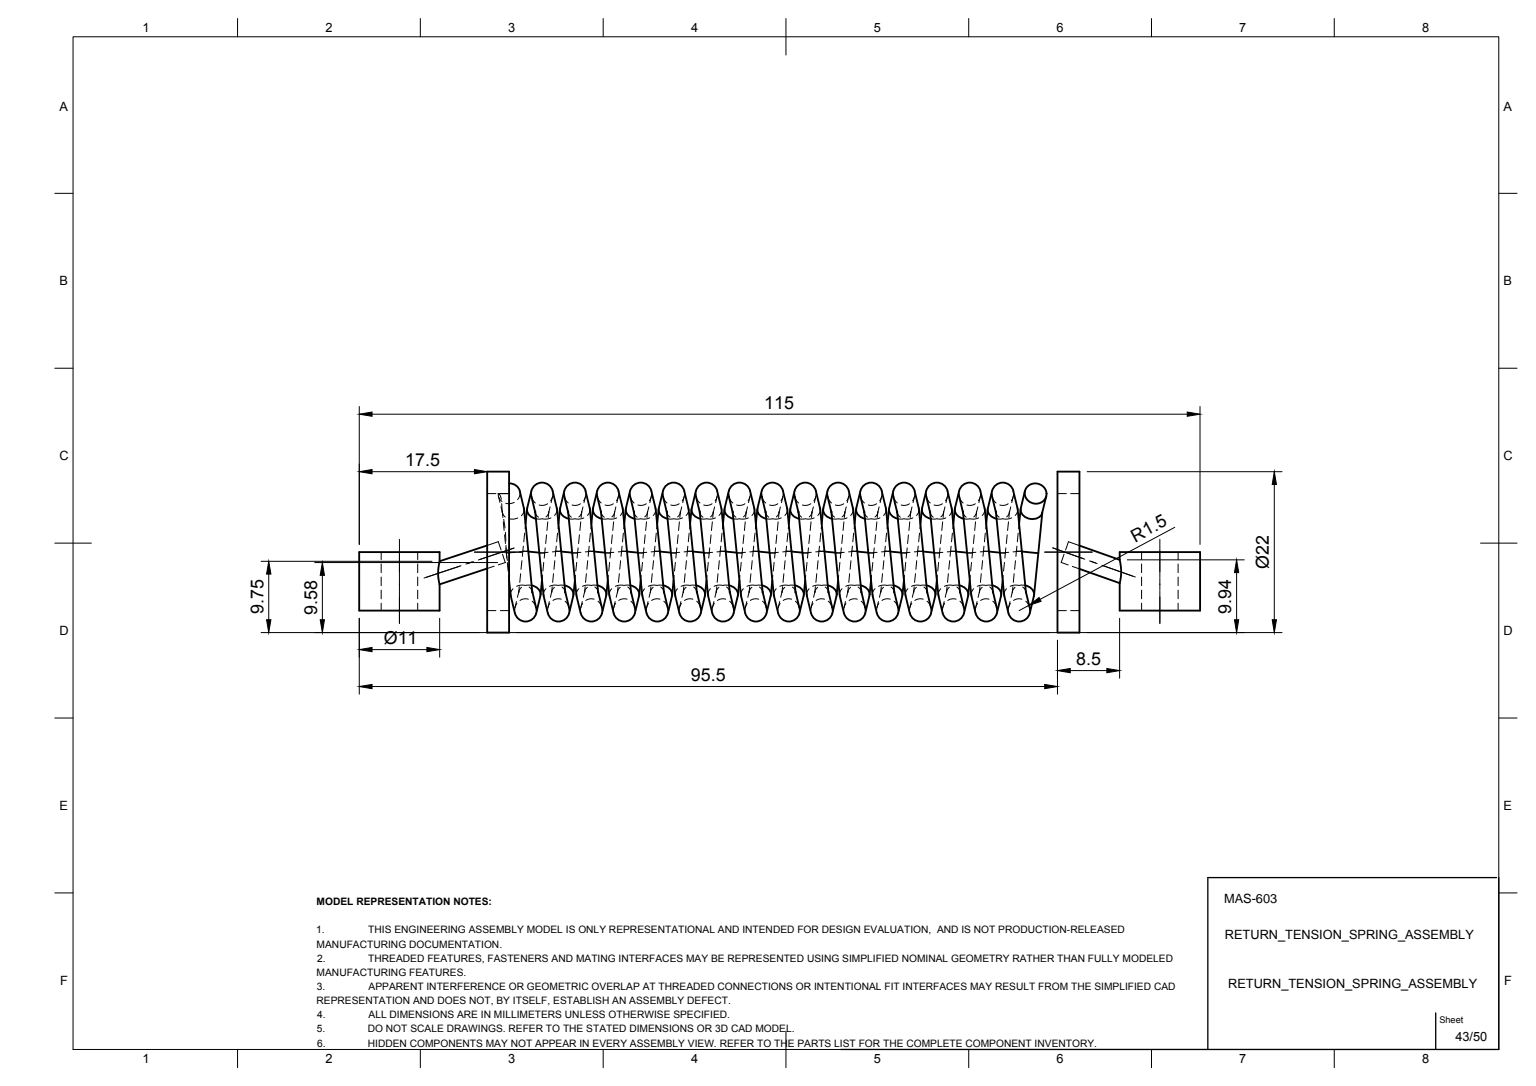
ISO-10303-21;
HEADER;
FILE_DESCRIPTION((''),'2;1');
FILE_NAME('RETURN_TENSION_SPRING_ASSEMBLY.step','2026-10-01T22:06:14-07:00',(''),(''),'','','');
FILE_SCHEMA (('AUTOMOTIVE_DESIGN { 1 0 10303 214 3 1 1 }'));
ENDSEC;
DATA;
#10=MECHANICAL_DESIGN_GEOMETRIC_PRESENTATION_REPRESENTATION('',(#1017,#1018,#1019,#1020),#50440);
#28=B_SPLINE_CURVE_WITH_KNOTS('',3,(#47529,#47530,#47531,#47532,#47533,
#47534,#47535,#47536,#47537,#47538),.UNSPECIFIED.,.F.,.F.,(4,2,2,2,4),(0.,
0.0609860967122279,0.121972193424456,0.180509993590844,0.239047793757233),
 .UNSPECIFIED.) ;
#29=B_SPLINE_CURVE_WITH_KNOTS('',3,(#47539,#47540,#47541,#47542,#47543,
#47544,#47545,#47546,#47547,#47548,#47549,#47550,#47551,#47552,#47553,#47554,
#47555,#47556,#47557,#47558,#47559,#47560,#47561,#47562,#47563,#47564),
 .UNSPECIFIED.,.F.,.F.,(4,2,2,2,2,2,2,2,2,2,2,2,4),(0.239047793757233,0.297585593923622,
0.35612339409001,0.417109490802238,0.478095587514466,0.536342851072485,
0.594590114630504,0.651016946753083,0.707443778875663,0.763870610998243,
0.820297443120823,0.878544706678841,0.93679197023686),.UNSPECIFIED.) ;
#30=B_SPLINE_CURVE_WITH_KNOTS('',3,(#47597,#47598,#47599,#47600,#47601,
#47602,#47603,#47604,#47605,#47606),.UNSPECIFIED.,.F.,.F.,(4,2,2,2,4),(1.59601342827562,
1.72868455666642,1.90688135822923,2.08609099459942,2.19153831493185),
 .UNSPECIFIED.) ;
#31=B_SPLINE_CURVE_WITH_KNOTS('',3,(#47608,#47609,#47610,#47611,#47612,
#47613,#47614,#47615,#47616,#47617),.UNSPECIFIED.,.F.,.F.,(4,2,2,2,4),(1.59601342827561,
1.72868455666641,1.90688135822922,2.0860909945994,2.19148469566779),
 .UNSPECIFIED.) ;
#32=B_SPLINE_CURVE_WITH_KNOTS('',3,(#47619,#47620,#47621,#47622,#47623,
#47624),.UNSPECIFIED.,.F.,.F.,(4,2,4),(1.93627902173741,2.08609099459941,
2.19148469566782),.UNSPECIFIED.) ;
#33=B_SPLINE_CURVE_WITH_KNOTS('',3,(#49299,#49300,#49301,#49302,#49303,
#49304,#49305,#49306,#49307,#49308,#49309,#49310,#49311,#49312,#49313,#49314,
#49315,#49316),.UNSPECIFIED.,.F.,.F.,(4,2,2,2,2,2,2,2,4),(0.228893413219578,
0.285350813018225,0.341808212816873,0.399797519628014,0.457786826439155,
0.518403668051846,0.579020509664538,0.637418929805441,0.695817349946344),
 .UNSPECIFIED.) ;
#34=B_SPLINE_CURVE_WITH_KNOTS('',3,(#49321,#49322,#49323,#49324,#49325,
#49326,#49327,#49328,#49329,#49330),.UNSPECIFIED.,.F.,.F.,(4,2,2,2,4),(0.,
0.0579893068111412,0.115978613622282,0.17243601342093,0.228893413219578),
 .UNSPECIFIED.) ;
#35=B_SPLINE_CURVE_WITH_KNOTS('',3,(#49331,#49332,#49333,#49334,#49335,
#49336,#49337,#49338,#49339,#49340),.UNSPECIFIED.,.F.,.F.,(4,2,2,2,4),(0.695817349946344,
0.754215770087248,0.812614190228152,0.873231031840842,0.933847873453534),
 .UNSPECIFIED.) ;
#417=ELLIPSE('',#31090,8.74484398085574,0.8) ;
#418=ELLIPSE('',#31097,1.63965824641058,0.15) ;
#419=ELLIPSE('',#31099,1.63965824641055,0.15) ;
#420=ELLIPSE('',#31101,1.63965824641045,0.15) ;
#421=ELLIPSE('',#31675,0.162242389830004,0.15) ;
#422=ELLIPSE('',#31677,0.162242389830007,0.15) ;
#423=ELLIPSE('',#31679,0.162242389830008,0.15) ;
#424=ELLIPSE('',#31680,0.162242389830008,0.15) ;
#425=ELLIPSE('',#31682,0.16224238983001,0.15) ;
#426=ELLIPSE('',#31683,0.16224238983001,0.15) ;
#427=ELLIPSE('',#31685,0.162242389830005,0.15) ;
#428=ELLIPSE('',#31686,0.162242389830005,0.15) ;
#429=ELLIPSE('',#31688,0.162242389830007,0.15) ;
#430=ELLIPSE('',#31689,0.162242389830007,0.15) ;
#431=ELLIPSE('',#31691,0.162242389830009,0.15) ;
#432=ELLIPSE('',#31692,0.162242389830009,0.15) ;
#433=ELLIPSE('',#31694,0.162242389830009,0.15) ;
#434=ELLIPSE('',#31695,0.162242389830009,0.15) ;
#435=ELLIPSE('',#31697,0.162242389830006,0.15) ;
#436=ELLIPSE('',#31698,0.162242389830006,0.15) ;
#437=ELLIPSE('',#31700,0.16224238983001,0.15) ;
#438=ELLIPSE('',#31701,0.16224238983001,0.15) ;
#439=ELLIPSE('',#31703,0.162242389830006,0.15) ;
#440=ELLIPSE('',#31704,0.162242389830006,0.15) ;
#441=ELLIPSE('',#31706,0.162242389830011,0.15) ;
#442=ELLIPSE('',#31707,0.162242389830011,0.15) ;
#443=ELLIPSE('',#31709,0.162242389830005,0.15) ;
#444=ELLIPSE('',#31710,0.162242389830005,0.15) ;
#445=ELLIPSE('',#31712,0.162242389830007,0.15) ;
#446=ELLIPSE('',#31713,0.162242389830007,0.15) ;
#447=ELLIPSE('',#31715,0.162242389830006,0.15) ;
#448=ELLIPSE('',#31716,0.162242389830006,0.15) ;
#449=ELLIPSE('',#31718,0.162242389830011,0.15) ;
#450=ELLIPSE('',#31719,0.162242389830011,0.15) ;
#451=ELLIPSE('',#31721,0.162242389830004,0.15) ;
#452=ELLIPSE('',#31722,0.162242389830004,0.15) ;
#453=ELLIPSE('',#31724,0.162242389830007,0.15) ;
#454=ELLIPSE('',#31725,0.162242389830007,0.15) ;
#455=ELLIPSE('',#31727,0.162242389830008,0.15) ;
#456=ELLIPSE('',#31728,0.162242389830008,0.15) ;
#457=ELLIPSE('',#31730,0.162242389830011,0.15) ;
#458=ELLIPSE('',#31731,0.162242389830011,0.15) ;
#459=ELLIPSE('',#31733,0.162242389830005,0.15) ;
#460=ELLIPSE('',#31734,0.162242389830005,0.15) ;
#461=ELLIPSE('',#31736,0.162242389830007,0.15) ;
#462=ELLIPSE('',#31737,0.162242389830007,0.15) ;
#463=ELLIPSE('',#31739,0.162242389830008,0.15) ;
#464=ELLIPSE('',#31740,0.162242389830008,0.15) ;
#465=ELLIPSE('',#31742,0.162242389830008,0.15) ;
#466=ELLIPSE('',#31743,0.162242389830008,0.15) ;
#467=ELLIPSE('',#31745,0.162242389830006,0.15) ;
#468=ELLIPSE('',#31746,0.162242389830006,0.15) ;
#469=ELLIPSE('',#31748,0.16224238983001,0.15) ;
#470=ELLIPSE('',#31749,0.16224238983001,0.15) ;
#471=ELLIPSE('',#31751,0.162242389830006,0.15) ;
#472=ELLIPSE('',#31752,0.162242389830006,0.15) ;
#473=ELLIPSE('',#31754,0.16224238983001,0.15) ;
#474=ELLIPSE('',#31755,0.16224238983001,0.15) ;
#475=ELLIPSE('',#31757,0.162242389830005,0.15) ;
#476=ELLIPSE('',#31758,0.162242389830005,0.15) ;
#477=ELLIPSE('',#31760,0.16224238983001,0.15) ;
#478=ELLIPSE('',#31761,0.16224238983001,0.15) ;
#479=ELLIPSE('',#31763,0.162242389830006,0.15) ;
#480=ELLIPSE('',#31764,0.162242389830006,0.15) ;
#481=ELLIPSE('',#31766,0.162242389830011,0.15) ;
#482=ELLIPSE('',#31767,0.162242389830011,0.15) ;
#483=ELLIPSE('',#31769,0.162242389830004,0.15) ;
#484=ELLIPSE('',#31770,0.162242389830004,0.15) ;
#485=ELLIPSE('',#31772,0.162242389830007,0.15) ;
#486=ELLIPSE('',#31773,0.162242389830007,0.15) ;
#487=ELLIPSE('',#31775,0.162242389830008,0.15) ;
#488=ELLIPSE('',#31776,0.162242389830008,0.15) ;
#489=ELLIPSE('',#31778,0.16224238983001,0.15) ;
#490=ELLIPSE('',#31779,0.16224238983001,0.15) ;
#491=ELLIPSE('',#31781,0.162242389830005,0.15) ;
#492=ELLIPSE('',#31782,0.162242389830005,0.15) ;
#493=ELLIPSE('',#31784,0.162242389830007,0.15) ;
#494=ELLIPSE('',#31785,0.162242389830007,0.15) ;
#495=ELLIPSE('',#31787,0.162242389830009,0.15) ;
#496=ELLIPSE('',#31788,0.162242389830009,0.15) ;
#497=ELLIPSE('',#31790,0.162242389830008,0.15) ;
#498=ELLIPSE('',#31791,0.162242389830008,0.15) ;
#499=ELLIPSE('',#31793,0.162242389830006,0.15) ;
#500=ELLIPSE('',#31794,0.162242389830006,0.15) ;
#501=ELLIPSE('',#31796,0.16224238983001,0.15) ;
#502=ELLIPSE('',#31797,0.16224238983001,0.15) ;
#503=ELLIPSE('',#31799,0.162242389830006,0.15) ;
#504=ELLIPSE('',#31800,0.162242389830006,0.15) ;
#505=ELLIPSE('',#31802,0.16224238983001,0.15) ;
#506=ELLIPSE('',#31803,0.16224238983001,0.15) ;
#507=ELLIPSE('',#31805,0.162242389830005,0.15) ;
#508=ELLIPSE('',#31806,0.162242389830005,0.15) ;
#509=ELLIPSE('',#31808,0.16224238983001,0.15) ;
#510=ELLIPSE('',#31809,0.16224238983001,0.15) ;
#511=ELLIPSE('',#31811,0.162242389830006,0.15) ;
#512=ELLIPSE('',#31812,0.162242389830006,0.15) ;
#513=ELLIPSE('',#31814,0.162242389830011,0.15) ;
#514=ELLIPSE('',#31815,0.162242389830011,0.15) ;
#515=ELLIPSE('',#31817,0.162242389830006,0.15) ;
#516=ELLIPSE('',#31818,0.162242389830006,0.15) ;
#517=ELLIPSE('',#31820,0.16224238983001,0.15) ;
#518=ELLIPSE('',#31821,0.16224238983001,0.15) ;
#519=ELLIPSE('',#31823,0.162242389830006,0.15) ;
#520=ELLIPSE('',#31824,0.162242389830006,0.15) ;
#521=ELLIPSE('',#31826,0.162242389830011,0.15) ;
#522=ELLIPSE('',#31827,0.162242389830011,0.15) ;
#523=ELLIPSE('',#31829,0.162242389830005,0.15) ;
#524=ELLIPSE('',#31830,0.162242389830005,0.15) ;
#525=ELLIPSE('',#31832,0.162242389830007,0.15) ;
#526=ELLIPSE('',#31833,0.162242389830007,0.15) ;
#527=ELLIPSE('',#31835,0.162242389830006,0.15) ;
#528=ELLIPSE('',#31836,0.162242389830006,0.15) ;
#529=ELLIPSE('',#31838,0.162242389830011,0.15) ;
#530=ELLIPSE('',#31839,0.162242389830011,0.15) ;
#531=ELLIPSE('',#31841,0.162242389830006,0.15) ;
#532=ELLIPSE('',#31842,0.162242389830006,0.15) ;
#533=ELLIPSE('',#31844,0.16224238983001,0.15) ;
#534=ELLIPSE('',#31845,0.16224238983001,0.15) ;
#535=ELLIPSE('',#31847,0.162242389830006,0.15) ;
#536=ELLIPSE('',#31848,0.162242389830006,0.15) ;
#537=ELLIPSE('',#31850,0.162242389830011,0.15) ;
#538=ELLIPSE('',#31851,0.162242389830011,0.15) ;
#539=ELLIPSE('',#31853,0.162242389830005,0.15) ;
#540=ELLIPSE('',#31854,0.162242389830005,0.15) ;
#541=ELLIPSE('',#31856,0.162242389830007,0.15) ;
#542=ELLIPSE('',#31857,0.162242389830007,0.15) ;
#543=ELLIPSE('',#31859,0.162242389830006,0.15) ;
#544=ELLIPSE('',#31860,0.162242389830006,0.15) ;
#545=ELLIPSE('',#31862,0.162242389830011,0.15) ;
#546=ELLIPSE('',#31863,0.162242389830011,0.15) ;
#547=ELLIPSE('',#31865,0.162242389830006,0.15) ;
#548=ELLIPSE('',#31866,0.162242389830006,0.15) ;
#549=ELLIPSE('',#31868,0.16224238983001,0.15) ;
#550=ELLIPSE('',#31869,0.16224238983001,0.15) ;
#551=ELLIPSE('',#31871,0.162242389830006,0.15) ;
#552=ELLIPSE('',#31872,0.162242389830006,0.15) ;
#553=ELLIPSE('',#31874,0.162242389830011,0.15) ;
#554=ELLIPSE('',#31875,0.162242389830011,0.15) ;
#555=ELLIPSE('',#31877,0.162242389830005,0.15) ;
#556=ELLIPSE('',#31878,0.162242389830005,0.15) ;
#557=ELLIPSE('',#31880,0.162242389830007,0.15) ;
#558=ELLIPSE('',#31881,0.162242389830007,0.15) ;
#559=ELLIPSE('',#31883,0.162242389830006,0.15) ;
#560=ELLIPSE('',#31884,0.162242389830006,0.15) ;
#561=ELLIPSE('',#31886,0.162242389830011,0.15) ;
#562=ELLIPSE('',#31887,0.162242389830011,0.15) ;
#563=ELLIPSE('',#31889,0.162242389830004,0.15) ;
#564=ELLIPSE('',#31890,0.162242389830004,0.15) ;
#565=ELLIPSE('',#31892,0.162242389830007,0.15) ;
#566=ELLIPSE('',#31893,0.162242389830007,0.15) ;
#567=ELLIPSE('',#31895,0.162242389830006,0.15) ;
#568=ELLIPSE('',#31896,0.162242389830006,0.15) ;
#569=ELLIPSE('',#31898,0.16224238983001,0.15) ;
#570=ELLIPSE('',#31899,0.16224238983001,0.15) ;
#571=ELLIPSE('',#31901,0.162242389830005,0.15) ;
#572=ELLIPSE('',#31902,0.162242389830005,0.15) ;
#573=ELLIPSE('',#31904,0.162242389830007,0.15) ;
#574=ELLIPSE('',#31905,0.162242389830007,0.15) ;
#575=ELLIPSE('',#31907,0.162242389830006,0.15) ;
#576=ELLIPSE('',#31908,0.162242389830006,0.15) ;
#577=ELLIPSE('',#31910,0.162242389830011,0.15) ;
#578=ELLIPSE('',#31911,0.162242389830011,0.15) ;
#579=ELLIPSE('',#31913,0.162242389830004,0.15) ;
#580=ELLIPSE('',#31914,0.162242389830004,0.15) ;
#581=ELLIPSE('',#31916,0.162242389830007,0.15) ;
#582=ELLIPSE('',#31917,0.162242389830007,0.15) ;
#583=ELLIPSE('',#31919,0.162242389830006,0.15) ;
#584=ELLIPSE('',#31920,0.162242389830006,0.15) ;
#585=ELLIPSE('',#31922,0.16224238983001,0.15) ;
#586=ELLIPSE('',#31923,0.16224238983001,0.15) ;
#587=ELLIPSE('',#31925,0.162242389830005,0.15) ;
#588=ELLIPSE('',#31926,0.162242389830005,0.15) ;
#589=ELLIPSE('',#31928,0.162242389830007,0.15) ;
#590=ELLIPSE('',#31929,0.162242389830007,0.15) ;
#591=ELLIPSE('',#31931,0.162242389830006,0.15) ;
#592=ELLIPSE('',#31932,0.162242389830006,0.15) ;
#593=ELLIPSE('',#31934,0.162242389830011,0.15) ;
#594=ELLIPSE('',#31935,0.162242389830011,0.15) ;
#595=ELLIPSE('',#31937,0.162242389830004,0.15) ;
#596=ELLIPSE('',#31938,0.162242389830004,0.15) ;
#597=ELLIPSE('',#31940,0.162242389830007,0.15) ;
#598=ELLIPSE('',#31941,0.162242389830007,0.15) ;
#599=ELLIPSE('',#31943,0.162242389830006,0.15) ;
#600=ELLIPSE('',#31944,0.162242389830006,0.15) ;
#601=ELLIPSE('',#31946,0.162242389830011,0.15) ;
#602=ELLIPSE('',#31947,0.162242389830011,0.15) ;
#603=ELLIPSE('',#31949,0.162242389830005,0.15) ;
#604=ELLIPSE('',#31950,0.162242389830005,0.15) ;
#605=ELLIPSE('',#31952,0.162242389830007,0.15) ;
#606=ELLIPSE('',#31953,0.162242389830007,0.15) ;
#607=ELLIPSE('',#31955,0.162242389830008,0.15) ;
#608=ELLIPSE('',#31956,0.162242389830008,0.15) ;
#609=ELLIPSE('',#31958,0.162242389830011,0.15) ;
#610=ELLIPSE('',#31959,0.162242389830011,0.15) ;
#611=ELLIPSE('',#31961,0.162242389830004,0.15) ;
#612=ELLIPSE('',#31962,0.162242389830004,0.15) ;
#613=ELLIPSE('',#31964,0.162242389830007,0.15) ;
#614=ELLIPSE('',#31965,0.162242389830007,0.15) ;
#615=ELLIPSE('',#31967,0.162242389830006,0.15) ;
#616=ELLIPSE('',#31968,0.162242389830006,0.15) ;
#617=ELLIPSE('',#31970,0.16224238983001,0.15) ;
#618=ELLIPSE('',#31971,0.16224238983001,0.15) ;
#619=ELLIPSE('',#31973,0.162242389830005,0.15) ;
#620=ELLIPSE('',#31974,0.162242389830005,0.15) ;
#621=ELLIPSE('',#31976,0.162242389830007,0.15) ;
#622=ELLIPSE('',#31977,0.162242389830007,0.15) ;
#623=ELLIPSE('',#31979,0.162242389830008,0.15) ;
#624=ELLIPSE('',#31980,0.162242389830008,0.15) ;
#625=ELLIPSE('',#31982,0.162242389830011,0.15) ;
#626=ELLIPSE('',#31983,0.162242389830011,0.15) ;
#627=ELLIPSE('',#31985,0.162242389830004,0.15) ;
#628=ELLIPSE('',#31986,0.162242389830004,0.15) ;
#629=ELLIPSE('',#31988,0.162242389830007,0.15) ;
#630=ELLIPSE('',#31989,0.162242389830007,0.15) ;
#631=ELLIPSE('',#31991,0.162242389830006,0.15) ;
#632=ELLIPSE('',#31992,0.162242389830006,0.15) ;
#633=ELLIPSE('',#31994,0.162242389830011,0.15) ;
#634=ELLIPSE('',#31995,0.162242389830011,0.15) ;
#635=ELLIPSE('',#31997,0.162242389830005,0.15) ;
#636=ELLIPSE('',#31998,0.162242389830005,0.15) ;
#637=ELLIPSE('',#32000,0.162242389830007,0.15) ;
#638=ELLIPSE('',#32001,0.162242389830007,0.15) ;
#639=ELLIPSE('',#32003,0.162242389830008,0.15) ;
#640=ELLIPSE('',#32004,0.162242389830008,0.15) ;
#641=ELLIPSE('',#32006,0.162242389830011,0.15) ;
#642=ELLIPSE('',#32007,0.162242389830011,0.15) ;
#643=ELLIPSE('',#32009,0.162242389830004,0.15) ;
#644=ELLIPSE('',#32010,0.162242389830004,0.15) ;
#645=ELLIPSE('',#32012,0.162242389830007,0.15) ;
#646=ELLIPSE('',#32013,0.162242389830007,0.15) ;
#647=ELLIPSE('',#32015,0.162242389830006,0.15) ;
#648=ELLIPSE('',#32016,0.162242389830006,0.15) ;
#649=ELLIPSE('',#32018,0.16224238983001,0.15) ;
#650=ELLIPSE('',#32019,0.16224238983001,0.15) ;
#651=ELLIPSE('',#32021,0.162242389830005,0.15) ;
#652=ELLIPSE('',#32022,0.162242389830005,0.15) ;
#653=ELLIPSE('',#32024,0.162242389830007,0.15) ;
#654=ELLIPSE('',#32025,0.162242389830007,0.15) ;
#655=ELLIPSE('',#32027,0.162242389830008,0.15) ;
#656=ELLIPSE('',#32028,0.162242389830008,0.15) ;
#657=ELLIPSE('',#32030,0.162242389830012,0.15) ;
#658=ELLIPSE('',#32031,0.162242389830012,0.15) ;
#659=ELLIPSE('',#32033,0.162242389830004,0.15) ;
#660=ELLIPSE('',#32034,0.162242389830004,0.15) ;
#661=ELLIPSE('',#32036,0.162242389830007,0.15) ;
#662=ELLIPSE('',#32037,0.162242389830007,0.15) ;
#663=ELLIPSE('',#32039,0.162242389830006,0.15) ;
#664=ELLIPSE('',#32040,0.162242389830006,0.15) ;
#665=ELLIPSE('',#32042,0.162242389830011,0.15) ;
#666=ELLIPSE('',#32043,0.162242389830011,0.15) ;
#667=ELLIPSE('',#32045,0.162242389830005,0.15) ;
#668=ELLIPSE('',#32046,0.162242389830005,0.15) ;
#669=ELLIPSE('',#32048,0.162242389830007,0.15) ;
#670=ELLIPSE('',#32049,0.162242389830007,0.15) ;
#671=ELLIPSE('',#32051,0.162242389830008,0.15) ;
#672=ELLIPSE('',#32052,0.162242389830008,0.15) ;
#748=SPHERICAL_SURFACE('',#31105,0.15) ;
#749=SPHERICAL_SURFACE('',#31108,0.15) ;
#750=SPHERICAL_SURFACE('',#31112,0.15) ;
#751=SPHERICAL_SURFACE('',#31116,0.15) ;
#752=SPHERICAL_SURFACE('',#31122,0.15) ;
#753=SPHERICAL_SURFACE('',#31126,0.15) ;
#754=SPHERICAL_SURFACE('',#31130,0.15) ;
#755=SPHERICAL_SURFACE('',#31134,0.15) ;
#756=SPHERICAL_SURFACE('',#31140,0.15) ;
#757=SPHERICAL_SURFACE('',#31144,0.15) ;
#758=SPHERICAL_SURFACE('',#31148,0.15) ;
#759=SPHERICAL_SURFACE('',#31152,0.15) ;
#760=SPHERICAL_SURFACE('',#31158,0.15) ;
#761=SPHERICAL_SURFACE('',#31162,0.15) ;
#762=SPHERICAL_SURFACE('',#31166,0.15) ;
#763=SPHERICAL_SURFACE('',#31170,0.15) ;
#764=SPHERICAL_SURFACE('',#31176,0.15) ;
#765=SPHERICAL_SURFACE('',#31180,0.15) ;
#766=SPHERICAL_SURFACE('',#31184,0.15) ;
#767=SPHERICAL_SURFACE('',#31188,0.15) ;
#768=SPHERICAL_SURFACE('',#31194,0.15) ;
#769=SPHERICAL_SURFACE('',#31198,0.15) ;
#770=SPHERICAL_SURFACE('',#31202,0.15) ;
#771=SPHERICAL_SURFACE('',#31206,0.15) ;
#772=SPHERICAL_SURFACE('',#31212,0.15) ;
#773=SPHERICAL_SURFACE('',#31216,0.15) ;
#774=SPHERICAL_SURFACE('',#31220,0.15) ;
#775=SPHERICAL_SURFACE('',#31224,0.15) ;
#776=SPHERICAL_SURFACE('',#31230,0.15) ;
#777=SPHERICAL_SURFACE('',#31234,0.15) ;
#778=SPHERICAL_SURFACE('',#31238,0.15) ;
#779=SPHERICAL_SURFACE('',#31242,0.15) ;
#780=SPHERICAL_SURFACE('',#31248,0.15) ;
#781=SPHERICAL_SURFACE('',#31252,0.15) ;
#782=SPHERICAL_SURFACE('',#31256,0.15) ;
#783=SPHERICAL_SURFACE('',#31260,0.15) ;
#784=SPHERICAL_SURFACE('',#31266,0.15) ;
#785=SPHERICAL_SURFACE('',#31270,0.15) ;
#786=SPHERICAL_SURFACE('',#31274,0.15) ;
#787=SPHERICAL_SURFACE('',#31278,0.15) ;
#788=SPHERICAL_SURFACE('',#31284,0.15) ;
#789=SPHERICAL_SURFACE('',#31288,0.15) ;
#790=SPHERICAL_SURFACE('',#31292,0.15) ;
#791=SPHERICAL_SURFACE('',#31296,0.15) ;
#792=SPHERICAL_SURFACE('',#31302,0.15) ;
#793=SPHERICAL_SURFACE('',#31306,0.15) ;
#794=SPHERICAL_SURFACE('',#31310,0.15) ;
#795=SPHERICAL_SURFACE('',#31314,0.15) ;
#796=SPHERICAL_SURFACE('',#31320,0.15) ;
#797=SPHERICAL_SURFACE('',#31324,0.15) ;
#798=SPHERICAL_SURFACE('',#31328,0.15) ;
#799=SPHERICAL_SURFACE('',#31332,0.15) ;
#800=SPHERICAL_SURFACE('',#31338,0.15) ;
#801=SPHERICAL_SURFACE('',#31342,0.15) ;
#802=SPHERICAL_SURFACE('',#31346,0.15) ;
#803=SPHERICAL_SURFACE('',#31350,0.15) ;
#804=SPHERICAL_SURFACE('',#31356,0.15) ;
#805=SPHERICAL_SURFACE('',#31360,0.15) ;
#806=SPHERICAL_SURFACE('',#31364,0.15) ;
#807=SPHERICAL_SURFACE('',#31368,0.15) ;
#808=SPHERICAL_SURFACE('',#31374,0.15) ;
#809=SPHERICAL_SURFACE('',#31378,0.15) ;
#810=SPHERICAL_SURFACE('',#31382,0.15) ;
#811=SPHERICAL_SURFACE('',#31386,0.15) ;
#812=SPHERICAL_SURFACE('',#31392,0.15) ;
#813=SPHERICAL_SURFACE('',#31396,0.15) ;
#814=SPHERICAL_SURFACE('',#31400,0.15) ;
#815=SPHERICAL_SURFACE('',#31404,0.15) ;
#816=SPHERICAL_SURFACE('',#31410,0.15) ;
#817=SPHERICAL_SURFACE('',#31414,0.15) ;
#818=SPHERICAL_SURFACE('',#31418,0.15) ;
#819=SPHERICAL_SURFACE('',#31422,0.15) ;
#820=SPHERICAL_SURFACE('',#31428,0.15) ;
#821=SPHERICAL_SURFACE('',#31432,0.15) ;
#822=SPHERICAL_SURFACE('',#31436,0.15) ;
#823=SPHERICAL_SURFACE('',#31440,0.15) ;
#824=SPHERICAL_SURFACE('',#31446,0.15) ;
#825=SPHERICAL_SURFACE('',#31450,0.15) ;
#826=SPHERICAL_SURFACE('',#31454,0.15) ;
#827=SPHERICAL_SURFACE('',#31458,0.15) ;
#828=SPHERICAL_SURFACE('',#31464,0.15) ;
#829=SPHERICAL_SURFACE('',#31468,0.15) ;
#830=SPHERICAL_SURFACE('',#31472,0.15) ;
#831=SPHERICAL_SURFACE('',#31476,0.15) ;
#832=SPHERICAL_SURFACE('',#31482,0.15) ;
#833=SPHERICAL_SURFACE('',#31486,0.15) ;
#834=SPHERICAL_SURFACE('',#31490,0.15) ;
#835=SPHERICAL_SURFACE('',#31494,0.15) ;
#836=SPHERICAL_SURFACE('',#31500,0.15) ;
#837=SPHERICAL_SURFACE('',#31504,0.15) ;
#838=SPHERICAL_SURFACE('',#31508,0.15) ;
#839=SPHERICAL_SURFACE('',#31512,0.15) ;
#840=SPHERICAL_SURFACE('',#31518,0.15) ;
#841=SPHERICAL_SURFACE('',#31522,0.15) ;
#842=SPHERICAL_SURFACE('',#31526,0.15) ;
#843=SPHERICAL_SURFACE('',#31530,0.15) ;
#844=SPHERICAL_SURFACE('',#31536,0.15) ;
#845=SPHERICAL_SURFACE('',#31540,0.15) ;
#846=SPHERICAL_SURFACE('',#31544,0.15) ;
#847=SPHERICAL_SURFACE('',#31548,0.15) ;
#848=SPHERICAL_SURFACE('',#31554,0.15) ;
#849=SPHERICAL_SURFACE('',#31558,0.15) ;
#850=SPHERICAL_SURFACE('',#31562,0.15) ;
#851=SPHERICAL_SURFACE('',#31566,0.15) ;
#852=SPHERICAL_SURFACE('',#31572,0.15) ;
#853=SPHERICAL_SURFACE('',#31576,0.15) ;
#854=SPHERICAL_SURFACE('',#31580,0.15) ;
#855=SPHERICAL_SURFACE('',#31584,0.15) ;
#856=SPHERICAL_SURFACE('',#31590,0.15) ;
#857=SPHERICAL_SURFACE('',#31594,0.15) ;
#858=SPHERICAL_SURFACE('',#31598,0.15) ;
#859=SPHERICAL_SURFACE('',#31602,0.15) ;
#860=SPHERICAL_SURFACE('',#31608,0.15) ;
#861=SPHERICAL_SURFACE('',#31612,0.15) ;
#862=SPHERICAL_SURFACE('',#31616,0.15) ;
#863=SPHERICAL_SURFACE('',#31620,0.15) ;
#864=SPHERICAL_SURFACE('',#31626,0.15) ;
#865=SPHERICAL_SURFACE('',#31630,0.15) ;
#866=SPHERICAL_SURFACE('',#31634,0.15) ;
#867=SPHERICAL_SURFACE('',#31638,0.15) ;
#868=SPHERICAL_SURFACE('',#31644,0.15) ;
#869=SPHERICAL_SURFACE('',#31648,0.15) ;
#870=SPHERICAL_SURFACE('',#31652,0.15) ;
#871=SPHERICAL_SURFACE('',#31656,0.15) ;
#872=SPHERICAL_SURFACE('',#31662,0.15) ;
#873=SPHERICAL_SURFACE('',#31666,0.15) ;
#874=SPHERICAL_SURFACE('',#31670,0.15) ;
#923=SHAPE_REPRESENTATION_RELATIONSHIP('SRR','None',#50656,#968) ;
#968=ADVANCED_BREP_SHAPE_REPRESENTATION('',(#1071,#1072,#1073,#1074),#50425) ;
#1017=STYLED_ITEM('',(#50883),#1071) ;
#1018=STYLED_ITEM('',(#50883),#1072) ;
#1019=STYLED_ITEM('',(#50883),#1073) ;
#1020=STYLED_ITEM('',(#50883),#1074) ;
#1071=MANIFOLD_SOLID_BREP('RETURN_TENSION_SPRING_ASSEMBLY',#28693) ;
#1072=MANIFOLD_SOLID_BREP('RETURN_TENSION_SPRING_ASSEMBLY',#28694) ;
#1073=MANIFOLD_SOLID_BREP('RETURN_TENSION_SPRING_ASSEMBLY',#28695) ;
#1074=MANIFOLD_SOLID_BREP('RETURN_TENSION_SPRING_ASSEMBLY',#28696) ;
#1379=FACE_BOUND('',#5297,.T.) ;
#1380=FACE_BOUND('',#5300,.T.) ;
#1381=FACE_BOUND('',#5302,.T.) ;
#1382=FACE_BOUND('',#5308,.T.) ;
#1383=FACE_BOUND('',#5310,.T.) ;
#1384=FACE_BOUND('',#5314,.T.) ;
#1385=FACE_BOUND('',#5316,.T.) ;
#1386=FACE_BOUND('',#5577,.T.) ;
#1387=FACE_BOUND('',#5579,.T.) ;
#2244=PLANE('',#31076) ;
#2245=PLANE('',#31077) ;
#2246=PLANE('',#31080) ;
#2247=PLANE('',#31087) ;
#2248=PLANE('',#31088) ;
#2249=PLANE('',#31096) ;
#2250=PLANE('',#31102) ;
#2251=PLANE('',#31103) ;
#2252=PLANE('',#32055) ;
#2253=PLANE('',#32062) ;
#2254=PLANE('',#32063) ;
#2255=PLANE('',#32066) ;
#3475=FACE_OUTER_BOUND('',#5296,.T.) ;
#3476=FACE_OUTER_BOUND('',#5298,.T.) ;
#3477=FACE_OUTER_BOUND('',#5299,.T.) ;
#3478=FACE_OUTER_BOUND('',#5301,.T.) ;
#3479=FACE_OUTER_BOUND('',#5303,.T.) ;
#3480=FACE_OUTER_BOUND('',#5304,.T.) ;
#3481=FACE_OUTER_BOUND('',#5305,.T.) ;
#3482=FACE_OUTER_BOUND('',#5306,.T.) ;
#3483=FACE_OUTER_BOUND('',#5307,.T.) ;
#3484=FACE_OUTER_BOUND('',#5309,.T.) ;
#3485=FACE_OUTER_BOUND('',#5311,.T.) ;
#3486=FACE_OUTER_BOUND('',#5312,.T.) ;
#3487=FACE_OUTER_BOUND('',#5313,.T.) ;
#3488=FACE_OUTER_BOUND('',#5315,.T.) ;
#3489=FACE_OUTER_BOUND('',#5317,.T.) ;
#3490=FACE_OUTER_BOUND('',#5318,.T.) ;
#3491=FACE_OUTER_BOUND('',#5319,.T.) ;
#3492=FACE_OUTER_BOUND('',#5320,.T.) ;
#3493=FACE_OUTER_BOUND('',#5321,.T.) ;
#3494=FACE_OUTER_BOUND('',#5322,.T.) ;
#3495=FACE_OUTER_BOUND('',#5323,.T.) ;
#3496=FACE_OUTER_BOUND('',#5324,.T.) ;
#3497=FACE_OUTER_BOUND('',#5325,.T.) ;
#3498=FACE_OUTER_BOUND('',#5326,.T.) ;
#3499=FACE_OUTER_BOUND('',#5327,.T.) ;
#3500=FACE_OUTER_BOUND('',#5328,.T.) ;
#3501=FACE_OUTER_BOUND('',#5329,.T.) ;
#3502=FACE_OUTER_BOUND('',#5330,.T.) ;
#3503=FACE_OUTER_BOUND('',#5331,.T.) ;
#3504=FACE_OUTER_BOUND('',#5332,.T.) ;
#3505=FACE_OUTER_BOUND('',#5333,.T.) ;
#3506=FACE_OUTER_BOUND('',#5334,.T.) ;
#3507=FACE_OUTER_BOUND('',#5335,.T.) ;
#3508=FACE_OUTER_BOUND('',#5336,.T.) ;
#3509=FACE_OUTER_BOUND('',#5337,.T.) ;
#3510=FACE_OUTER_BOUND('',#5338,.T.) ;
#3511=FACE_OUTER_BOUND('',#5339,.T.) ;
#3512=FACE_OUTER_BOUND('',#5340,.T.) ;
#3513=FACE_OUTER_BOUND('',#5341,.T.) ;
#3514=FACE_OUTER_BOUND('',#5342,.T.) ;
#3515=FACE_OUTER_BOUND('',#5343,.T.) ;
#3516=FACE_OUTER_BOUND('',#5344,.T.) ;
#3517=FACE_OUTER_BOUND('',#5345,.T.) ;
#3518=FACE_OUTER_BOUND('',#5346,.T.) ;
#3519=FACE_OUTER_BOUND('',#5347,.T.) ;
#3520=FACE_OUTER_BOUND('',#5348,.T.) ;
#3521=FACE_OUTER_BOUND('',#5349,.T.) ;
#3522=FACE_OUTER_BOUND('',#5350,.T.) ;
#3523=FACE_OUTER_BOUND('',#5351,.T.) ;
#3524=FACE_OUTER_BOUND('',#5352,.T.) ;
#3525=FACE_OUTER_BOUND('',#5353,.T.) ;
#3526=FACE_OUTER_BOUND('',#5354,.T.) ;
#3527=FACE_OUTER_BOUND('',#5355,.T.) ;
#3528=FACE_OUTER_BOUND('',#5356,.T.) ;
#3529=FACE_OUTER_BOUND('',#5357,.T.) ;
#3530=FACE_OUTER_BOUND('',#5358,.T.) ;
#3531=FACE_OUTER_BOUND('',#5359,.T.) ;
#3532=FACE_OUTER_BOUND('',#5360,.T.) ;
#3533=FACE_OUTER_BOUND('',#5361,.T.) ;
#3534=FACE_OUTER_BOUND('',#5362,.T.) ;
#3535=FACE_OUTER_BOUND('',#5363,.T.) ;
#3536=FACE_OUTER_BOUND('',#5364,.T.) ;
#3537=FACE_OUTER_BOUND('',#5365,.T.) ;
#3538=FACE_OUTER_BOUND('',#5366,.T.) ;
#3539=FACE_OUTER_BOUND('',#5367,.T.) ;
#3540=FACE_OUTER_BOUND('',#5368,.T.) ;
#3541=FACE_OUTER_BOUND('',#5369,.T.) ;
#3542=FACE_OUTER_BOUND('',#5370,.T.) ;
#3543=FACE_OUTER_BOUND('',#5371,.T.) ;
#3544=FACE_OUTER_BOUND('',#5372,.T.) ;
#3545=FACE_OUTER_BOUND('',#5373,.T.) ;
#3546=FACE_OUTER_BOUND('',#5374,.T.) ;
#3547=FACE_OUTER_BOUND('',#5375,.T.) ;
#3548=FACE_OUTER_BOUND('',#5376,.T.) ;
#3549=FACE_OUTER_BOUND('',#5377,.T.) ;
#3550=FACE_OUTER_BOUND('',#5378,.T.) ;
#3551=FACE_OUTER_BOUND('',#5379,.T.) ;
#3552=FACE_OUTER_BOUND('',#5380,.T.) ;
#3553=FACE_OUTER_BOUND('',#5381,.T.) ;
#3554=FACE_OUTER_BOUND('',#5382,.T.) ;
#3555=FACE_OUTER_BOUND('',#5383,.T.) ;
#3556=FACE_OUTER_BOUND('',#5384,.T.) ;
#3557=FACE_OUTER_BOUND('',#5385,.T.) ;
#3558=FACE_OUTER_BOUND('',#5386,.T.) ;
#3559=FACE_OUTER_BOUND('',#5387,.T.) ;
#3560=FACE_OUTER_BOUND('',#5388,.T.) ;
#3561=FACE_OUTER_BOUND('',#5389,.T.) ;
#3562=FACE_OUTER_BOUND('',#5390,.T.) ;
#3563=FACE_OUTER_BOUND('',#5391,.T.) ;
#3564=FACE_OUTER_BOUND('',#5392,.T.) ;
#3565=FACE_OUTER_BOUND('',#5393,.T.) ;
#3566=FACE_OUTER_BOUND('',#5394,.T.) ;
#3567=FACE_OUTER_BOUND('',#5395,.T.) ;
#3568=FACE_OUTER_BOUND('',#5396,.T.) ;
#3569=FACE_OUTER_BOUND('',#5397,.T.) ;
#3570=FACE_OUTER_BOUND('',#5398,.T.) ;
#3571=FACE_OUTER_BOUND('',#5399,.T.) ;
#3572=FACE_OUTER_BOUND('',#5400,.T.) ;
#3573=FACE_OUTER_BOUND('',#5401,.T.) ;
#3574=FACE_OUTER_BOUND('',#5402,.T.) ;
#3575=FACE_OUTER_BOUND('',#5403,.T.) ;
#3576=FACE_OUTER_BOUND('',#5404,.T.) ;
#3577=FACE_OUTER_BOUND('',#5405,.T.) ;
#3578=FACE_OUTER_BOUND('',#5406,.T.) ;
#3579=FACE_OUTER_BOUND('',#5407,.T.) ;
#3580=FACE_OUTER_BOUND('',#5408,.T.) ;
#3581=FACE_OUTER_BOUND('',#5409,.T.) ;
#3582=FACE_OUTER_BOUND('',#5410,.T.) ;
#3583=FACE_OUTER_BOUND('',#5411,.T.) ;
#3584=FACE_OUTER_BOUND('',#5412,.T.) ;
#3585=FACE_OUTER_BOUND('',#5413,.T.) ;
#3586=FACE_OUTER_BOUND('',#5414,.T.) ;
#3587=FACE_OUTER_BOUND('',#5415,.T.) ;
#3588=FACE_OUTER_BOUND('',#5416,.T.) ;
#3589=FACE_OUTER_BOUND('',#5417,.T.) ;
#3590=FACE_OUTER_BOUND('',#5418,.T.) ;
#3591=FACE_OUTER_BOUND('',#5419,.T.) ;
#3592=FACE_OUTER_BOUND('',#5420,.T.) ;
#3593=FACE_OUTER_BOUND('',#5421,.T.) ;
#3594=FACE_OUTER_BOUND('',#5422,.T.) ;
#3595=FACE_OUTER_BOUND('',#5423,.T.) ;
#3596=FACE_OUTER_BOUND('',#5424,.T.) ;
#3597=FACE_OUTER_BOUND('',#5425,.T.) ;
#3598=FACE_OUTER_BOUND('',#5426,.T.) ;
#3599=FACE_OUTER_BOUND('',#5427,.T.) ;
#3600=FACE_OUTER_BOUND('',#5428,.T.) ;
#3601=FACE_OUTER_BOUND('',#5429,.T.) ;
#3602=FACE_OUTER_BOUND('',#5430,.T.) ;
#3603=FACE_OUTER_BOUND('',#5431,.T.) ;
#3604=FACE_OUTER_BOUND('',#5432,.T.) ;
#3605=FACE_OUTER_BOUND('',#5433,.T.) ;
#3606=FACE_OUTER_BOUND('',#5434,.T.) ;
#3607=FACE_OUTER_BOUND('',#5435,.T.) ;
#3608=FACE_OUTER_BOUND('',#5436,.T.) ;
#3609=FACE_OUTER_BOUND('',#5437,.T.) ;
#3610=FACE_OUTER_BOUND('',#5438,.T.) ;
#3611=FACE_OUTER_BOUND('',#5439,.T.) ;
#3612=FACE_OUTER_BOUND('',#5440,.T.) ;
#3613=FACE_OUTER_BOUND('',#5441,.T.) ;
#3614=FACE_OUTER_BOUND('',#5442,.T.) ;
#3615=FACE_OUTER_BOUND('',#5443,.T.) ;
#3616=FACE_OUTER_BOUND('',#5444,.T.) ;
#3617=FACE_OUTER_BOUND('',#5445,.T.) ;
#3618=FACE_OUTER_BOUND('',#5446,.T.) ;
#3619=FACE_OUTER_BOUND('',#5447,.T.) ;
#3620=FACE_OUTER_BOUND('',#5448,.T.) ;
#3621=FACE_OUTER_BOUND('',#5449,.T.) ;
#3622=FACE_OUTER_BOUND('',#5450,.T.) ;
#3623=FACE_OUTER_BOUND('',#5451,.T.) ;
#3624=FACE_OUTER_BOUND('',#5452,.T.) ;
#3625=FACE_OUTER_BOUND('',#5453,.T.) ;
#3626=FACE_OUTER_BOUND('',#5454,.T.) ;
#3627=FACE_OUTER_BOUND('',#5455,.T.) ;
#3628=FACE_OUTER_BOUND('',#5456,.T.) ;
#3629=FACE_OUTER_BOUND('',#5457,.T.) ;
#3630=FACE_OUTER_BOUND('',#5458,.T.) ;
#3631=FACE_OUTER_BOUND('',#5459,.T.) ;
#3632=FACE_OUTER_BOUND('',#5460,.T.) ;
#3633=FACE_OUTER_BOUND('',#5461,.T.) ;
#3634=FACE_OUTER_BOUND('',#5462,.T.) ;
#3635=FACE_OUTER_BOUND('',#5463,.T.) ;
#3636=FACE_OUTER_BOUND('',#5464,.T.) ;
#3637=FACE_OUTER_BOUND('',#5465,.T.) ;
#3638=FACE_OUTER_BOUND('',#5466,.T.) ;
#3639=FACE_OUTER_BOUND('',#5467,.T.) ;
#3640=FACE_OUTER_BOUND('',#5468,.T.) ;
#3641=FACE_OUTER_BOUND('',#5469,.T.) ;
#3642=FACE_OUTER_BOUND('',#5470,.T.) ;
#3643=FACE_OUTER_BOUND('',#5471,.T.) ;
#3644=FACE_OUTER_BOUND('',#5472,.T.) ;
#3645=FACE_OUTER_BOUND('',#5473,.T.) ;
#3646=FACE_OUTER_BOUND('',#5474,.T.) ;
#3647=FACE_OUTER_BOUND('',#5475,.T.) ;
#3648=FACE_OUTER_BOUND('',#5476,.T.) ;
#3649=FACE_OUTER_BOUND('',#5477,.T.) ;
#3650=FACE_OUTER_BOUND('',#5478,.T.) ;
#3651=FACE_OUTER_BOUND('',#5479,.T.) ;
#3652=FACE_OUTER_BOUND('',#5480,.T.) ;
#3653=FACE_OUTER_BOUND('',#5481,.T.) ;
#3654=FACE_OUTER_BOUND('',#5482,.T.) ;
#3655=FACE_OUTER_BOUND('',#5483,.T.) ;
#3656=FACE_OUTER_BOUND('',#5484,.T.) ;
#3657=FACE_OUTER_BOUND('',#5485,.T.) ;
#3658=FACE_OUTER_BOUND('',#5486,.T.) ;
#3659=FACE_OUTER_BOUND('',#5487,.T.) ;
#3660=FACE_OUTER_BOUND('',#5488,.T.) ;
#3661=FACE_OUTER_BOUND('',#5489,.T.) ;
#3662=FACE_OUTER_BOUND('',#5490,.T.) ;
#3663=FACE_OUTER_BOUND('',#5491,.T.) ;
#3664=FACE_OUTER_BOUND('',#5492,.T.) ;
#3665=FACE_OUTER_BOUND('',#5493,.T.) ;
#3666=FACE_OUTER_BOUND('',#5494,.T.) ;
#3667=FACE_OUTER_BOUND('',#5495,.T.) ;
#3668=FACE_OUTER_BOUND('',#5496,.T.) ;
#3669=FACE_OUTER_BOUND('',#5497,.T.) ;
#3670=FACE_OUTER_BOUND('',#5498,.T.) ;
#3671=FACE_OUTER_BOUND('',#5499,.T.) ;
#3672=FACE_OUTER_BOUND('',#5500,.T.) ;
#3673=FACE_OUTER_BOUND('',#5501,.T.) ;
#3674=FACE_OUTER_BOUND('',#5502,.T.) ;
#3675=FACE_OUTER_BOUND('',#5503,.T.) ;
#3676=FACE_OUTER_BOUND('',#5504,.T.) ;
#3677=FACE_OUTER_BOUND('',#5505,.T.) ;
#3678=FACE_OUTER_BOUND('',#5506,.T.) ;
#3679=FACE_OUTER_BOUND('',#5507,.T.) ;
#3680=FACE_OUTER_BOUND('',#5508,.T.) ;
#3681=FACE_OUTER_BOUND('',#5509,.T.) ;
#3682=FACE_OUTER_BOUND('',#5510,.T.) ;
#3683=FACE_OUTER_BOUND('',#5511,.T.) ;
#3684=FACE_OUTER_BOUND('',#5512,.T.) ;
#3685=FACE_OUTER_BOUND('',#5513,.T.) ;
#3686=FACE_OUTER_BOUND('',#5514,.T.) ;
#3687=FACE_OUTER_BOUND('',#5515,.T.) ;
#3688=FACE_OUTER_BOUND('',#5516,.T.) ;
#3689=FACE_OUTER_BOUND('',#5517,.T.) ;
#3690=FACE_OUTER_BOUND('',#5518,.T.) ;
#3691=FACE_OUTER_BOUND('',#5519,.T.) ;
#3692=FACE_OUTER_BOUND('',#5520,.T.) ;
#3693=FACE_OUTER_BOUND('',#5521,.T.) ;
#3694=FACE_OUTER_BOUND('',#5522,.T.) ;
#3695=FACE_OUTER_BOUND('',#5523,.T.) ;
#3696=FACE_OUTER_BOUND('',#5524,.T.) ;
#3697=FACE_OUTER_BOUND('',#5525,.T.) ;
#3698=FACE_OUTER_BOUND('',#5526,.T.) ;
#3699=FACE_OUTER_BOUND('',#5527,.T.) ;
#3700=FACE_OUTER_BOUND('',#5528,.T.) ;
#3701=FACE_OUTER_BOUND('',#5529,.T.) ;
#3702=FACE_OUTER_BOUND('',#5530,.T.) ;
#3703=FACE_OUTER_BOUND('',#5531,.T.) ;
#3704=FACE_OUTER_BOUND('',#5532,.T.) ;
#3705=FACE_OUTER_BOUND('',#5533,.T.) ;
#3706=FACE_OUTER_BOUND('',#5534,.T.) ;
#3707=FACE_OUTER_BOUND('',#5535,.T.) ;
#3708=FACE_OUTER_BOUND('',#5536,.T.) ;
#3709=FACE_OUTER_BOUND('',#5537,.T.) ;
#3710=FACE_OUTER_BOUND('',#5538,.T.) ;
#3711=FACE_OUTER_BOUND('',#5539,.T.) ;
#3712=FACE_OUTER_BOUND('',#5540,.T.) ;
#3713=FACE_OUTER_BOUND('',#5541,.T.) ;
#3714=FACE_OUTER_BOUND('',#5542,.T.) ;
#3715=FACE_OUTER_BOUND('',#5543,.T.) ;
#3716=FACE_OUTER_BOUND('',#5544,.T.) ;
#3717=FACE_OUTER_BOUND('',#5545,.T.) ;
#3718=FACE_OUTER_BOUND('',#5546,.T.) ;
#3719=FACE_OUTER_BOUND('',#5547,.T.) ;
#3720=FACE_OUTER_BOUND('',#5548,.T.) ;
#3721=FACE_OUTER_BOUND('',#5549,.T.) ;
#3722=FACE_OUTER_BOUND('',#5550,.T.) ;
#3723=FACE_OUTER_BOUND('',#5551,.T.) ;
#3724=FACE_OUTER_BOUND('',#5552,.T.) ;
#3725=FACE_OUTER_BOUND('',#5553,.T.) ;
#3726=FACE_OUTER_BOUND('',#5554,.T.) ;
#3727=FACE_OUTER_BOUND('',#5555,.T.) ;
#3728=FACE_OUTER_BOUND('',#5556,.T.) ;
#3729=FACE_OUTER_BOUND('',#5557,.T.) ;
#3730=FACE_OUTER_BOUND('',#5558,.T.) ;
#3731=FACE_OUTER_BOUND('',#5559,.T.) ;
#3732=FACE_OUTER_BOUND('',#5560,.T.) ;
#3733=FACE_OUTER_BOUND('',#5561,.T.) ;
#3734=FACE_OUTER_BOUND('',#5562,.T.) ;
#3735=FACE_OUTER_BOUND('',#5563,.T.) ;
#3736=FACE_OUTER_BOUND('',#5564,.T.) ;
#3737=FACE_OUTER_BOUND('',#5565,.T.) ;
#3738=FACE_OUTER_BOUND('',#5566,.T.) ;
#3739=FACE_OUTER_BOUND('',#5567,.T.) ;
#3740=FACE_OUTER_BOUND('',#5568,.T.) ;
#3741=FACE_OUTER_BOUND('',#5569,.T.) ;
#3742=FACE_OUTER_BOUND('',#5570,.T.) ;
#3743=FACE_OUTER_BOUND('',#5571,.T.) ;
#3744=FACE_OUTER_BOUND('',#5572,.T.) ;
#3745=FACE_OUTER_BOUND('',#5573,.T.) ;
#3746=FACE_OUTER_BOUND('',#5574,.T.) ;
#3747=FACE_OUTER_BOUND('',#5575,.T.) ;
#3748=FACE_OUTER_BOUND('',#5576,.T.) ;
#3749=FACE_OUTER_BOUND('',#5578,.T.) ;
#3750=FACE_OUTER_BOUND('',#5580,.T.) ;
#3751=FACE_OUTER_BOUND('',#5581,.T.) ;
#5296=EDGE_LOOP('',(#24295,#24296,#24297,#24298)) ;
#5297=EDGE_LOOP('',(#24299,#24300)) ;
#5298=EDGE_LOOP('',(#24301,#24302,#24303,#24304)) ;
#5299=EDGE_LOOP('',(#24305)) ;
#5300=EDGE_LOOP('',(#24306)) ;
#5301=EDGE_LOOP('',(#24307)) ;
#5302=EDGE_LOOP('',(#24308)) ;
#5303=EDGE_LOOP('',(#24309,#24310,#24311,#24312,#24313)) ;
#5304=EDGE_LOOP('',(#24314)) ;
#5305=EDGE_LOOP('',(#24315,#24316,#24317,#24318)) ;
#5306=EDGE_LOOP('',(#24319,#24320,#24321,#24322)) ;
#5307=EDGE_LOOP('',(#24323)) ;
#5308=EDGE_LOOP('',(#24324)) ;
#5309=EDGE_LOOP('',(#24325)) ;
#5310=EDGE_LOOP('',(#24326)) ;
#5311=EDGE_LOOP('',(#24327,#24328,#24329,#24330,#24331,#24332,#24333,#24334)) ;
#5312=EDGE_LOOP('',(#24335,#24336,#24337,#24338)) ;
#5313=EDGE_LOOP('',(#24339)) ;
#5314=EDGE_LOOP('',(#24340,#24341,#24342,#24343,#24344,#24345,#24346)) ;
#5315=EDGE_LOOP('',(#24347)) ;
#5316=EDGE_LOOP('',(#24348)) ;
#5317=EDGE_LOOP('',(#24349,#24350,#24351)) ;
#5318=EDGE_LOOP('',(#24352,#24353,#24354)) ;
#5319=EDGE_LOOP('',(#24355,#24356,#24357,#24358)) ;
#5320=EDGE_LOOP('',(#24359,#24360,#24361)) ;
#5321=EDGE_LOOP('',(#24362,#24363,#24364,#24365,#24366,#24367)) ;
#5322=EDGE_LOOP('',(#24368,#24369,#24370)) ;
#5323=EDGE_LOOP('',(#24371,#24372,#24373)) ;
#5324=EDGE_LOOP('',(#24374,#24375,#24376)) ;
#5325=EDGE_LOOP('',(#24377,#24378,#24379,#24380,#24381,#24382)) ;
#5326=EDGE_LOOP('',(#24383,#24384,#24385)) ;
#5327=EDGE_LOOP('',(#24386,#24387,#24388)) ;
#5328=EDGE_LOOP('',(#24389,#24390,#24391)) ;
#5329=EDGE_LOOP('',(#24392,#24393,#24394,#24395,#24396,#24397)) ;
#5330=EDGE_LOOP('',(#24398,#24399,#24400)) ;
#5331=EDGE_LOOP('',(#24401,#24402,#24403)) ;
#5332=EDGE_LOOP('',(#24404,#24405,#24406)) ;
#5333=EDGE_LOOP('',(#24407,#24408,#24409,#24410,#24411,#24412)) ;
#5334=EDGE_LOOP('',(#24413,#24414,#24415)) ;
#5335=EDGE_LOOP('',(#24416,#24417,#24418)) ;
#5336=EDGE_LOOP('',(#24419,#24420,#24421)) ;
#5337=EDGE_LOOP('',(#24422,#24423,#24424,#24425,#24426,#24427)) ;
#5338=EDGE_LOOP('',(#24428,#24429,#24430)) ;
#5339=EDGE_LOOP('',(#24431,#24432,#24433)) ;
#5340=EDGE_LOOP('',(#24434,#24435,#24436)) ;
#5341=EDGE_LOOP('',(#24437,#24438,#24439,#24440,#24441,#24442)) ;
#5342=EDGE_LOOP('',(#24443,#24444,#24445)) ;
#5343=EDGE_LOOP('',(#24446,#24447,#24448)) ;
#5344=EDGE_LOOP('',(#24449,#24450,#24451)) ;
#5345=EDGE_LOOP('',(#24452,#24453,#24454,#24455,#24456,#24457)) ;
#5346=EDGE_LOOP('',(#24458,#24459,#24460)) ;
#5347=EDGE_LOOP('',(#24461,#24462,#24463)) ;
#5348=EDGE_LOOP('',(#24464,#24465,#24466)) ;
#5349=EDGE_LOOP('',(#24467,#24468,#24469,#24470,#24471,#24472)) ;
#5350=EDGE_LOOP('',(#24473,#24474,#24475)) ;
#5351=EDGE_LOOP('',(#24476,#24477,#24478)) ;
#5352=EDGE_LOOP('',(#24479,#24480,#24481)) ;
#5353=EDGE_LOOP('',(#24482,#24483,#24484,#24485,#24486,#24487)) ;
#5354=EDGE_LOOP('',(#24488,#24489,#24490)) ;
#5355=EDGE_LOOP('',(#24491,#24492,#24493)) ;
#5356=EDGE_LOOP('',(#24494,#24495,#24496)) ;
#5357=EDGE_LOOP('',(#24497,#24498,#24499,#24500,#24501,#24502)) ;
#5358=EDGE_LOOP('',(#24503,#24504,#24505)) ;
#5359=EDGE_LOOP('',(#24506,#24507,#24508)) ;
#5360=EDGE_LOOP('',(#24509,#24510,#24511)) ;
#5361=EDGE_LOOP('',(#24512,#24513,#24514,#24515,#24516,#24517)) ;
#5362=EDGE_LOOP('',(#24518,#24519,#24520)) ;
#5363=EDGE_LOOP('',(#24521,#24522,#24523)) ;
#5364=EDGE_LOOP('',(#24524,#24525,#24526)) ;
#5365=EDGE_LOOP('',(#24527,#24528,#24529,#24530,#24531,#24532)) ;
#5366=EDGE_LOOP('',(#24533,#24534,#24535)) ;
#5367=EDGE_LOOP('',(#24536,#24537,#24538)) ;
#5368=EDGE_LOOP('',(#24539,#24540,#24541)) ;
#5369=EDGE_LOOP('',(#24542,#24543,#24544,#24545,#24546,#24547)) ;
#5370=EDGE_LOOP('',(#24548,#24549,#24550)) ;
#5371=EDGE_LOOP('',(#24551,#24552,#24553)) ;
#5372=EDGE_LOOP('',(#24554,#24555,#24556)) ;
#5373=EDGE_LOOP('',(#24557,#24558,#24559,#24560,#24561,#24562)) ;
#5374=EDGE_LOOP('',(#24563,#24564,#24565)) ;
#5375=EDGE_LOOP('',(#24566,#24567,#24568)) ;
#5376=EDGE_LOOP('',(#24569,#24570,#24571)) ;
#5377=EDGE_LOOP('',(#24572,#24573,#24574,#24575,#24576,#24577)) ;
#5378=EDGE_LOOP('',(#24578,#24579,#24580)) ;
#5379=EDGE_LOOP('',(#24581,#24582,#24583)) ;
#5380=EDGE_LOOP('',(#24584,#24585,#24586)) ;
#5381=EDGE_LOOP('',(#24587,#24588,#24589,#24590,#24591,#24592)) ;
#5382=EDGE_LOOP('',(#24593,#24594,#24595)) ;
#5383=EDGE_LOOP('',(#24596,#24597,#24598)) ;
#5384=EDGE_LOOP('',(#24599,#24600,#24601)) ;
#5385=EDGE_LOOP('',(#24602,#24603,#24604,#24605,#24606,#24607)) ;
#5386=EDGE_LOOP('',(#24608,#24609,#24610)) ;
#5387=EDGE_LOOP('',(#24611,#24612,#24613)) ;
#5388=EDGE_LOOP('',(#24614,#24615,#24616)) ;
#5389=EDGE_LOOP('',(#24617,#24618,#24619,#24620,#24621,#24622)) ;
#5390=EDGE_LOOP('',(#24623,#24624,#24625)) ;
#5391=EDGE_LOOP('',(#24626,#24627,#24628)) ;
#5392=EDGE_LOOP('',(#24629,#24630,#24631)) ;
#5393=EDGE_LOOP('',(#24632,#24633,#24634,#24635,#24636,#24637)) ;
#5394=EDGE_LOOP('',(#24638,#24639,#24640)) ;
#5395=EDGE_LOOP('',(#24641,#24642,#24643)) ;
#5396=EDGE_LOOP('',(#24644,#24645,#24646)) ;
#5397=EDGE_LOOP('',(#24647,#24648,#24649,#24650,#24651,#24652)) ;
#5398=EDGE_LOOP('',(#24653,#24654,#24655)) ;
#5399=EDGE_LOOP('',(#24656,#24657,#24658)) ;
#5400=EDGE_LOOP('',(#24659,#24660,#24661)) ;
#5401=EDGE_LOOP('',(#24662,#24663,#24664,#24665,#24666,#24667)) ;
#5402=EDGE_LOOP('',(#24668,#24669,#24670)) ;
#5403=EDGE_LOOP('',(#24671,#24672,#24673)) ;
#5404=EDGE_LOOP('',(#24674,#24675,#24676)) ;
#5405=EDGE_LOOP('',(#24677,#24678,#24679,#24680,#24681,#24682)) ;
#5406=EDGE_LOOP('',(#24683,#24684,#24685)) ;
#5407=EDGE_LOOP('',(#24686,#24687,#24688)) ;
#5408=EDGE_LOOP('',(#24689,#24690,#24691)) ;
#5409=EDGE_LOOP('',(#24692,#24693,#24694,#24695,#24696,#24697)) ;
#5410=EDGE_LOOP('',(#24698,#24699,#24700)) ;
#5411=EDGE_LOOP('',(#24701,#24702,#24703)) ;
#5412=EDGE_LOOP('',(#24704,#24705,#24706)) ;
#5413=EDGE_LOOP('',(#24707,#24708,#24709,#24710,#24711,#24712)) ;
#5414=EDGE_LOOP('',(#24713,#24714,#24715)) ;
#5415=EDGE_LOOP('',(#24716,#24717,#24718)) ;
#5416=EDGE_LOOP('',(#24719,#24720,#24721)) ;
#5417=EDGE_LOOP('',(#24722,#24723,#24724,#24725,#24726,#24727)) ;
#5418=EDGE_LOOP('',(#24728,#24729,#24730)) ;
#5419=EDGE_LOOP('',(#24731,#24732,#24733)) ;
#5420=EDGE_LOOP('',(#24734,#24735,#24736)) ;
#5421=EDGE_LOOP('',(#24737,#24738,#24739,#24740,#24741,#24742)) ;
#5422=EDGE_LOOP('',(#24743,#24744,#24745)) ;
#5423=EDGE_LOOP('',(#24746,#24747,#24748)) ;
#5424=EDGE_LOOP('',(#24749,#24750,#24751)) ;
#5425=EDGE_LOOP('',(#24752,#24753,#24754,#24755,#24756,#24757)) ;
#5426=EDGE_LOOP('',(#24758,#24759,#24760)) ;
#5427=EDGE_LOOP('',(#24761,#24762,#24763)) ;
#5428=EDGE_LOOP('',(#24764,#24765,#24766)) ;
#5429=EDGE_LOOP('',(#24767,#24768,#24769,#24770,#24771,#24772)) ;
#5430=EDGE_LOOP('',(#24773,#24774,#24775)) ;
#5431=EDGE_LOOP('',(#24776,#24777,#24778)) ;
#5432=EDGE_LOOP('',(#24779,#24780,#24781)) ;
#5433=EDGE_LOOP('',(#24782,#24783,#24784,#24785,#24786,#24787)) ;
#5434=EDGE_LOOP('',(#24788,#24789,#24790)) ;
#5435=EDGE_LOOP('',(#24791,#24792,#24793)) ;
#5436=EDGE_LOOP('',(#24794,#24795,#24796)) ;
#5437=EDGE_LOOP('',(#24797,#24798,#24799,#24800,#24801,#24802)) ;
#5438=EDGE_LOOP('',(#24803,#24804,#24805)) ;
#5439=EDGE_LOOP('',(#24806,#24807,#24808)) ;
#5440=EDGE_LOOP('',(#24809,#24810,#24811)) ;
#5441=EDGE_LOOP('',(#24812,#24813,#24814,#24815,#24816,#24817)) ;
#5442=EDGE_LOOP('',(#24818,#24819,#24820)) ;
#5443=EDGE_LOOP('',(#24821,#24822,#24823)) ;
#5444=EDGE_LOOP('',(#24824,#24825,#24826)) ;
#5445=EDGE_LOOP('',(#24827,#24828,#24829,#24830,#24831)) ;
#5446=EDGE_LOOP('',(#24832,#24833,#24834,#24835,#24836,#24837)) ;
#5447=EDGE_LOOP('',(#24838,#24839,#24840,#24841,#24842,#24843,#24844,#24845,
#24846,#24847)) ;
#5448=EDGE_LOOP('',(#24848,#24849,#24850,#24851,#24852,#24853,#24854,#24855,
#24856)) ;
#5449=EDGE_LOOP('',(#24857,#24858,#24859,#24860,#24861,#24862,#24863,#24864,
#24865,#24866)) ;
#5450=EDGE_LOOP('',(#24867,#24868,#24869,#24870,#24871,#24872,#24873,#24874,
#24875)) ;
#5451=EDGE_LOOP('',(#24876,#24877,#24878,#24879,#24880,#24881,#24882,#24883,
#24884)) ;
#5452=EDGE_LOOP('',(#24885,#24886,#24887,#24888,#24889,#24890,#24891,#24892,
#24893)) ;
#5453=EDGE_LOOP('',(#24894,#24895,#24896,#24897,#24898,#24899,#24900,#24901,
#24902,#24903)) ;
#5454=EDGE_LOOP('',(#24904,#24905,#24906,#24907,#24908,#24909,#24910,#24911,
#24912)) ;
#5455=EDGE_LOOP('',(#24913,#24914,#24915,#24916,#24917,#24918,#24919,#24920,
#24921)) ;
#5456=EDGE_LOOP('',(#24922,#24923,#24924,#24925,#24926,#24927,#24928,#24929,
#24930)) ;
#5457=EDGE_LOOP('',(#24931,#24932,#24933,#24934,#24935,#24936,#24937,#24938,
#24939,#24940)) ;
#5458=EDGE_LOOP('',(#24941,#24942,#24943,#24944,#24945,#24946,#24947,#24948,
#24949)) ;
#5459=EDGE_LOOP('',(#24950,#24951,#24952,#24953,#24954,#24955,#24956,#24957,
#24958)) ;
#5460=EDGE_LOOP('',(#24959,#24960,#24961,#24962,#24963,#24964,#24965,#24966,
#24967)) ;
#5461=EDGE_LOOP('',(#24968,#24969,#24970,#24971,#24972,#24973,#24974,#24975,
#24976,#24977)) ;
#5462=EDGE_LOOP('',(#24978,#24979,#24980,#24981,#24982,#24983,#24984,#24985,
#24986)) ;
#5463=EDGE_LOOP('',(#24987,#24988,#24989,#24990,#24991,#24992,#24993,#24994,
#24995)) ;
#5464=EDGE_LOOP('',(#24996,#24997,#24998,#24999,#25000,#25001,#25002,#25003,
#25004)) ;
#5465=EDGE_LOOP('',(#25005,#25006,#25007,#25008,#25009,#25010,#25011,#25012,
#25013,#25014)) ;
#5466=EDGE_LOOP('',(#25015,#25016,#25017,#25018,#25019,#25020,#25021,#25022,
#25023)) ;
#5467=EDGE_LOOP('',(#25024,#25025,#25026,#25027,#25028,#25029,#25030,#25031,
#25032)) ;
#5468=EDGE_LOOP('',(#25033,#25034,#25035,#25036,#25037,#25038,#25039,#25040,
#25041)) ;
#5469=EDGE_LOOP('',(#25042,#25043,#25044,#25045,#25046,#25047,#25048,#25049,
#25050,#25051)) ;
#5470=EDGE_LOOP('',(#25052,#25053,#25054,#25055,#25056,#25057,#25058,#25059,
#25060)) ;
#5471=EDGE_LOOP('',(#25061,#25062,#25063,#25064,#25065,#25066,#25067,#25068,
#25069)) ;
#5472=EDGE_LOOP('',(#25070,#25071,#25072,#25073,#25074,#25075,#25076,#25077,
#25078)) ;
#5473=EDGE_LOOP('',(#25079,#25080,#25081,#25082,#25083,#25084,#25085,#25086,
#25087,#25088)) ;
#5474=EDGE_LOOP('',(#25089,#25090,#25091,#25092,#25093,#25094,#25095,#25096,
#25097)) ;
#5475=EDGE_LOOP('',(#25098,#25099,#25100,#25101,#25102,#25103,#25104,#25105,
#25106)) ;
#5476=EDGE_LOOP('',(#25107,#25108,#25109,#25110,#25111,#25112,#25113,#25114,
#25115)) ;
#5477=EDGE_LOOP('',(#25116,#25117,#25118,#25119,#25120,#25121,#25122,#25123,
#25124,#25125)) ;
#5478=EDGE_LOOP('',(#25126,#25127,#25128,#25129,#25130,#25131,#25132,#25133,
#25134)) ;
#5479=EDGE_LOOP('',(#25135,#25136,#25137,#25138,#25139,#25140,#25141,#25142,
#25143)) ;
#5480=EDGE_LOOP('',(#25144,#25145,#25146,#25147,#25148,#25149,#25150,#25151,
#25152)) ;
#5481=EDGE_LOOP('',(#25153,#25154,#25155,#25156,#25157,#25158,#25159,#25160,
#25161,#25162)) ;
#5482=EDGE_LOOP('',(#25163,#25164,#25165,#25166,#25167,#25168,#25169,#25170,
#25171)) ;
#5483=EDGE_LOOP('',(#25172,#25173,#25174,#25175,#25176,#25177,#25178,#25179,
#25180)) ;
#5484=EDGE_LOOP('',(#25181,#25182,#25183,#25184,#25185,#25186,#25187,#25188,
#25189)) ;
#5485=EDGE_LOOP('',(#25190,#25191,#25192,#25193,#25194,#25195,#25196,#25197,
#25198,#25199)) ;
#5486=EDGE_LOOP('',(#25200,#25201,#25202,#25203,#25204,#25205,#25206,#25207,
#25208)) ;
#5487=EDGE_LOOP('',(#25209,#25210,#25211,#25212,#25213,#25214,#25215,#25216,
#25217)) ;
#5488=EDGE_LOOP('',(#25218,#25219,#25220,#25221,#25222,#25223,#25224,#25225,
#25226)) ;
#5489=EDGE_LOOP('',(#25227,#25228,#25229,#25230,#25231,#25232,#25233,#25234,
#25235,#25236)) ;
#5490=EDGE_LOOP('',(#25237,#25238,#25239,#25240,#25241,#25242,#25243,#25244,
#25245)) ;
#5491=EDGE_LOOP('',(#25246,#25247,#25248,#25249,#25250,#25251,#25252,#25253,
#25254)) ;
#5492=EDGE_LOOP('',(#25255,#25256,#25257,#25258,#25259,#25260,#25261,#25262,
#25263)) ;
#5493=EDGE_LOOP('',(#25264,#25265,#25266,#25267,#25268,#25269,#25270,#25271,
#25272,#25273)) ;
#5494=EDGE_LOOP('',(#25274,#25275,#25276,#25277,#25278,#25279,#25280,#25281,
#25282)) ;
#5495=EDGE_LOOP('',(#25283,#25284,#25285,#25286,#25287,#25288,#25289,#25290,
#25291)) ;
#5496=EDGE_LOOP('',(#25292,#25293,#25294,#25295,#25296,#25297,#25298,#25299,
#25300)) ;
#5497=EDGE_LOOP('',(#25301,#25302,#25303,#25304,#25305,#25306,#25307,#25308,
#25309,#25310)) ;
#5498=EDGE_LOOP('',(#25311,#25312,#25313,#25314,#25315,#25316,#25317,#25318,
#25319)) ;
#5499=EDGE_LOOP('',(#25320,#25321,#25322,#25323,#25324,#25325,#25326,#25327,
#25328)) ;
#5500=EDGE_LOOP('',(#25329,#25330,#25331,#25332,#25333,#25334,#25335,#25336,
#25337)) ;
#5501=EDGE_LOOP('',(#25338,#25339,#25340,#25341,#25342,#25343,#25344,#25345,
#25346,#25347)) ;
#5502=EDGE_LOOP('',(#25348,#25349,#25350,#25351,#25352,#25353,#25354,#25355,
#25356)) ;
#5503=EDGE_LOOP('',(#25357,#25358,#25359,#25360,#25361,#25362,#25363,#25364,
#25365)) ;
#5504=EDGE_LOOP('',(#25366,#25367,#25368,#25369,#25370,#25371,#25372,#25373,
#25374)) ;
#5505=EDGE_LOOP('',(#25375,#25376,#25377,#25378,#25379,#25380,#25381,#25382,
#25383,#25384)) ;
#5506=EDGE_LOOP('',(#25385,#25386,#25387,#25388,#25389,#25390,#25391,#25392,
#25393)) ;
#5507=EDGE_LOOP('',(#25394,#25395,#25396,#25397,#25398,#25399,#25400,#25401,
#25402)) ;
#5508=EDGE_LOOP('',(#25403,#25404,#25405,#25406,#25407,#25408,#25409,#25410,
#25411)) ;
#5509=EDGE_LOOP('',(#25412,#25413,#25414,#25415,#25416,#25417,#25418,#25419,
#25420,#25421)) ;
#5510=EDGE_LOOP('',(#25422,#25423,#25424,#25425,#25426,#25427,#25428,#25429,
#25430)) ;
#5511=EDGE_LOOP('',(#25431,#25432,#25433,#25434,#25435,#25436,#25437,#25438,
#25439)) ;
#5512=EDGE_LOOP('',(#25440,#25441,#25442,#25443,#25444,#25445,#25446,#25447,
#25448)) ;
#5513=EDGE_LOOP('',(#25449,#25450,#25451,#25452,#25453,#25454,#25455,#25456,
#25457,#25458)) ;
#5514=EDGE_LOOP('',(#25459,#25460,#25461,#25462,#25463,#25464,#25465,#25466,
#25467)) ;
#5515=EDGE_LOOP('',(#25468,#25469,#25470,#25471,#25472,#25473,#25474,#25475,
#25476)) ;
#5516=EDGE_LOOP('',(#25477,#25478,#25479,#25480,#25481,#25482,#25483,#25484,
#25485)) ;
#5517=EDGE_LOOP('',(#25486,#25487,#25488,#25489,#25490,#25491,#25492,#25493,
#25494,#25495)) ;
#5518=EDGE_LOOP('',(#25496,#25497,#25498,#25499,#25500,#25501,#25502,#25503,
#25504)) ;
#5519=EDGE_LOOP('',(#25505,#25506,#25507,#25508,#25509,#25510,#25511,#25512,
#25513)) ;
#5520=EDGE_LOOP('',(#25514,#25515,#25516,#25517,#25518,#25519,#25520,#25521,
#25522)) ;
#5521=EDGE_LOOP('',(#25523,#25524,#25525,#25526,#25527,#25528,#25529,#25530,
#25531,#25532)) ;
#5522=EDGE_LOOP('',(#25533,#25534,#25535,#25536,#25537,#25538,#25539,#25540,
#25541)) ;
#5523=EDGE_LOOP('',(#25542,#25543,#25544,#25545,#25546,#25547,#25548,#25549,
#25550)) ;
#5524=EDGE_LOOP('',(#25551,#25552,#25553,#25554,#25555,#25556,#25557,#25558,
#25559)) ;
#5525=EDGE_LOOP('',(#25560,#25561,#25562,#25563,#25564,#25565,#25566,#25567,
#25568,#25569)) ;
#5526=EDGE_LOOP('',(#25570,#25571,#25572,#25573,#25574,#25575,#25576,#25577,
#25578)) ;
#5527=EDGE_LOOP('',(#25579,#25580,#25581,#25582,#25583,#25584,#25585,#25586,
#25587)) ;
#5528=EDGE_LOOP('',(#25588,#25589,#25590,#25591,#25592,#25593,#25594,#25595,
#25596)) ;
#5529=EDGE_LOOP('',(#25597,#25598,#25599,#25600,#25601,#25602,#25603,#25604,
#25605,#25606)) ;
#5530=EDGE_LOOP('',(#25607,#25608,#25609,#25610,#25611,#25612,#25613,#25614,
#25615)) ;
#5531=EDGE_LOOP('',(#25616,#25617,#25618,#25619,#25620,#25621,#25622,#25623,
#25624)) ;
#5532=EDGE_LOOP('',(#25625,#25626,#25627,#25628,#25629,#25630,#25631,#25632,
#25633)) ;
#5533=EDGE_LOOP('',(#25634,#25635,#25636,#25637,#25638,#25639,#25640,#25641,
#25642,#25643)) ;
#5534=EDGE_LOOP('',(#25644,#25645,#25646,#25647,#25648,#25649,#25650,#25651,
#25652)) ;
#5535=EDGE_LOOP('',(#25653,#25654,#25655,#25656,#25657,#25658,#25659,#25660,
#25661)) ;
#5536=EDGE_LOOP('',(#25662,#25663,#25664,#25665,#25666,#25667,#25668,#25669,
#25670)) ;
#5537=EDGE_LOOP('',(#25671,#25672,#25673,#25674,#25675,#25676,#25677,#25678,
#25679,#25680)) ;
#5538=EDGE_LOOP('',(#25681,#25682,#25683,#25684,#25685,#25686,#25687,#25688,
#25689)) ;
#5539=EDGE_LOOP('',(#25690,#25691,#25692,#25693,#25694,#25695,#25696,#25697,
#25698)) ;
#5540=EDGE_LOOP('',(#25699,#25700,#25701,#25702,#25703,#25704,#25705,#25706,
#25707)) ;
#5541=EDGE_LOOP('',(#25708,#25709,#25710,#25711,#25712,#25713,#25714,#25715,
#25716,#25717)) ;
#5542=EDGE_LOOP('',(#25718,#25719,#25720,#25721,#25722,#25723,#25724,#25725,
#25726)) ;
#5543=EDGE_LOOP('',(#25727,#25728,#25729,#25730,#25731,#25732,#25733,#25734,
#25735)) ;
#5544=EDGE_LOOP('',(#25736,#25737,#25738,#25739,#25740,#25741,#25742,#25743,
#25744)) ;
#5545=EDGE_LOOP('',(#25745,#25746,#25747,#25748,#25749,#25750,#25751,#25752,
#25753,#25754)) ;
#5546=EDGE_LOOP('',(#25755,#25756,#25757,#25758,#25759,#25760,#25761,#25762,
#25763)) ;
#5547=EDGE_LOOP('',(#25764,#25765,#25766,#25767,#25768,#25769,#25770,#25771,
#25772)) ;
#5548=EDGE_LOOP('',(#25773,#25774,#25775,#25776,#25777,#25778,#25779,#25780,
#25781)) ;
#5549=EDGE_LOOP('',(#25782,#25783,#25784,#25785,#25786,#25787,#25788,#25789,
#25790,#25791)) ;
#5550=EDGE_LOOP('',(#25792,#25793,#25794,#25795,#25796,#25797,#25798,#25799,
#25800)) ;
#5551=EDGE_LOOP('',(#25801,#25802,#25803,#25804,#25805,#25806,#25807,#25808,
#25809)) ;
#5552=EDGE_LOOP('',(#25810,#25811,#25812,#25813,#25814,#25815,#25816,#25817,
#25818)) ;
#5553=EDGE_LOOP('',(#25819,#25820,#25821,#25822,#25823,#25824,#25825,#25826,
#25827,#25828)) ;
#5554=EDGE_LOOP('',(#25829,#25830,#25831,#25832,#25833,#25834,#25835,#25836,
#25837)) ;
#5555=EDGE_LOOP('',(#25838,#25839,#25840,#25841,#25842,#25843,#25844,#25845,
#25846)) ;
#5556=EDGE_LOOP('',(#25847,#25848,#25849,#25850,#25851,#25852,#25853,#25854,
#25855)) ;
#5557=EDGE_LOOP('',(#25856,#25857,#25858,#25859,#25860,#25861,#25862,#25863,
#25864,#25865)) ;
#5558=EDGE_LOOP('',(#25866,#25867,#25868,#25869,#25870,#25871,#25872,#25873,
#25874)) ;
#5559=EDGE_LOOP('',(#25875,#25876,#25877,#25878,#25879,#25880,#25881,#25882,
#25883)) ;
#5560=EDGE_LOOP('',(#25884,#25885,#25886,#25887,#25888,#25889,#25890,#25891,
#25892)) ;
#5561=EDGE_LOOP('',(#25893,#25894,#25895,#25896,#25897,#25898,#25899,#25900,
#25901,#25902)) ;
#5562=EDGE_LOOP('',(#25903,#25904,#25905,#25906,#25907,#25908,#25909,#25910,
#25911)) ;
#5563=EDGE_LOOP('',(#25912,#25913,#25914,#25915,#25916,#25917,#25918,#25919,
#25920)) ;
#5564=EDGE_LOOP('',(#25921,#25922,#25923,#25924,#25925,#25926,#25927,#25928,
#25929)) ;
#5565=EDGE_LOOP('',(#25930,#25931,#25932,#25933,#25934,#25935,#25936,#25937,
#25938,#25939)) ;
#5566=EDGE_LOOP('',(#25940,#25941,#25942,#25943,#25944,#25945,#25946,#25947,
#25948)) ;
#5567=EDGE_LOOP('',(#25949,#25950,#25951,#25952,#25953,#25954,#25955,#25956,
#25957)) ;
#5568=EDGE_LOOP('',(#25958,#25959,#25960,#25961,#25962,#25963,#25964,#25965,
#25966)) ;
#5569=EDGE_LOOP('',(#25967,#25968,#25969,#25970,#25971,#25972,#25973,#25974,
#25975,#25976)) ;
#5570=EDGE_LOOP('',(#25977,#25978,#25979,#25980,#25981,#25982,#25983,#25984,
#25985)) ;
#5571=EDGE_LOOP('',(#25986,#25987,#25988,#25989,#25990,#25991,#25992,#25993,
#25994)) ;
#5572=EDGE_LOOP('',(#25995,#25996,#25997,#25998,#25999,#26000,#26001)) ;
#5573=EDGE_LOOP('',(#26002)) ;
#5574=EDGE_LOOP('',(#26003,#26004,#26005,#26006,#26007,#26008,#26009,#26010,
#26011)) ;
#5575=EDGE_LOOP('',(#26012,#26013,#26014,#26015)) ;
#5576=EDGE_LOOP('',(#26016)) ;
#5577=EDGE_LOOP('',(#26017)) ;
#5578=EDGE_LOOP('',(#26018)) ;
#5579=EDGE_LOOP('',(#26019)) ;
#5580=EDGE_LOOP('',(#26020,#26021,#26022,#26023,#26024,#26025)) ;
#5581=EDGE_LOOP('',(#26026)) ;
#7901=LINE('',#47525,#10373) ;
#7902=LINE('',#47569,#10374) ;
#7903=LINE('',#47576,#10375) ;
#7904=LINE('',#47582,#10376) ;
#7905=LINE('',#47588,#10377) ;
#7906=LINE('',#47627,#10378) ;
#7907=LINE('',#47633,#10379) ;
#7908=LINE('',#47637,#10380) ;
#7909=LINE('',#48665,#10381) ;
#7910=LINE('',#48670,#10382) ;
#7911=LINE('',#48675,#10383) ;
#7912=LINE('',#48680,#10384) ;
#7913=LINE('',#48685,#10385) ;
#7914=LINE('',#48690,#10386) ;
#7915=LINE('',#48695,#10387) ;
#7916=LINE('',#48700,#10388) ;
#7917=LINE('',#48705,#10389) ;
#7918=LINE('',#48710,#10390) ;
#7919=LINE('',#48715,#10391) ;
#7920=LINE('',#48720,#10392) ;
#7921=LINE('',#48725,#10393) ;
#7922=LINE('',#48730,#10394) ;
#7923=LINE('',#48735,#10395) ;
#7924=LINE('',#48740,#10396) ;
#7925=LINE('',#48745,#10397) ;
#7926=LINE('',#48750,#10398) ;
#7927=LINE('',#48755,#10399) ;
#7928=LINE('',#48760,#10400) ;
#7929=LINE('',#48765,#10401) ;
#7930=LINE('',#48770,#10402) ;
#7931=LINE('',#48775,#10403) ;
#7932=LINE('',#48780,#10404) ;
#7933=LINE('',#48785,#10405) ;
#7934=LINE('',#48790,#10406) ;
#7935=LINE('',#48795,#10407) ;
#7936=LINE('',#48800,#10408) ;
#7937=LINE('',#48805,#10409) ;
#7938=LINE('',#48810,#10410) ;
#7939=LINE('',#48815,#10411) ;
#7940=LINE('',#48820,#10412) ;
#7941=LINE('',#48825,#10413) ;
#7942=LINE('',#48830,#10414) ;
#7943=LINE('',#48835,#10415) ;
#7944=LINE('',#48840,#10416) ;
#7945=LINE('',#48845,#10417) ;
#7946=LINE('',#48850,#10418) ;
#7947=LINE('',#48855,#10419) ;
#7948=LINE('',#48860,#10420) ;
#7949=LINE('',#48865,#10421) ;
#7950=LINE('',#48870,#10422) ;
#7951=LINE('',#48875,#10423) ;
#7952=LINE('',#48880,#10424) ;
#7953=LINE('',#48885,#10425) ;
#7954=LINE('',#48890,#10426) ;
#7955=LINE('',#48895,#10427) ;
#7956=LINE('',#48900,#10428) ;
#7957=LINE('',#48905,#10429) ;
#7958=LINE('',#48910,#10430) ;
#7959=LINE('',#48915,#10431) ;
#7960=LINE('',#48920,#10432) ;
#7961=LINE('',#48925,#10433) ;
#7962=LINE('',#48930,#10434) ;
#7963=LINE('',#48935,#10435) ;
#7964=LINE('',#48940,#10436) ;
#7965=LINE('',#48945,#10437) ;
#7966=LINE('',#48950,#10438) ;
#7967=LINE('',#48955,#10439) ;
#7968=LINE('',#48960,#10440) ;
#7969=LINE('',#48965,#10441) ;
#7970=LINE('',#48970,#10442) ;
#7971=LINE('',#48975,#10443) ;
#7972=LINE('',#48980,#10444) ;
#7973=LINE('',#48985,#10445) ;
#7974=LINE('',#48990,#10446) ;
#7975=LINE('',#48995,#10447) ;
#7976=LINE('',#49000,#10448) ;
#7977=LINE('',#49005,#10449) ;
#7978=LINE('',#49010,#10450) ;
#7979=LINE('',#49015,#10451) ;
#7980=LINE('',#49020,#10452) ;
#7981=LINE('',#49025,#10453) ;
#7982=LINE('',#49030,#10454) ;
#7983=LINE('',#49035,#10455) ;
#7984=LINE('',#49040,#10456) ;
#7985=LINE('',#49045,#10457) ;
#7986=LINE('',#49050,#10458) ;
#7987=LINE('',#49055,#10459) ;
#7988=LINE('',#49060,#10460) ;
#7989=LINE('',#49065,#10461) ;
#7990=LINE('',#49070,#10462) ;
#7991=LINE('',#49075,#10463) ;
#7992=LINE('',#49080,#10464) ;
#7993=LINE('',#49085,#10465) ;
#7994=LINE('',#49090,#10466) ;
#7995=LINE('',#49095,#10467) ;
#7996=LINE('',#49100,#10468) ;
#7997=LINE('',#49105,#10469) ;
#7998=LINE('',#49110,#10470) ;
#7999=LINE('',#49115,#10471) ;
#8000=LINE('',#49120,#10472) ;
#8001=LINE('',#49125,#10473) ;
#8002=LINE('',#49130,#10474) ;
#8003=LINE('',#49135,#10475) ;
#8004=LINE('',#49140,#10476) ;
#8005=LINE('',#49145,#10477) ;
#8006=LINE('',#49150,#10478) ;
#8007=LINE('',#49155,#10479) ;
#8008=LINE('',#49160,#10480) ;
#8009=LINE('',#49165,#10481) ;
#8010=LINE('',#49170,#10482) ;
#8011=LINE('',#49175,#10483) ;
#8012=LINE('',#49180,#10484) ;
#8013=LINE('',#49185,#10485) ;
#8014=LINE('',#49190,#10486) ;
#8015=LINE('',#49195,#10487) ;
#8016=LINE('',#49200,#10488) ;
#8017=LINE('',#49205,#10489) ;
#8018=LINE('',#49210,#10490) ;
#8019=LINE('',#49215,#10491) ;
#8020=LINE('',#49220,#10492) ;
#8021=LINE('',#49225,#10493) ;
#8022=LINE('',#49230,#10494) ;
#8023=LINE('',#49235,#10495) ;
#8024=LINE('',#49240,#10496) ;
#8025=LINE('',#49245,#10497) ;
#8026=LINE('',#49250,#10498) ;
#8027=LINE('',#49255,#10499) ;
#8028=LINE('',#49260,#10500) ;
#8029=LINE('',#49265,#10501) ;
#8030=LINE('',#49270,#10502) ;
#8031=LINE('',#49275,#10503) ;
#8032=LINE('',#49280,#10504) ;
#8033=LINE('',#49285,#10505) ;
#8034=LINE('',#49290,#10506) ;
#8035=LINE('',#49297,#10507) ;
#8036=LINE('',#49318,#10508) ;
#8037=LINE('',#49345,#10509) ;
#8038=LINE('',#49351,#10510) ;
#10373=VECTOR('',#38270,0.55) ;
#10374=VECTOR('',#38277,0.25) ;
#10375=VECTOR('',#38288,0.15) ;
#10376=VECTOR('',#38295,0.8) ;
#10377=VECTOR('',#38302,1.1) ;
#10378=VECTOR('',#38315,0.8) ;
#10379=VECTOR('',#38322,1.1) ;
#10380=VECTOR('',#38327,1.) ;
#10381=VECTOR('',#39492,0.15) ;
#10382=VECTOR('',#39499,0.15) ;
#10383=VECTOR('',#39506,0.15) ;
#10384=VECTOR('',#39513,0.15) ;
#10385=VECTOR('',#39520,0.15) ;
#10386=VECTOR('',#39527,0.15) ;
#10387=VECTOR('',#39534,0.15) ;
#10388=VECTOR('',#39541,0.15) ;
#10389=VECTOR('',#39548,0.15) ;
#10390=VECTOR('',#39555,0.15) ;
#10391=VECTOR('',#39562,0.15) ;
#10392=VECTOR('',#39569,0.15) ;
#10393=VECTOR('',#39576,0.15) ;
#10394=VECTOR('',#39583,0.15) ;
#10395=VECTOR('',#39590,0.15) ;
#10396=VECTOR('',#39597,0.15) ;
#10397=VECTOR('',#39604,0.15) ;
#10398=VECTOR('',#39611,0.15) ;
#10399=VECTOR('',#39618,0.15) ;
#10400=VECTOR('',#39625,0.15) ;
#10401=VECTOR('',#39632,0.15) ;
#10402=VECTOR('',#39639,0.15) ;
#10403=VECTOR('',#39646,0.15) ;
#10404=VECTOR('',#39653,0.15) ;
#10405=VECTOR('',#39660,0.15) ;
#10406=VECTOR('',#39667,0.15) ;
#10407=VECTOR('',#39674,0.15) ;
#10408=VECTOR('',#39681,0.15) ;
#10409=VECTOR('',#39688,0.15) ;
#10410=VECTOR('',#39695,0.15) ;
#10411=VECTOR('',#39702,0.15) ;
#10412=VECTOR('',#39709,0.15) ;
#10413=VECTOR('',#39716,0.15) ;
#10414=VECTOR('',#39723,0.15) ;
#10415=VECTOR('',#39730,0.15) ;
#10416=VECTOR('',#39737,0.15) ;
#10417=VECTOR('',#39744,0.15) ;
#10418=VECTOR('',#39751,0.15) ;
#10419=VECTOR('',#39758,0.15) ;
#10420=VECTOR('',#39765,0.15) ;
#10421=VECTOR('',#39772,0.15) ;
#10422=VECTOR('',#39779,0.15) ;
#10423=VECTOR('',#39786,0.15) ;
#10424=VECTOR('',#39793,0.15) ;
#10425=VECTOR('',#39800,0.15) ;
#10426=VECTOR('',#39807,0.15) ;
#10427=VECTOR('',#39814,0.15) ;
#10428=VECTOR('',#39821,0.15) ;
#10429=VECTOR('',#39828,0.15) ;
#10430=VECTOR('',#39835,0.15) ;
#10431=VECTOR('',#39842,0.15) ;
#10432=VECTOR('',#39849,0.15) ;
#10433=VECTOR('',#39856,0.15) ;
#10434=VECTOR('',#39863,0.15) ;
#10435=VECTOR('',#39870,0.15) ;
#10436=VECTOR('',#39877,0.15) ;
#10437=VECTOR('',#39884,0.15) ;
#10438=VECTOR('',#39891,0.15) ;
#10439=VECTOR('',#39898,0.15) ;
#10440=VECTOR('',#39905,0.15) ;
#10441=VECTOR('',#39912,0.15) ;
#10442=VECTOR('',#39919,0.15) ;
#10443=VECTOR('',#39926,0.15) ;
#10444=VECTOR('',#39933,0.15) ;
#10445=VECTOR('',#39940,0.15) ;
#10446=VECTOR('',#39947,0.15) ;
#10447=VECTOR('',#39954,0.15) ;
#10448=VECTOR('',#39961,0.15) ;
#10449=VECTOR('',#39968,0.15) ;
#10450=VECTOR('',#39975,0.15) ;
#10451=VECTOR('',#39982,0.15) ;
#10452=VECTOR('',#39989,0.15) ;
#10453=VECTOR('',#39996,0.15) ;
#10454=VECTOR('',#40003,0.15) ;
#10455=VECTOR('',#40010,0.15) ;
#10456=VECTOR('',#40017,0.15) ;
#10457=VECTOR('',#40024,0.15) ;
#10458=VECTOR('',#40031,0.15) ;
#10459=VECTOR('',#40038,0.15) ;
#10460=VECTOR('',#40045,0.15) ;
#10461=VECTOR('',#40052,0.15) ;
#10462=VECTOR('',#40059,0.15) ;
#10463=VECTOR('',#40066,0.15) ;
#10464=VECTOR('',#40073,0.15) ;
#10465=VECTOR('',#40080,0.15) ;
#10466=VECTOR('',#40087,0.15) ;
#10467=VECTOR('',#40094,0.15) ;
#10468=VECTOR('',#40101,0.15) ;
#10469=VECTOR('',#40108,0.15) ;
#10470=VECTOR('',#40115,0.15) ;
#10471=VECTOR('',#40122,0.15) ;
#10472=VECTOR('',#40129,0.15) ;
#10473=VECTOR('',#40136,0.15) ;
#10474=VECTOR('',#40143,0.15) ;
#10475=VECTOR('',#40150,0.15) ;
#10476=VECTOR('',#40157,0.15) ;
#10477=VECTOR('',#40164,0.15) ;
#10478=VECTOR('',#40171,0.15) ;
#10479=VECTOR('',#40178,0.15) ;
#10480=VECTOR('',#40185,0.15) ;
#10481=VECTOR('',#40192,0.15) ;
#10482=VECTOR('',#40199,0.15) ;
#10483=VECTOR('',#40206,0.15) ;
#10484=VECTOR('',#40213,0.15) ;
#10485=VECTOR('',#40220,0.15) ;
#10486=VECTOR('',#40227,0.15) ;
#10487=VECTOR('',#40234,0.15) ;
#10488=VECTOR('',#40241,0.15) ;
#10489=VECTOR('',#40248,0.15) ;
#10490=VECTOR('',#40255,0.15) ;
#10491=VECTOR('',#40262,0.15) ;
#10492=VECTOR('',#40269,0.15) ;
#10493=VECTOR('',#40276,0.15) ;
#10494=VECTOR('',#40283,0.15) ;
#10495=VECTOR('',#40290,0.15) ;
#10496=VECTOR('',#40297,0.15) ;
#10497=VECTOR('',#40304,0.15) ;
#10498=VECTOR('',#40311,0.15) ;
#10499=VECTOR('',#40318,0.15) ;
#10500=VECTOR('',#40325,0.15) ;
#10501=VECTOR('',#40332,0.15) ;
#10502=VECTOR('',#40339,0.15) ;
#10503=VECTOR('',#40346,0.15) ;
#10504=VECTOR('',#40353,0.15) ;
#10505=VECTOR('',#40360,0.15) ;
#10506=VECTOR('',#40367,0.15) ;
#10507=VECTOR('',#40376,0.55) ;
#10508=VECTOR('',#40377,0.55) ;
#10509=VECTOR('',#40384,0.25) ;
#10510=VECTOR('',#40393,0.15) ;
#11295=CIRCLE('',#31071,0.55) ;
#11296=CIRCLE('',#31072,0.55) ;
#11297=CIRCLE('',#31074,0.25) ;
#11298=CIRCLE('',#31075,0.25) ;
#11299=CIRCLE('',#31079,0.15) ;
#11300=CIRCLE('',#31082,0.8) ;
#11301=CIRCLE('',#31083,0.8) ;
#11302=CIRCLE('',#31085,1.1) ;
#11303=CIRCLE('',#31086,1.1) ;
#11304=CIRCLE('',#31091,0.8) ;
#11305=CIRCLE('',#31092,0.8) ;
#11306=CIRCLE('',#31094,1.1) ;
#11307=CIRCLE('',#31095,1.1) ;
#11308=CIRCLE('',#31098,0.0992156741649173) ;
#11309=CIRCLE('',#31100,0.139053721633041) ;
#11310=CIRCLE('',#31104,0.15) ;
#11311=CIRCLE('',#31106,0.15) ;
#11312=CIRCLE('',#31107,0.15) ;
#11313=CIRCLE('',#31109,0.15) ;
#11314=CIRCLE('',#31110,0.15) ;
#11315=CIRCLE('',#31111,0.15) ;
#11316=CIRCLE('',#31113,0.15) ;
#11317=CIRCLE('',#31114,0.15) ;
#11318=CIRCLE('',#31115,0.15) ;
#11319=CIRCLE('',#31117,0.15) ;
#11320=CIRCLE('',#31118,0.15) ;
#11321=CIRCLE('',#31119,0.149999999999999) ;
#11322=CIRCLE('',#31120,0.15) ;
#11323=CIRCLE('',#31121,0.15) ;
#11324=CIRCLE('',#31123,0.15) ;
#11325=CIRCLE('',#31124,0.15) ;
#11326=CIRCLE('',#31125,0.15) ;
#11327=CIRCLE('',#31127,0.15) ;
#11328=CIRCLE('',#31128,0.15) ;
#11329=CIRCLE('',#31129,0.15) ;
#11330=CIRCLE('',#31131,0.15) ;
#11331=CIRCLE('',#31132,0.15) ;
#11332=CIRCLE('',#31133,0.15) ;
#11333=CIRCLE('',#31135,0.15) ;
#11334=CIRCLE('',#31136,0.15) ;
#11335=CIRCLE('',#31137,0.149999999999999) ;
#11336=CIRCLE('',#31138,0.15) ;
#11337=CIRCLE('',#31139,0.15) ;
#11338=CIRCLE('',#31141,0.15) ;
#11339=CIRCLE('',#31142,0.15) ;
#11340=CIRCLE('',#31143,0.15) ;
#11341=CIRCLE('',#31145,0.15) ;
#11342=CIRCLE('',#31146,0.15) ;
#11343=CIRCLE('',#31147,0.15) ;
#11344=CIRCLE('',#31149,0.15) ;
#11345=CIRCLE('',#31150,0.15) ;
#11346=CIRCLE('',#31151,0.15) ;
#11347=CIRCLE('',#31153,0.15) ;
#11348=CIRCLE('',#31154,0.15) ;
#11349=CIRCLE('',#31155,0.149999999999999) ;
#11350=CIRCLE('',#31156,0.15) ;
#11351=CIRCLE('',#31157,0.15) ;
#11352=CIRCLE('',#31159,0.15) ;
#11353=CIRCLE('',#31160,0.15) ;
#11354=CIRCLE('',#31161,0.15) ;
#11355=CIRCLE('',#31163,0.15) ;
#11356=CIRCLE('',#31164,0.15) ;
#11357=CIRCLE('',#31165,0.15) ;
#11358=CIRCLE('',#31167,0.15) ;
#11359=CIRCLE('',#31168,0.15) ;
#11360=CIRCLE('',#31169,0.15) ;
#11361=CIRCLE('',#31171,0.15) ;
#11362=CIRCLE('',#31172,0.15) ;
#11363=CIRCLE('',#31173,0.149999999999999) ;
#11364=CIRCLE('',#31174,0.15) ;
#11365=CIRCLE('',#31175,0.15) ;
#11366=CIRCLE('',#31177,0.15) ;
#11367=CIRCLE('',#31178,0.15) ;
#11368=CIRCLE('',#31179,0.15) ;
#11369=CIRCLE('',#31181,0.15) ;
#11370=CIRCLE('',#31182,0.15) ;
#11371=CIRCLE('',#31183,0.15) ;
#11372=CIRCLE('',#31185,0.15) ;
#11373=CIRCLE('',#31186,0.15) ;
#11374=CIRCLE('',#31187,0.15) ;
#11375=CIRCLE('',#31189,0.15) ;
#11376=CIRCLE('',#31190,0.15) ;
#11377=CIRCLE('',#31191,0.149999999999999) ;
#11378=CIRCLE('',#31192,0.15) ;
#11379=CIRCLE('',#31193,0.15) ;
#11380=CIRCLE('',#31195,0.15) ;
#11381=CIRCLE('',#31196,0.15) ;
#11382=CIRCLE('',#31197,0.15) ;
#11383=CIRCLE('',#31199,0.15) ;
#11384=CIRCLE('',#31200,0.15) ;
#11385=CIRCLE('',#31201,0.15) ;
#11386=CIRCLE('',#31203,0.15) ;
#11387=CIRCLE('',#31204,0.15) ;
#11388=CIRCLE('',#31205,0.15) ;
#11389=CIRCLE('',#31207,0.15) ;
#11390=CIRCLE('',#31208,0.15) ;
#11391=CIRCLE('',#31209,0.149999999999999) ;
#11392=CIRCLE('',#31210,0.15) ;
#11393=CIRCLE('',#31211,0.15) ;
#11394=CIRCLE('',#31213,0.15) ;
#11395=CIRCLE('',#31214,0.15) ;
#11396=CIRCLE('',#31215,0.15) ;
#11397=CIRCLE('',#31217,0.15) ;
#11398=CIRCLE('',#31218,0.15) ;
#11399=CIRCLE('',#31219,0.15) ;
#11400=CIRCLE('',#31221,0.15) ;
#11401=CIRCLE('',#31222,0.15) ;
#11402=CIRCLE('',#31223,0.15) ;
#11403=CIRCLE('',#31225,0.15) ;
#11404=CIRCLE('',#31226,0.15) ;
#11405=CIRCLE('',#31227,0.149999999999999) ;
#11406=CIRCLE('',#31228,0.15) ;
#11407=CIRCLE('',#31229,0.15) ;
#11408=CIRCLE('',#31231,0.15) ;
#11409=CIRCLE('',#31232,0.15) ;
#11410=CIRCLE('',#31233,0.15) ;
#11411=CIRCLE('',#31235,0.15) ;
#11412=CIRCLE('',#31236,0.15) ;
#11413=CIRCLE('',#31237,0.15) ;
#11414=CIRCLE('',#31239,0.15) ;
#11415=CIRCLE('',#31240,0.15) ;
#11416=CIRCLE('',#31241,0.15) ;
#11417=CIRCLE('',#31243,0.15) ;
#11418=CIRCLE('',#31244,0.15) ;
#11419=CIRCLE('',#31245,0.149999999999999) ;
#11420=CIRCLE('',#31246,0.15) ;
#11421=CIRCLE('',#31247,0.15) ;
#11422=CIRCLE('',#31249,0.15) ;
#11423=CIRCLE('',#31250,0.15) ;
#11424=CIRCLE('',#31251,0.15) ;
#11425=CIRCLE('',#31253,0.15) ;
#11426=CIRCLE('',#31254,0.15) ;
#11427=CIRCLE('',#31255,0.15) ;
#11428=CIRCLE('',#31257,0.15) ;
#11429=CIRCLE('',#31258,0.15) ;
#11430=CIRCLE('',#31259,0.15) ;
#11431=CIRCLE('',#31261,0.15) ;
#11432=CIRCLE('',#31262,0.15) ;
#11433=CIRCLE('',#31263,0.149999999999999) ;
#11434=CIRCLE('',#31264,0.15) ;
#11435=CIRCLE('',#31265,0.15) ;
#11436=CIRCLE('',#31267,0.15) ;
#11437=CIRCLE('',#31268,0.15) ;
#11438=CIRCLE('',#31269,0.15) ;
#11439=CIRCLE('',#31271,0.15) ;
#11440=CIRCLE('',#31272,0.15) ;
#11441=CIRCLE('',#31273,0.15) ;
#11442=CIRCLE('',#31275,0.15) ;
#11443=CIRCLE('',#31276,0.15) ;
#11444=CIRCLE('',#31277,0.15) ;
#11445=CIRCLE('',#31279,0.15) ;
#11446=CIRCLE('',#31280,0.15) ;
#11447=CIRCLE('',#31281,0.149999999999999) ;
#11448=CIRCLE('',#31282,0.15) ;
#11449=CIRCLE('',#31283,0.15) ;
#11450=CIRCLE('',#31285,0.15) ;
#11451=CIRCLE('',#31286,0.15) ;
#11452=CIRCLE('',#31287,0.15) ;
#11453=CIRCLE('',#31289,0.15) ;
#11454=CIRCLE('',#31290,0.15) ;
#11455=CIRCLE('',#31291,0.15) ;
#11456=CIRCLE('',#31293,0.15) ;
#11457=CIRCLE('',#31294,0.15) ;
#11458=CIRCLE('',#31295,0.15) ;
#11459=CIRCLE('',#31297,0.15) ;
#11460=CIRCLE('',#31298,0.15) ;
#11461=CIRCLE('',#31299,0.149999999999999) ;
#11462=CIRCLE('',#31300,0.15) ;
#11463=CIRCLE('',#31301,0.15) ;
#11464=CIRCLE('',#31303,0.15) ;
#11465=CIRCLE('',#31304,0.15) ;
#11466=CIRCLE('',#31305,0.15) ;
#11467=CIRCLE('',#31307,0.15) ;
#11468=CIRCLE('',#31308,0.15) ;
#11469=CIRCLE('',#31309,0.15) ;
#11470=CIRCLE('',#31311,0.15) ;
#11471=CIRCLE('',#31312,0.15) ;
#11472=CIRCLE('',#31313,0.15) ;
#11473=CIRCLE('',#31315,0.15) ;
#11474=CIRCLE('',#31316,0.15) ;
#11475=CIRCLE('',#31317,0.149999999999999) ;
#11476=CIRCLE('',#31318,0.15) ;
#11477=CIRCLE('',#31319,0.15) ;
#11478=CIRCLE('',#31321,0.15) ;
#11479=CIRCLE('',#31322,0.15) ;
#11480=CIRCLE('',#31323,0.15) ;
#11481=CIRCLE('',#31325,0.15) ;
#11482=CIRCLE('',#31326,0.15) ;
#11483=CIRCLE('',#31327,0.15) ;
#11484=CIRCLE('',#31329,0.15) ;
#11485=CIRCLE('',#31330,0.15) ;
#11486=CIRCLE('',#31331,0.15) ;
#11487=CIRCLE('',#31333,0.15) ;
#11488=CIRCLE('',#31334,0.15) ;
#11489=CIRCLE('',#31335,0.149999999999999) ;
#11490=CIRCLE('',#31336,0.15) ;
#11491=CIRCLE('',#31337,0.15) ;
#11492=CIRCLE('',#31339,0.15) ;
#11493=CIRCLE('',#31340,0.15) ;
#11494=CIRCLE('',#31341,0.15) ;
#11495=CIRCLE('',#31343,0.15) ;
#11496=CIRCLE('',#31344,0.15) ;
#11497=CIRCLE('',#31345,0.15) ;
#11498=CIRCLE('',#31347,0.15) ;
#11499=CIRCLE('',#31348,0.15) ;
#11500=CIRCLE('',#31349,0.15) ;
#11501=CIRCLE('',#31351,0.15) ;
#11502=CIRCLE('',#31352,0.15) ;
#11503=CIRCLE('',#31353,0.149999999999999) ;
#11504=CIRCLE('',#31354,0.15) ;
#11505=CIRCLE('',#31355,0.15) ;
#11506=CIRCLE('',#31357,0.15) ;
#11507=CIRCLE('',#31358,0.15) ;
#11508=CIRCLE('',#31359,0.15) ;
#11509=CIRCLE('',#31361,0.15) ;
#11510=CIRCLE('',#31362,0.15) ;
#11511=CIRCLE('',#31363,0.15) ;
#11512=CIRCLE('',#31365,0.15) ;
#11513=CIRCLE('',#31366,0.15) ;
#11514=CIRCLE('',#31367,0.15) ;
#11515=CIRCLE('',#31369,0.15) ;
#11516=CIRCLE('',#31370,0.15) ;
#11517=CIRCLE('',#31371,0.149999999999999) ;
#11518=CIRCLE('',#31372,0.15) ;
#11519=CIRCLE('',#31373,0.15) ;
#11520=CIRCLE('',#31375,0.15) ;
#11521=CIRCLE('',#31376,0.15) ;
#11522=CIRCLE('',#31377,0.15) ;
#11523=CIRCLE('',#31379,0.15) ;
#11524=CIRCLE('',#31380,0.15) ;
#11525=CIRCLE('',#31381,0.15) ;
#11526=CIRCLE('',#31383,0.15) ;
#11527=CIRCLE('',#31384,0.15) ;
#11528=CIRCLE('',#31385,0.15) ;
#11529=CIRCLE('',#31387,0.15) ;
#11530=CIRCLE('',#31388,0.15) ;
#11531=CIRCLE('',#31389,0.149999999999999) ;
#11532=CIRCLE('',#31390,0.15) ;
#11533=CIRCLE('',#31391,0.15) ;
#11534=CIRCLE('',#31393,0.15) ;
#11535=CIRCLE('',#31394,0.15) ;
#11536=CIRCLE('',#31395,0.15) ;
#11537=CIRCLE('',#31397,0.15) ;
#11538=CIRCLE('',#31398,0.15) ;
#11539=CIRCLE('',#31399,0.15) ;
#11540=CIRCLE('',#31401,0.15) ;
#11541=CIRCLE('',#31402,0.15) ;
#11542=CIRCLE('',#31403,0.15) ;
#11543=CIRCLE('',#31405,0.15) ;
#11544=CIRCLE('',#31406,0.15) ;
#11545=CIRCLE('',#31407,0.149999999999999) ;
#11546=CIRCLE('',#31408,0.15) ;
#11547=CIRCLE('',#31409,0.15) ;
#11548=CIRCLE('',#31411,0.15) ;
#11549=CIRCLE('',#31412,0.15) ;
#11550=CIRCLE('',#31413,0.15) ;
#11551=CIRCLE('',#31415,0.15) ;
#11552=CIRCLE('',#31416,0.15) ;
#11553=CIRCLE('',#31417,0.15) ;
#11554=CIRCLE('',#31419,0.15) ;
#11555=CIRCLE('',#31420,0.15) ;
#11556=CIRCLE('',#31421,0.15) ;
#11557=CIRCLE('',#31423,0.15) ;
#11558=CIRCLE('',#31424,0.15) ;
#11559=CIRCLE('',#31425,0.149999999999999) ;
#11560=CIRCLE('',#31426,0.15) ;
#11561=CIRCLE('',#31427,0.15) ;
#11562=CIRCLE('',#31429,0.15) ;
#11563=CIRCLE('',#31430,0.15) ;
#11564=CIRCLE('',#31431,0.15) ;
#11565=CIRCLE('',#31433,0.15) ;
#11566=CIRCLE('',#31434,0.15) ;
#11567=CIRCLE('',#31435,0.15) ;
#11568=CIRCLE('',#31437,0.15) ;
#11569=CIRCLE('',#31438,0.15) ;
#11570=CIRCLE('',#31439,0.15) ;
#11571=CIRCLE('',#31441,0.15) ;
#11572=CIRCLE('',#31442,0.15) ;
#11573=CIRCLE('',#31443,0.149999999999999) ;
#11574=CIRCLE('',#31444,0.15) ;
#11575=CIRCLE('',#31445,0.15) ;
#11576=CIRCLE('',#31447,0.15) ;
#11577=CIRCLE('',#31448,0.15) ;
#11578=CIRCLE('',#31449,0.15) ;
#11579=CIRCLE('',#31451,0.15) ;
#11580=CIRCLE('',#31452,0.15) ;
#11581=CIRCLE('',#31453,0.15) ;
#11582=CIRCLE('',#31455,0.15) ;
#11583=CIRCLE('',#31456,0.15) ;
#11584=CIRCLE('',#31457,0.15) ;
#11585=CIRCLE('',#31459,0.15) ;
#11586=CIRCLE('',#31460,0.15) ;
#11587=CIRCLE('',#31461,0.149999999999999) ;
#11588=CIRCLE('',#31462,0.15) ;
#11589=CIRCLE('',#31463,0.15) ;
#11590=CIRCLE('',#31465,0.15) ;
#11591=CIRCLE('',#31466,0.15) ;
#11592=CIRCLE('',#31467,0.15) ;
#11593=CIRCLE('',#31469,0.15) ;
#11594=CIRCLE('',#31470,0.15) ;
#11595=CIRCLE('',#31471,0.15) ;
#11596=CIRCLE('',#31473,0.15) ;
#11597=CIRCLE('',#31474,0.15) ;
#11598=CIRCLE('',#31475,0.15) ;
#11599=CIRCLE('',#31477,0.15) ;
#11600=CIRCLE('',#31478,0.15) ;
#11601=CIRCLE('',#31479,0.149999999999999) ;
#11602=CIRCLE('',#31480,0.15) ;
#11603=CIRCLE('',#31481,0.15) ;
#11604=CIRCLE('',#31483,0.15) ;
#11605=CIRCLE('',#31484,0.15) ;
#11606=CIRCLE('',#31485,0.15) ;
#11607=CIRCLE('',#31487,0.15) ;
#11608=CIRCLE('',#31488,0.15) ;
#11609=CIRCLE('',#31489,0.15) ;
#11610=CIRCLE('',#31491,0.15) ;
#11611=CIRCLE('',#31492,0.15) ;
#11612=CIRCLE('',#31493,0.15) ;
#11613=CIRCLE('',#31495,0.15) ;
#11614=CIRCLE('',#31496,0.15) ;
#11615=CIRCLE('',#31497,0.149999999999999) ;
#11616=CIRCLE('',#31498,0.15) ;
#11617=CIRCLE('',#31499,0.15) ;
#11618=CIRCLE('',#31501,0.15) ;
#11619=CIRCLE('',#31502,0.15) ;
#11620=CIRCLE('',#31503,0.15) ;
#11621=CIRCLE('',#31505,0.15) ;
#11622=CIRCLE('',#31506,0.15) ;
#11623=CIRCLE('',#31507,0.15) ;
#11624=CIRCLE('',#31509,0.15) ;
#11625=CIRCLE('',#31510,0.15) ;
#11626=CIRCLE('',#31511,0.15) ;
#11627=CIRCLE('',#31513,0.15) ;
#11628=CIRCLE('',#31514,0.15) ;
#11629=CIRCLE('',#31515,0.149999999999999) ;
#11630=CIRCLE('',#31516,0.15) ;
#11631=CIRCLE('',#31517,0.15) ;
#11632=CIRCLE('',#31519,0.15) ;
#11633=CIRCLE('',#31520,0.15) ;
#11634=CIRCLE('',#31521,0.15) ;
#11635=CIRCLE('',#31523,0.15) ;
#11636=CIRCLE('',#31524,0.15) ;
#11637=CIRCLE('',#31525,0.15) ;
#11638=CIRCLE('',#31527,0.15) ;
#11639=CIRCLE('',#31528,0.15) ;
#11640=CIRCLE('',#31529,0.15) ;
#11641=CIRCLE('',#31531,0.15) ;
#11642=CIRCLE('',#31532,0.15) ;
#11643=CIRCLE('',#31533,0.149999999999999) ;
#11644=CIRCLE('',#31534,0.15) ;
#11645=CIRCLE('',#31535,0.15) ;
#11646=CIRCLE('',#31537,0.15) ;
#11647=CIRCLE('',#31538,0.15) ;
#11648=CIRCLE('',#31539,0.15) ;
#11649=CIRCLE('',#31541,0.15) ;
#11650=CIRCLE('',#31542,0.15) ;
#11651=CIRCLE('',#31543,0.15) ;
#11652=CIRCLE('',#31545,0.15) ;
#11653=CIRCLE('',#31546,0.15) ;
#11654=CIRCLE('',#31547,0.15) ;
#11655=CIRCLE('',#31549,0.15) ;
#11656=CIRCLE('',#31550,0.15) ;
#11657=CIRCLE('',#31551,0.149999999999999) ;
#11658=CIRCLE('',#31552,0.15) ;
#11659=CIRCLE('',#31553,0.15) ;
#11660=CIRCLE('',#31555,0.15) ;
#11661=CIRCLE('',#31556,0.15) ;
#11662=CIRCLE('',#31557,0.15) ;
#11663=CIRCLE('',#31559,0.15) ;
#11664=CIRCLE('',#31560,0.15) ;
#11665=CIRCLE('',#31561,0.15) ;
#11666=CIRCLE('',#31563,0.15) ;
#11667=CIRCLE('',#31564,0.15) ;
#11668=CIRCLE('',#31565,0.15) ;
#11669=CIRCLE('',#31567,0.15) ;
#11670=CIRCLE('',#31568,0.15) ;
#11671=CIRCLE('',#31569,0.149999999999999) ;
#11672=CIRCLE('',#31570,0.15) ;
#11673=CIRCLE('',#31571,0.15) ;
#11674=CIRCLE('',#31573,0.15) ;
#11675=CIRCLE('',#31574,0.15) ;
#11676=CIRCLE('',#31575,0.15) ;
#11677=CIRCLE('',#31577,0.15) ;
#11678=CIRCLE('',#31578,0.15) ;
#11679=CIRCLE('',#31579,0.15) ;
#11680=CIRCLE('',#31581,0.15) ;
#11681=CIRCLE('',#31582,0.15) ;
#11682=CIRCLE('',#31583,0.15) ;
#11683=CIRCLE('',#31585,0.15) ;
#11684=CIRCLE('',#31586,0.15) ;
#11685=CIRCLE('',#31587,0.149999999999999) ;
#11686=CIRCLE('',#31588,0.15) ;
#11687=CIRCLE('',#31589,0.15) ;
#11688=CIRCLE('',#31591,0.15) ;
#11689=CIRCLE('',#31592,0.15) ;
#11690=CIRCLE('',#31593,0.15) ;
#11691=CIRCLE('',#31595,0.15) ;
#11692=CIRCLE('',#31596,0.15) ;
#11693=CIRCLE('',#31597,0.15) ;
#11694=CIRCLE('',#31599,0.15) ;
#11695=CIRCLE('',#31600,0.15) ;
#11696=CIRCLE('',#31601,0.15) ;
#11697=CIRCLE('',#31603,0.15) ;
#11698=CIRCLE('',#31604,0.15) ;
#11699=CIRCLE('',#31605,0.149999999999999) ;
#11700=CIRCLE('',#31606,0.15) ;
#11701=CIRCLE('',#31607,0.15) ;
#11702=CIRCLE('',#31609,0.15) ;
#11703=CIRCLE('',#31610,0.15) ;
#11704=CIRCLE('',#31611,0.15) ;
#11705=CIRCLE('',#31613,0.15) ;
#11706=CIRCLE('',#31614,0.15) ;
#11707=CIRCLE('',#31615,0.15) ;
#11708=CIRCLE('',#31617,0.15) ;
#11709=CIRCLE('',#31618,0.15) ;
#11710=CIRCLE('',#31619,0.15) ;
#11711=CIRCLE('',#31621,0.15) ;
#11712=CIRCLE('',#31622,0.15) ;
#11713=CIRCLE('',#31623,0.149999999999999) ;
#11714=CIRCLE('',#31624,0.15) ;
#11715=CIRCLE('',#31625,0.15) ;
#11716=CIRCLE('',#31627,0.15) ;
#11717=CIRCLE('',#31628,0.15) ;
#11718=CIRCLE('',#31629,0.15) ;
#11719=CIRCLE('',#31631,0.15) ;
#11720=CIRCLE('',#31632,0.15) ;
#11721=CIRCLE('',#31633,0.15) ;
#11722=CIRCLE('',#31635,0.15) ;
#11723=CIRCLE('',#31636,0.15) ;
#11724=CIRCLE('',#31637,0.15) ;
#11725=CIRCLE('',#31639,0.15) ;
#11726=CIRCLE('',#31640,0.15) ;
#11727=CIRCLE('',#31641,0.149999999999999) ;
#11728=CIRCLE('',#31642,0.15) ;
#11729=CIRCLE('',#31643,0.15) ;
#11730=CIRCLE('',#31645,0.15) ;
#11731=CIRCLE('',#31646,0.15) ;
#11732=CIRCLE('',#31647,0.15) ;
#11733=CIRCLE('',#31649,0.15) ;
#11734=CIRCLE('',#31650,0.15) ;
#11735=CIRCLE('',#31651,0.15) ;
#11736=CIRCLE('',#31653,0.15) ;
#11737=CIRCLE('',#31654,0.15) ;
#11738=CIRCLE('',#31655,0.15) ;
#11739=CIRCLE('',#31657,0.15) ;
#11740=CIRCLE('',#31658,0.15) ;
#11741=CIRCLE('',#31659,0.149999999999999) ;
#11742=CIRCLE('',#31660,0.15) ;
#11743=CIRCLE('',#31661,0.15) ;
#11744=CIRCLE('',#31663,0.15) ;
#11745=CIRCLE('',#31664,0.15) ;
#11746=CIRCLE('',#31665,0.15) ;
#11747=CIRCLE('',#31667,0.15) ;
#11748=CIRCLE('',#31668,0.15) ;
#11749=CIRCLE('',#31669,0.15) ;
#11750=CIRCLE('',#31671,0.15) ;
#11751=CIRCLE('',#31672,0.15) ;
#11752=CIRCLE('',#31673,0.15) ;
#11753=CIRCLE('',#32054,0.15) ;
#11754=CIRCLE('',#32057,0.55) ;
#11755=CIRCLE('',#32058,0.55) ;
#11756=CIRCLE('',#32060,0.25) ;
#11757=CIRCLE('',#32061,0.25) ;
#11758=CIRCLE('',#32065,0.15) ;
#13753=VERTEX_POINT('',#47522) ;
#13754=VERTEX_POINT('',#47524) ;
#13755=VERTEX_POINT('',#47527) ;
#13756=VERTEX_POINT('',#47528) ;
#13757=VERTEX_POINT('',#47566) ;
#13758=VERTEX_POINT('',#47568) ;
#13759=VERTEX_POINT('',#47574) ;
#13760=VERTEX_POINT('',#47579) ;
#13761=VERTEX_POINT('',#47581) ;
#13762=VERTEX_POINT('',#47585) ;
#13763=VERTEX_POINT('',#47587) ;
#13764=VERTEX_POINT('',#47593) ;
#13765=VERTEX_POINT('',#47594) ;
#13766=VERTEX_POINT('',#47596) ;
#13767=VERTEX_POINT('',#47607) ;
#13768=VERTEX_POINT('',#47618) ;
#13769=VERTEX_POINT('',#47626) ;
#13770=VERTEX_POINT('',#47630) ;
#13771=VERTEX_POINT('',#47632) ;
#13772=VERTEX_POINT('',#47636) ;
#13773=VERTEX_POINT('',#47638) ;
#13774=VERTEX_POINT('',#47640) ;
#13775=VERTEX_POINT('',#47642) ;
#13776=VERTEX_POINT('',#47644) ;
#13777=VERTEX_POINT('',#47651) ;
#13778=VERTEX_POINT('',#47655) ;
#13779=VERTEX_POINT('',#47657) ;
#13780=VERTEX_POINT('',#47661) ;
#13781=VERTEX_POINT('',#47662) ;
#13782=VERTEX_POINT('',#47664) ;
#13783=VERTEX_POINT('',#47668) ;
#13784=VERTEX_POINT('',#47669) ;
#13785=VERTEX_POINT('',#47671) ;
#13786=VERTEX_POINT('',#47673) ;
#13787=VERTEX_POINT('',#47675) ;
#13788=VERTEX_POINT('',#47679) ;
#13789=VERTEX_POINT('',#47680) ;
#13790=VERTEX_POINT('',#47682) ;
#13791=VERTEX_POINT('',#47686) ;
#13792=VERTEX_POINT('',#47687) ;
#13793=VERTEX_POINT('',#47689) ;
#13794=VERTEX_POINT('',#47693) ;
#13795=VERTEX_POINT('',#47694) ;
#13796=VERTEX_POINT('',#47696) ;
#13797=VERTEX_POINT('',#47700) ;
#13798=VERTEX_POINT('',#47701) ;
#13799=VERTEX_POINT('',#47703) ;
#13800=VERTEX_POINT('',#47705) ;
#13801=VERTEX_POINT('',#47707) ;
#13802=VERTEX_POINT('',#47711) ;
#13803=VERTEX_POINT('',#47712) ;
#13804=VERTEX_POINT('',#47714) ;
#13805=VERTEX_POINT('',#47718) ;
#13806=VERTEX_POINT('',#47719) ;
#13807=VERTEX_POINT('',#47721) ;
#13808=VERTEX_POINT('',#47725) ;
#13809=VERTEX_POINT('',#47726) ;
#13810=VERTEX_POINT('',#47728) ;
#13811=VERTEX_POINT('',#47732) ;
#13812=VERTEX_POINT('',#47733) ;
#13813=VERTEX_POINT('',#47735) ;
#13814=VERTEX_POINT('',#47737) ;
#13815=VERTEX_POINT('',#47739) ;
#13816=VERTEX_POINT('',#47743) ;
#13817=VERTEX_POINT('',#47744) ;
#13818=VERTEX_POINT('',#47746) ;
#13819=VERTEX_POINT('',#47750) ;
#13820=VERTEX_POINT('',#47751) ;
#13821=VERTEX_POINT('',#47753) ;
#13822=VERTEX_POINT('',#47757) ;
#13823=VERTEX_POINT('',#47758) ;
#13824=VERTEX_POINT('',#47760) ;
#13825=VERTEX_POINT('',#47764) ;
#13826=VERTEX_POINT('',#47765) ;
#13827=VERTEX_POINT('',#47767) ;
#13828=VERTEX_POINT('',#47769) ;
#13829=VERTEX_POINT('',#47771) ;
#13830=VERTEX_POINT('',#47775) ;
#13831=VERTEX_POINT('',#47776) ;
#13832=VERTEX_POINT('',#47778) ;
#13833=VERTEX_POINT('',#47782) ;
#13834=VERTEX_POINT('',#47783) ;
#13835=VERTEX_POINT('',#47785) ;
#13836=VERTEX_POINT('',#47789) ;
#13837=VERTEX_POINT('',#47790) ;
#13838=VERTEX_POINT('',#47792) ;
#13839=VERTEX_POINT('',#47796) ;
#13840=VERTEX_POINT('',#47797) ;
#13841=VERTEX_POINT('',#47799) ;
#13842=VERTEX_POINT('',#47801) ;
#13843=VERTEX_POINT('',#47803) ;
#13844=VERTEX_POINT('',#47807) ;
#13845=VERTEX_POINT('',#47808) ;
#13846=VERTEX_POINT('',#47810) ;
#13847=VERTEX_POINT('',#47814) ;
#13848=VERTEX_POINT('',#47815) ;
#13849=VERTEX_POINT('',#47817) ;
#13850=VERTEX_POINT('',#47821) ;
#13851=VERTEX_POINT('',#47822) ;
#13852=VERTEX_POINT('',#47824) ;
#13853=VERTEX_POINT('',#47828) ;
#13854=VERTEX_POINT('',#47829) ;
#13855=VERTEX_POINT('',#47831) ;
#13856=VERTEX_POINT('',#47833) ;
#13857=VERTEX_POINT('',#47835) ;
#13858=VERTEX_POINT('',#47839) ;
#13859=VERTEX_POINT('',#47840) ;
#13860=VERTEX_POINT('',#47842) ;
#13861=VERTEX_POINT('',#47846) ;
#13862=VERTEX_POINT('',#47847) ;
#13863=VERTEX_POINT('',#47849) ;
#13864=VERTEX_POINT('',#47853) ;
#13865=VERTEX_POINT('',#47854) ;
#13866=VERTEX_POINT('',#47856) ;
#13867=VERTEX_POINT('',#47860) ;
#13868=VERTEX_POINT('',#47861) ;
#13869=VERTEX_POINT('',#47863) ;
#13870=VERTEX_POINT('',#47865) ;
#13871=VERTEX_POINT('',#47867) ;
#13872=VERTEX_POINT('',#47871) ;
#13873=VERTEX_POINT('',#47872) ;
#13874=VERTEX_POINT('',#47874) ;
#13875=VERTEX_POINT('',#47878) ;
#13876=VERTEX_POINT('',#47879) ;
#13877=VERTEX_POINT('',#47881) ;
#13878=VERTEX_POINT('',#47885) ;
#13879=VERTEX_POINT('',#47886) ;
#13880=VERTEX_POINT('',#47888) ;
#13881=VERTEX_POINT('',#47892) ;
#13882=VERTEX_POINT('',#47893) ;
#13883=VERTEX_POINT('',#47895) ;
#13884=VERTEX_POINT('',#47897) ;
#13885=VERTEX_POINT('',#47899) ;
#13886=VERTEX_POINT('',#47903) ;
#13887=VERTEX_POINT('',#47904) ;
#13888=VERTEX_POINT('',#47906) ;
#13889=VERTEX_POINT('',#47910) ;
#13890=VERTEX_POINT('',#47911) ;
#13891=VERTEX_POINT('',#47913) ;
#13892=VERTEX_POINT('',#47917) ;
#13893=VERTEX_POINT('',#47918) ;
#13894=VERTEX_POINT('',#47920) ;
#13895=VERTEX_POINT('',#47924) ;
#13896=VERTEX_POINT('',#47925) ;
#13897=VERTEX_POINT('',#47927) ;
#13898=VERTEX_POINT('',#47929) ;
#13899=VERTEX_POINT('',#47931) ;
#13900=VERTEX_POINT('',#47935) ;
#13901=VERTEX_POINT('',#47936) ;
#13902=VERTEX_POINT('',#47938) ;
#13903=VERTEX_POINT('',#47942) ;
#13904=VERTEX_POINT('',#47943) ;
#13905=VERTEX_POINT('',#47945) ;
#13906=VERTEX_POINT('',#47949) ;
#13907=VERTEX_POINT('',#47950) ;
#13908=VERTEX_POINT('',#47952) ;
#13909=VERTEX_POINT('',#47956) ;
#13910=VERTEX_POINT('',#47957) ;
#13911=VERTEX_POINT('',#47959) ;
#13912=VERTEX_POINT('',#47961) ;
#13913=VERTEX_POINT('',#47963) ;
#13914=VERTEX_POINT('',#47967) ;
#13915=VERTEX_POINT('',#47968) ;
#13916=VERTEX_POINT('',#47970) ;
#13917=VERTEX_POINT('',#47974) ;
#13918=VERTEX_POINT('',#47975) ;
#13919=VERTEX_POINT('',#47977) ;
#13920=VERTEX_POINT('',#47981) ;
#13921=VERTEX_POINT('',#47982) ;
#13922=VERTEX_POINT('',#47984) ;
#13923=VERTEX_POINT('',#47988) ;
#13924=VERTEX_POINT('',#47989) ;
#13925=VERTEX_POINT('',#47991) ;
#13926=VERTEX_POINT('',#47993) ;
#13927=VERTEX_POINT('',#47995) ;
#13928=VERTEX_POINT('',#47999) ;
#13929=VERTEX_POINT('',#48000) ;
#13930=VERTEX_POINT('',#48002) ;
#13931=VERTEX_POINT('',#48006) ;
#13932=VERTEX_POINT('',#48007) ;
#13933=VERTEX_POINT('',#48009) ;
#13934=VERTEX_POINT('',#48013) ;
#13935=VERTEX_POINT('',#48014) ;
#13936=VERTEX_POINT('',#48016) ;
#13937=VERTEX_POINT('',#48020) ;
#13938=VERTEX_POINT('',#48021) ;
#13939=VERTEX_POINT('',#48023) ;
#13940=VERTEX_POINT('',#48025) ;
#13941=VERTEX_POINT('',#48027) ;
#13942=VERTEX_POINT('',#48031) ;
#13943=VERTEX_POINT('',#48032) ;
#13944=VERTEX_POINT('',#48034) ;
#13945=VERTEX_POINT('',#48038) ;
#13946=VERTEX_POINT('',#48039) ;
#13947=VERTEX_POINT('',#48041) ;
#13948=VERTEX_POINT('',#48045) ;
#13949=VERTEX_POINT('',#48046) ;
#13950=VERTEX_POINT('',#48048) ;
#13951=VERTEX_POINT('',#48052) ;
#13952=VERTEX_POINT('',#48053) ;
#13953=VERTEX_POINT('',#48055) ;
#13954=VERTEX_POINT('',#48057) ;
#13955=VERTEX_POINT('',#48059) ;
#13956=VERTEX_POINT('',#48063) ;
#13957=VERTEX_POINT('',#48064) ;
#13958=VERTEX_POINT('',#48066) ;
#13959=VERTEX_POINT('',#48070) ;
#13960=VERTEX_POINT('',#48071) ;
#13961=VERTEX_POINT('',#48073) ;
#13962=VERTEX_POINT('',#48077) ;
#13963=VERTEX_POINT('',#48078) ;
#13964=VERTEX_POINT('',#48080) ;
#13965=VERTEX_POINT('',#48084) ;
#13966=VERTEX_POINT('',#48085) ;
#13967=VERTEX_POINT('',#48087) ;
#13968=VERTEX_POINT('',#48089) ;
#13969=VERTEX_POINT('',#48091) ;
#13970=VERTEX_POINT('',#48095) ;
#13971=VERTEX_POINT('',#48096) ;
#13972=VERTEX_POINT('',#48098) ;
#13973=VERTEX_POINT('',#48102) ;
#13974=VERTEX_POINT('',#48103) ;
#13975=VERTEX_POINT('',#48105) ;
#13976=VERTEX_POINT('',#48109) ;
#13977=VERTEX_POINT('',#48110) ;
#13978=VERTEX_POINT('',#48112) ;
#13979=VERTEX_POINT('',#48116) ;
#13980=VERTEX_POINT('',#48117) ;
#13981=VERTEX_POINT('',#48119) ;
#13982=VERTEX_POINT('',#48121) ;
#13983=VERTEX_POINT('',#48123) ;
#13984=VERTEX_POINT('',#48127) ;
#13985=VERTEX_POINT('',#48128) ;
#13986=VERTEX_POINT('',#48130) ;
#13987=VERTEX_POINT('',#48134) ;
#13988=VERTEX_POINT('',#48135) ;
#13989=VERTEX_POINT('',#48137) ;
#13990=VERTEX_POINT('',#48141) ;
#13991=VERTEX_POINT('',#48142) ;
#13992=VERTEX_POINT('',#48144) ;
#13993=VERTEX_POINT('',#48148) ;
#13994=VERTEX_POINT('',#48149) ;
#13995=VERTEX_POINT('',#48151) ;
#13996=VERTEX_POINT('',#48153) ;
#13997=VERTEX_POINT('',#48155) ;
#13998=VERTEX_POINT('',#48159) ;
#13999=VERTEX_POINT('',#48160) ;
#14000=VERTEX_POINT('',#48162) ;
#14001=VERTEX_POINT('',#48166) ;
#14002=VERTEX_POINT('',#48167) ;
#14003=VERTEX_POINT('',#48169) ;
#14004=VERTEX_POINT('',#48173) ;
#14005=VERTEX_POINT('',#48174) ;
#14006=VERTEX_POINT('',#48176) ;
#14007=VERTEX_POINT('',#48180) ;
#14008=VERTEX_POINT('',#48181) ;
#14009=VERTEX_POINT('',#48183) ;
#14010=VERTEX_POINT('',#48185) ;
#14011=VERTEX_POINT('',#48187) ;
#14012=VERTEX_POINT('',#48191) ;
#14013=VERTEX_POINT('',#48192) ;
#14014=VERTEX_POINT('',#48194) ;
#14015=VERTEX_POINT('',#48198) ;
#14016=VERTEX_POINT('',#48199) ;
#14017=VERTEX_POINT('',#48201) ;
#14018=VERTEX_POINT('',#48205) ;
#14019=VERTEX_POINT('',#48206) ;
#14020=VERTEX_POINT('',#48208) ;
#14021=VERTEX_POINT('',#48212) ;
#14022=VERTEX_POINT('',#48213) ;
#14023=VERTEX_POINT('',#48215) ;
#14024=VERTEX_POINT('',#48217) ;
#14025=VERTEX_POINT('',#48219) ;
#14026=VERTEX_POINT('',#48223) ;
#14027=VERTEX_POINT('',#48224) ;
#14028=VERTEX_POINT('',#48226) ;
#14029=VERTEX_POINT('',#48230) ;
#14030=VERTEX_POINT('',#48231) ;
#14031=VERTEX_POINT('',#48233) ;
#14032=VERTEX_POINT('',#48237) ;
#14033=VERTEX_POINT('',#48238) ;
#14034=VERTEX_POINT('',#48240) ;
#14035=VERTEX_POINT('',#48244) ;
#14036=VERTEX_POINT('',#48245) ;
#14037=VERTEX_POINT('',#48247) ;
#14038=VERTEX_POINT('',#48249) ;
#14039=VERTEX_POINT('',#48251) ;
#14040=VERTEX_POINT('',#48255) ;
#14041=VERTEX_POINT('',#48256) ;
#14042=VERTEX_POINT('',#48258) ;
#14043=VERTEX_POINT('',#48262) ;
#14044=VERTEX_POINT('',#48263) ;
#14045=VERTEX_POINT('',#48265) ;
#14046=VERTEX_POINT('',#48269) ;
#14047=VERTEX_POINT('',#48270) ;
#14048=VERTEX_POINT('',#48272) ;
#14049=VERTEX_POINT('',#48276) ;
#14050=VERTEX_POINT('',#48277) ;
#14051=VERTEX_POINT('',#48279) ;
#14052=VERTEX_POINT('',#48281) ;
#14053=VERTEX_POINT('',#48283) ;
#14054=VERTEX_POINT('',#48287) ;
#14055=VERTEX_POINT('',#48288) ;
#14056=VERTEX_POINT('',#48290) ;
#14057=VERTEX_POINT('',#48294) ;
#14058=VERTEX_POINT('',#48295) ;
#14059=VERTEX_POINT('',#48297) ;
#14060=VERTEX_POINT('',#48301) ;
#14061=VERTEX_POINT('',#48302) ;
#14062=VERTEX_POINT('',#48304) ;
#14063=VERTEX_POINT('',#48308) ;
#14064=VERTEX_POINT('',#48309) ;
#14065=VERTEX_POINT('',#48311) ;
#14066=VERTEX_POINT('',#48313) ;
#14067=VERTEX_POINT('',#48315) ;
#14068=VERTEX_POINT('',#48319) ;
#14069=VERTEX_POINT('',#48320) ;
#14070=VERTEX_POINT('',#48322) ;
#14071=VERTEX_POINT('',#48326) ;
#14072=VERTEX_POINT('',#48327) ;
#14073=VERTEX_POINT('',#48329) ;
#14074=VERTEX_POINT('',#48333) ;
#14075=VERTEX_POINT('',#48334) ;
#14076=VERTEX_POINT('',#48336) ;
#14077=VERTEX_POINT('',#48340) ;
#14078=VERTEX_POINT('',#48341) ;
#14079=VERTEX_POINT('',#48343) ;
#14080=VERTEX_POINT('',#48345) ;
#14081=VERTEX_POINT('',#48347) ;
#14082=VERTEX_POINT('',#48351) ;
#14083=VERTEX_POINT('',#48352) ;
#14084=VERTEX_POINT('',#48354) ;
#14085=VERTEX_POINT('',#48358) ;
#14086=VERTEX_POINT('',#48359) ;
#14087=VERTEX_POINT('',#48361) ;
#14088=VERTEX_POINT('',#48365) ;
#14089=VERTEX_POINT('',#48366) ;
#14090=VERTEX_POINT('',#48368) ;
#14091=VERTEX_POINT('',#48372) ;
#14092=VERTEX_POINT('',#48373) ;
#14093=VERTEX_POINT('',#48375) ;
#14094=VERTEX_POINT('',#48377) ;
#14095=VERTEX_POINT('',#48379) ;
#14096=VERTEX_POINT('',#48383) ;
#14097=VERTEX_POINT('',#48384) ;
#14098=VERTEX_POINT('',#48386) ;
#14099=VERTEX_POINT('',#48390) ;
#14100=VERTEX_POINT('',#48391) ;
#14101=VERTEX_POINT('',#48393) ;
#14102=VERTEX_POINT('',#48397) ;
#14103=VERTEX_POINT('',#48398) ;
#14104=VERTEX_POINT('',#48400) ;
#14105=VERTEX_POINT('',#48404) ;
#14106=VERTEX_POINT('',#48405) ;
#14107=VERTEX_POINT('',#48407) ;
#14108=VERTEX_POINT('',#48409) ;
#14109=VERTEX_POINT('',#48411) ;
#14110=VERTEX_POINT('',#48415) ;
#14111=VERTEX_POINT('',#48416) ;
#14112=VERTEX_POINT('',#48418) ;
#14113=VERTEX_POINT('',#48422) ;
#14114=VERTEX_POINT('',#48423) ;
#14115=VERTEX_POINT('',#48425) ;
#14116=VERTEX_POINT('',#48429) ;
#14117=VERTEX_POINT('',#48430) ;
#14118=VERTEX_POINT('',#48432) ;
#14119=VERTEX_POINT('',#48436) ;
#14120=VERTEX_POINT('',#48437) ;
#14121=VERTEX_POINT('',#48439) ;
#14122=VERTEX_POINT('',#48441) ;
#14123=VERTEX_POINT('',#48443) ;
#14124=VERTEX_POINT('',#48447) ;
#14125=VERTEX_POINT('',#48448) ;
#14126=VERTEX_POINT('',#48450) ;
#14127=VERTEX_POINT('',#48454) ;
#14128=VERTEX_POINT('',#48455) ;
#14129=VERTEX_POINT('',#48457) ;
#14130=VERTEX_POINT('',#48461) ;
#14131=VERTEX_POINT('',#48462) ;
#14132=VERTEX_POINT('',#48464) ;
#14133=VERTEX_POINT('',#48468) ;
#14134=VERTEX_POINT('',#48469) ;
#14135=VERTEX_POINT('',#48471) ;
#14136=VERTEX_POINT('',#48473) ;
#14137=VERTEX_POINT('',#48475) ;
#14138=VERTEX_POINT('',#48479) ;
#14139=VERTEX_POINT('',#48480) ;
#14140=VERTEX_POINT('',#48482) ;
#14141=VERTEX_POINT('',#48486) ;
#14142=VERTEX_POINT('',#48487) ;
#14143=VERTEX_POINT('',#48489) ;
#14144=VERTEX_POINT('',#48493) ;
#14145=VERTEX_POINT('',#48494) ;
#14146=VERTEX_POINT('',#48496) ;
#14147=VERTEX_POINT('',#48500) ;
#14148=VERTEX_POINT('',#48501) ;
#14149=VERTEX_POINT('',#48503) ;
#14150=VERTEX_POINT('',#48505) ;
#14151=VERTEX_POINT('',#48507) ;
#14152=VERTEX_POINT('',#48511) ;
#14153=VERTEX_POINT('',#48512) ;
#14154=VERTEX_POINT('',#48514) ;
#14155=VERTEX_POINT('',#48518) ;
#14156=VERTEX_POINT('',#48519) ;
#14157=VERTEX_POINT('',#48521) ;
#14158=VERTEX_POINT('',#48525) ;
#14159=VERTEX_POINT('',#48526) ;
#14160=VERTEX_POINT('',#48528) ;
#14161=VERTEX_POINT('',#48532) ;
#14162=VERTEX_POINT('',#48533) ;
#14163=VERTEX_POINT('',#48535) ;
#14164=VERTEX_POINT('',#48537) ;
#14165=VERTEX_POINT('',#48539) ;
#14166=VERTEX_POINT('',#48543) ;
#14167=VERTEX_POINT('',#48544) ;
#14168=VERTEX_POINT('',#48546) ;
#14169=VERTEX_POINT('',#48550) ;
#14170=VERTEX_POINT('',#48551) ;
#14171=VERTEX_POINT('',#48553) ;
#14172=VERTEX_POINT('',#48557) ;
#14173=VERTEX_POINT('',#48558) ;
#14174=VERTEX_POINT('',#48560) ;
#14175=VERTEX_POINT('',#48564) ;
#14176=VERTEX_POINT('',#48565) ;
#14177=VERTEX_POINT('',#48567) ;
#14178=VERTEX_POINT('',#48569) ;
#14179=VERTEX_POINT('',#48571) ;
#14180=VERTEX_POINT('',#48575) ;
#14181=VERTEX_POINT('',#48576) ;
#14182=VERTEX_POINT('',#48578) ;
#14183=VERTEX_POINT('',#48582) ;
#14184=VERTEX_POINT('',#48583) ;
#14185=VERTEX_POINT('',#48585) ;
#14186=VERTEX_POINT('',#48589) ;
#14187=VERTEX_POINT('',#48590) ;
#14188=VERTEX_POINT('',#48592) ;
#14189=VERTEX_POINT('',#48596) ;
#14190=VERTEX_POINT('',#48597) ;
#14191=VERTEX_POINT('',#48599) ;
#14192=VERTEX_POINT('',#48601) ;
#14193=VERTEX_POINT('',#48603) ;
#14194=VERTEX_POINT('',#48607) ;
#14195=VERTEX_POINT('',#48608) ;
#14196=VERTEX_POINT('',#48610) ;
#14197=VERTEX_POINT('',#48614) ;
#14198=VERTEX_POINT('',#48615) ;
#14199=VERTEX_POINT('',#48617) ;
#14200=VERTEX_POINT('',#48621) ;
#14201=VERTEX_POINT('',#48622) ;
#14202=VERTEX_POINT('',#48624) ;
#14203=VERTEX_POINT('',#48628) ;
#14204=VERTEX_POINT('',#48629) ;
#14205=VERTEX_POINT('',#48631) ;
#14206=VERTEX_POINT('',#48633) ;
#14207=VERTEX_POINT('',#48635) ;
#14208=VERTEX_POINT('',#48639) ;
#14209=VERTEX_POINT('',#48640) ;
#14210=VERTEX_POINT('',#48642) ;
#14211=VERTEX_POINT('',#48646) ;
#14212=VERTEX_POINT('',#48647) ;
#14213=VERTEX_POINT('',#48649) ;
#14214=VERTEX_POINT('',#48653) ;
#14215=VERTEX_POINT('',#48654) ;
#14216=VERTEX_POINT('',#48656) ;
#14217=VERTEX_POINT('',#48664) ;
#14218=VERTEX_POINT('',#48669) ;
#14219=VERTEX_POINT('',#48674) ;
#14220=VERTEX_POINT('',#48679) ;
#14221=VERTEX_POINT('',#48684) ;
#14222=VERTEX_POINT('',#48689) ;
#14223=VERTEX_POINT('',#48694) ;
#14224=VERTEX_POINT('',#48699) ;
#14225=VERTEX_POINT('',#48704) ;
#14226=VERTEX_POINT('',#48709) ;
#14227=VERTEX_POINT('',#48714) ;
#14228=VERTEX_POINT('',#48719) ;
#14229=VERTEX_POINT('',#48724) ;
#14230=VERTEX_POINT('',#48729) ;
#14231=VERTEX_POINT('',#48734) ;
#14232=VERTEX_POINT('',#48739) ;
#14233=VERTEX_POINT('',#48744) ;
#14234=VERTEX_POINT('',#48749) ;
#14235=VERTEX_POINT('',#48754) ;
#14236=VERTEX_POINT('',#48759) ;
#14237=VERTEX_POINT('',#48764) ;
#14238=VERTEX_POINT('',#48769) ;
#14239=VERTEX_POINT('',#48774) ;
#14240=VERTEX_POINT('',#48779) ;
#14241=VERTEX_POINT('',#48784) ;
#14242=VERTEX_POINT('',#48789) ;
#14243=VERTEX_POINT('',#48794) ;
#14244=VERTEX_POINT('',#48799) ;
#14245=VERTEX_POINT('',#48804) ;
#14246=VERTEX_POINT('',#48809) ;
#14247=VERTEX_POINT('',#48814) ;
#14248=VERTEX_POINT('',#48819) ;
#14249=VERTEX_POINT('',#48824) ;
#14250=VERTEX_POINT('',#48829) ;
#14251=VERTEX_POINT('',#48834) ;
#14252=VERTEX_POINT('',#48839) ;
#14253=VERTEX_POINT('',#48844) ;
#14254=VERTEX_POINT('',#48849) ;
#14255=VERTEX_POINT('',#48854) ;
#14256=VERTEX_POINT('',#48859) ;
#14257=VERTEX_POINT('',#48864) ;
#14258=VERTEX_POINT('',#48869) ;
#14259=VERTEX_POINT('',#48874) ;
#14260=VERTEX_POINT('',#48879) ;
#14261=VERTEX_POINT('',#48884) ;
#14262=VERTEX_POINT('',#48889) ;
#14263=VERTEX_POINT('',#48894) ;
#14264=VERTEX_POINT('',#48899) ;
#14265=VERTEX_POINT('',#48904) ;
#14266=VERTEX_POINT('',#48909) ;
#14267=VERTEX_POINT('',#48914) ;
#14268=VERTEX_POINT('',#48919) ;
#14269=VERTEX_POINT('',#48924) ;
#14270=VERTEX_POINT('',#48929) ;
#14271=VERTEX_POINT('',#48934) ;
#14272=VERTEX_POINT('',#48939) ;
#14273=VERTEX_POINT('',#48944) ;
#14274=VERTEX_POINT('',#48949) ;
#14275=VERTEX_POINT('',#48954) ;
#14276=VERTEX_POINT('',#48959) ;
#14277=VERTEX_POINT('',#48964) ;
#14278=VERTEX_POINT('',#48969) ;
#14279=VERTEX_POINT('',#48974) ;
#14280=VERTEX_POINT('',#48979) ;
#14281=VERTEX_POINT('',#48984) ;
#14282=VERTEX_POINT('',#48989) ;
#14283=VERTEX_POINT('',#48994) ;
#14284=VERTEX_POINT('',#48999) ;
#14285=VERTEX_POINT('',#49004) ;
#14286=VERTEX_POINT('',#49009) ;
#14287=VERTEX_POINT('',#49014) ;
#14288=VERTEX_POINT('',#49019) ;
#14289=VERTEX_POINT('',#49024) ;
#14290=VERTEX_POINT('',#49029) ;
#14291=VERTEX_POINT('',#49034) ;
#14292=VERTEX_POINT('',#49039) ;
#14293=VERTEX_POINT('',#49044) ;
#14294=VERTEX_POINT('',#49049) ;
#14295=VERTEX_POINT('',#49054) ;
#14296=VERTEX_POINT('',#49059) ;
#14297=VERTEX_POINT('',#49064) ;
#14298=VERTEX_POINT('',#49069) ;
#14299=VERTEX_POINT('',#49074) ;
#14300=VERTEX_POINT('',#49079) ;
#14301=VERTEX_POINT('',#49084) ;
#14302=VERTEX_POINT('',#49089) ;
#14303=VERTEX_POINT('',#49094) ;
#14304=VERTEX_POINT('',#49099) ;
#14305=VERTEX_POINT('',#49104) ;
#14306=VERTEX_POINT('',#49109) ;
#14307=VERTEX_POINT('',#49114) ;
#14308=VERTEX_POINT('',#49119) ;
#14309=VERTEX_POINT('',#49124) ;
#14310=VERTEX_POINT('',#49129) ;
#14311=VERTEX_POINT('',#49134) ;
#14312=VERTEX_POINT('',#49139) ;
#14313=VERTEX_POINT('',#49144) ;
#14314=VERTEX_POINT('',#49149) ;
#14315=VERTEX_POINT('',#49154) ;
#14316=VERTEX_POINT('',#49159) ;
#14317=VERTEX_POINT('',#49164) ;
#14318=VERTEX_POINT('',#49169) ;
#14319=VERTEX_POINT('',#49174) ;
#14320=VERTEX_POINT('',#49179) ;
#14321=VERTEX_POINT('',#49184) ;
#14322=VERTEX_POINT('',#49189) ;
#14323=VERTEX_POINT('',#49194) ;
#14324=VERTEX_POINT('',#49199) ;
#14325=VERTEX_POINT('',#49204) ;
#14326=VERTEX_POINT('',#49209) ;
#14327=VERTEX_POINT('',#49214) ;
#14328=VERTEX_POINT('',#49219) ;
#14329=VERTEX_POINT('',#49224) ;
#14330=VERTEX_POINT('',#49229) ;
#14331=VERTEX_POINT('',#49234) ;
#14332=VERTEX_POINT('',#49239) ;
#14333=VERTEX_POINT('',#49244) ;
#14334=VERTEX_POINT('',#49249) ;
#14335=VERTEX_POINT('',#49254) ;
#14336=VERTEX_POINT('',#49259) ;
#14337=VERTEX_POINT('',#49264) ;
#14338=VERTEX_POINT('',#49269) ;
#14339=VERTEX_POINT('',#49274) ;
#14340=VERTEX_POINT('',#49279) ;
#14341=VERTEX_POINT('',#49284) ;
#14342=VERTEX_POINT('',#49289) ;
#14343=VERTEX_POINT('',#49294) ;
#14344=VERTEX_POINT('',#49296) ;
#14345=VERTEX_POINT('',#49298) ;
#14346=VERTEX_POINT('',#49317) ;
#14347=VERTEX_POINT('',#49320) ;
#14348=VERTEX_POINT('',#49342) ;
#14349=VERTEX_POINT('',#49344) ;
#14350=VERTEX_POINT('',#49350) ;
#17413=EDGE_CURVE('',#13753,#13753,#11295,.T.) ;
#17414=EDGE_CURVE('',#13753,#13754,#7901,.T.) ;
#17415=EDGE_CURVE('',#13754,#13754,#11296,.T.) ;
#17416=EDGE_CURVE('',#13755,#13756,#28,.T.) ;
#17417=EDGE_CURVE('',#13756,#13755,#29,.T.) ;
#17418=EDGE_CURVE('',#13757,#13757,#11297,.T.) ;
#17419=EDGE_CURVE('',#13757,#13758,#7902,.T.) ;
#17420=EDGE_CURVE('',#13758,#13758,#11298,.T.) ;
#17421=EDGE_CURVE('',#13759,#13759,#11299,.T.) ;
#17422=EDGE_CURVE('',#13759,#13756,#7903,.T.) ;
#17423=EDGE_CURVE('',#13760,#13760,#11300,.T.) ;
#17424=EDGE_CURVE('',#13760,#13761,#7904,.T.) ;
#17425=EDGE_CURVE('',#13761,#13761,#11301,.T.) ;
#17426=EDGE_CURVE('',#13762,#13762,#11302,.T.) ;
#17427=EDGE_CURVE('',#13762,#13763,#7905,.T.) ;
#17428=EDGE_CURVE('',#13763,#13763,#11303,.T.) ;
#17429=EDGE_CURVE('',#13764,#13765,#417,.T.) ;
#17430=EDGE_CURVE('',#13766,#13764,#30,.T.) ;
#17431=EDGE_CURVE('',#13767,#13766,#31,.T.) ;
#17432=EDGE_CURVE('',#13768,#13767,#32,.T.) ;
#17433=EDGE_CURVE('',#13765,#13768,#11304,.T.) ;
#17434=EDGE_CURVE('',#13765,#13769,#7906,.T.) ;
#17435=EDGE_CURVE('',#13769,#13769,#11305,.T.) ;
#17436=EDGE_CURVE('',#13770,#13770,#11306,.T.) ;
#17437=EDGE_CURVE('',#13770,#13771,#7907,.T.) ;
#17438=EDGE_CURVE('',#13771,#13771,#11307,.T.) ;
#17439=EDGE_CURVE('',#13765,#13772,#7908,.T.) ;
#17440=EDGE_CURVE('',#13773,#13768,#418,.T.) ;
#17441=EDGE_CURVE('',#13774,#13773,#11308,.T.) ;
#17442=EDGE_CURVE('',#13775,#13774,#419,.T.) ;
#17443=EDGE_CURVE('',#13776,#13775,#11309,.T.) ;
#17444=EDGE_CURVE('',#13772,#13776,#420,.T.) ;
#17445=EDGE_CURVE('',#13772,#13764,#11310,.T.) ;
#17446=EDGE_CURVE('',#13775,#13777,#11311,.T.) ;
#17447=EDGE_CURVE('',#13777,#13776,#11312,.T.) ;
#17448=EDGE_CURVE('',#13773,#13778,#11313,.T.) ;
#17449=EDGE_CURVE('',#13778,#13779,#11314,.T.) ;
#17450=EDGE_CURVE('',#13779,#13774,#11315,.T.) ;
#17451=EDGE_CURVE('',#13780,#13781,#11316,.T.) ;
#17452=EDGE_CURVE('',#13781,#13782,#11317,.T.) ;
#17453=EDGE_CURVE('',#13782,#13780,#11318,.T.) ;
#17454=EDGE_CURVE('',#13783,#13784,#11319,.T.) ;
#17455=EDGE_CURVE('',#13784,#13785,#11320,.T.) ;
#17456=EDGE_CURVE('',#13785,#13786,#11321,.T.) ;
#17457=EDGE_CURVE('',#13785,#13787,#11322,.T.) ;
#17458=EDGE_CURVE('',#13787,#13783,#11323,.T.) ;
#17459=EDGE_CURVE('',#13788,#13789,#11324,.T.) ;
#17460=EDGE_CURVE('',#13789,#13790,#11325,.T.) ;
#17461=EDGE_CURVE('',#13790,#13788,#11326,.T.) ;
#17462=EDGE_CURVE('',#13791,#13792,#11327,.T.) ;
#17463=EDGE_CURVE('',#13792,#13793,#11328,.T.) ;
#17464=EDGE_CURVE('',#13793,#13791,#11329,.T.) ;
#17465=EDGE_CURVE('',#13794,#13795,#11330,.T.) ;
#17466=EDGE_CURVE('',#13795,#13796,#11331,.T.) ;
#17467=EDGE_CURVE('',#13796,#13794,#11332,.T.) ;
#17468=EDGE_CURVE('',#13797,#13798,#11333,.T.) ;
#17469=EDGE_CURVE('',#13798,#13799,#11334,.T.) ;
#17470=EDGE_CURVE('',#13800,#13799,#11335,.T.) ;
#17471=EDGE_CURVE('',#13799,#13801,#11336,.T.) ;
#17472=EDGE_CURVE('',#13801,#13797,#11337,.T.) ;
#17473=EDGE_CURVE('',#13802,#13803,#11338,.T.) ;
#17474=EDGE_CURVE('',#13803,#13804,#11339,.T.) ;
#17475=EDGE_CURVE('',#13804,#13802,#11340,.T.) ;
#17476=EDGE_CURVE('',#13805,#13806,#11341,.T.) ;
#17477=EDGE_CURVE('',#13806,#13807,#11342,.T.) ;
#17478=EDGE_CURVE('',#13807,#13805,#11343,.T.) ;
#17479=EDGE_CURVE('',#13808,#13809,#11344,.T.) ;
#17480=EDGE_CURVE('',#13809,#13810,#11345,.T.) ;
#17481=EDGE_CURVE('',#13810,#13808,#11346,.T.) ;
#17482=EDGE_CURVE('',#13811,#13812,#11347,.T.) ;
#17483=EDGE_CURVE('',#13812,#13813,#11348,.T.) ;
#17484=EDGE_CURVE('',#13813,#13814,#11349,.T.) ;
#17485=EDGE_CURVE('',#13813,#13815,#11350,.T.) ;
#17486=EDGE_CURVE('',#13815,#13811,#11351,.T.) ;
#17487=EDGE_CURVE('',#13816,#13817,#11352,.T.) ;
#17488=EDGE_CURVE('',#13817,#13818,#11353,.T.) ;
#17489=EDGE_CURVE('',#13818,#13816,#11354,.T.) ;
#17490=EDGE_CURVE('',#13819,#13820,#11355,.T.) ;
#17491=EDGE_CURVE('',#13820,#13821,#11356,.T.) ;
#17492=EDGE_CURVE('',#13821,#13819,#11357,.T.) ;
#17493=EDGE_CURVE('',#13822,#13823,#11358,.T.) ;
#17494=EDGE_CURVE('',#13823,#13824,#11359,.T.) ;
#17495=EDGE_CURVE('',#13824,#13822,#11360,.T.) ;
#17496=EDGE_CURVE('',#13825,#13826,#11361,.T.) ;
#17497=EDGE_CURVE('',#13826,#13827,#11362,.T.) ;
#17498=EDGE_CURVE('',#13828,#13827,#11363,.T.) ;
#17499=EDGE_CURVE('',#13827,#13829,#11364,.T.) ;
#17500=EDGE_CURVE('',#13829,#13825,#11365,.T.) ;
#17501=EDGE_CURVE('',#13830,#13831,#11366,.T.) ;
#17502=EDGE_CURVE('',#13831,#13832,#11367,.T.) ;
#17503=EDGE_CURVE('',#13832,#13830,#11368,.T.) ;
#17504=EDGE_CURVE('',#13833,#13834,#11369,.T.) ;
#17505=EDGE_CURVE('',#13834,#13835,#11370,.T.) ;
#17506=EDGE_CURVE('',#13835,#13833,#11371,.T.) ;
#17507=EDGE_CURVE('',#13836,#13837,#11372,.T.) ;
#17508=EDGE_CURVE('',#13837,#13838,#11373,.T.) ;
#17509=EDGE_CURVE('',#13838,#13836,#11374,.T.) ;
#17510=EDGE_CURVE('',#13839,#13840,#11375,.T.) ;
#17511=EDGE_CURVE('',#13840,#13841,#11376,.T.) ;
#17512=EDGE_CURVE('',#13841,#13842,#11377,.T.) ;
#17513=EDGE_CURVE('',#13841,#13843,#11378,.T.) ;
#17514=EDGE_CURVE('',#13843,#13839,#11379,.T.) ;
#17515=EDGE_CURVE('',#13844,#13845,#11380,.T.) ;
#17516=EDGE_CURVE('',#13845,#13846,#11381,.T.) ;
#17517=EDGE_CURVE('',#13846,#13844,#11382,.T.) ;
#17518=EDGE_CURVE('',#13847,#13848,#11383,.T.) ;
#17519=EDGE_CURVE('',#13848,#13849,#11384,.T.) ;
#17520=EDGE_CURVE('',#13849,#13847,#11385,.T.) ;
#17521=EDGE_CURVE('',#13850,#13851,#11386,.T.) ;
#17522=EDGE_CURVE('',#13851,#13852,#11387,.T.) ;
#17523=EDGE_CURVE('',#13852,#13850,#11388,.T.) ;
#17524=EDGE_CURVE('',#13853,#13854,#11389,.T.) ;
#17525=EDGE_CURVE('',#13854,#13855,#11390,.T.) ;
#17526=EDGE_CURVE('',#13856,#13855,#11391,.T.) ;
#17527=EDGE_CURVE('',#13855,#13857,#11392,.T.) ;
#17528=EDGE_CURVE('',#13857,#13853,#11393,.T.) ;
#17529=EDGE_CURVE('',#13858,#13859,#11394,.T.) ;
#17530=EDGE_CURVE('',#13859,#13860,#11395,.T.) ;
#17531=EDGE_CURVE('',#13860,#13858,#11396,.T.) ;
#17532=EDGE_CURVE('',#13861,#13862,#11397,.T.) ;
#17533=EDGE_CURVE('',#13862,#13863,#11398,.T.) ;
#17534=EDGE_CURVE('',#13863,#13861,#11399,.T.) ;
#17535=EDGE_CURVE('',#13864,#13865,#11400,.T.) ;
#17536=EDGE_CURVE('',#13865,#13866,#11401,.T.) ;
#17537=EDGE_CURVE('',#13866,#13864,#11402,.T.) ;
#17538=EDGE_CURVE('',#13867,#13868,#11403,.T.) ;
#17539=EDGE_CURVE('',#13868,#13869,#11404,.T.) ;
#17540=EDGE_CURVE('',#13869,#13870,#11405,.T.) ;
#17541=EDGE_CURVE('',#13869,#13871,#11406,.T.) ;
#17542=EDGE_CURVE('',#13871,#13867,#11407,.T.) ;
#17543=EDGE_CURVE('',#13872,#13873,#11408,.T.) ;
#17544=EDGE_CURVE('',#13873,#13874,#11409,.T.) ;
#17545=EDGE_CURVE('',#13874,#13872,#11410,.T.) ;
#17546=EDGE_CURVE('',#13875,#13876,#11411,.T.) ;
#17547=EDGE_CURVE('',#13876,#13877,#11412,.T.) ;
#17548=EDGE_CURVE('',#13877,#13875,#11413,.T.) ;
#17549=EDGE_CURVE('',#13878,#13879,#11414,.T.) ;
#17550=EDGE_CURVE('',#13879,#13880,#11415,.T.) ;
#17551=EDGE_CURVE('',#13880,#13878,#11416,.T.) ;
#17552=EDGE_CURVE('',#13881,#13882,#11417,.T.) ;
#17553=EDGE_CURVE('',#13882,#13883,#11418,.T.) ;
#17554=EDGE_CURVE('',#13884,#13883,#11419,.T.) ;
#17555=EDGE_CURVE('',#13883,#13885,#11420,.T.) ;
#17556=EDGE_CURVE('',#13885,#13881,#11421,.T.) ;
#17557=EDGE_CURVE('',#13886,#13887,#11422,.T.) ;
#17558=EDGE_CURVE('',#13887,#13888,#11423,.T.) ;
#17559=EDGE_CURVE('',#13888,#13886,#11424,.T.) ;
#17560=EDGE_CURVE('',#13889,#13890,#11425,.T.) ;
#17561=EDGE_CURVE('',#13890,#13891,#11426,.T.) ;
#17562=EDGE_CURVE('',#13891,#13889,#11427,.T.) ;
#17563=EDGE_CURVE('',#13892,#13893,#11428,.T.) ;
#17564=EDGE_CURVE('',#13893,#13894,#11429,.T.) ;
#17565=EDGE_CURVE('',#13894,#13892,#11430,.T.) ;
#17566=EDGE_CURVE('',#13895,#13896,#11431,.T.) ;
#17567=EDGE_CURVE('',#13896,#13897,#11432,.T.) ;
#17568=EDGE_CURVE('',#13897,#13898,#11433,.T.) ;
#17569=EDGE_CURVE('',#13897,#13899,#11434,.T.) ;
#17570=EDGE_CURVE('',#13899,#13895,#11435,.T.) ;
#17571=EDGE_CURVE('',#13900,#13901,#11436,.T.) ;
#17572=EDGE_CURVE('',#13901,#13902,#11437,.T.) ;
#17573=EDGE_CURVE('',#13902,#13900,#11438,.T.) ;
#17574=EDGE_CURVE('',#13903,#13904,#11439,.T.) ;
#17575=EDGE_CURVE('',#13904,#13905,#11440,.T.) ;
#17576=EDGE_CURVE('',#13905,#13903,#11441,.T.) ;
#17577=EDGE_CURVE('',#13906,#13907,#11442,.T.) ;
#17578=EDGE_CURVE('',#13907,#13908,#11443,.T.) ;
#17579=EDGE_CURVE('',#13908,#13906,#11444,.T.) ;
#17580=EDGE_CURVE('',#13909,#13910,#11445,.T.) ;
#17581=EDGE_CURVE('',#13910,#13911,#11446,.T.) ;
#17582=EDGE_CURVE('',#13912,#13911,#11447,.T.) ;
#17583=EDGE_CURVE('',#13911,#13913,#11448,.T.) ;
#17584=EDGE_CURVE('',#13913,#13909,#11449,.T.) ;
#17585=EDGE_CURVE('',#13914,#13915,#11450,.T.) ;
#17586=EDGE_CURVE('',#13915,#13916,#11451,.T.) ;
#17587=EDGE_CURVE('',#13916,#13914,#11452,.T.) ;
#17588=EDGE_CURVE('',#13917,#13918,#11453,.T.) ;
#17589=EDGE_CURVE('',#13918,#13919,#11454,.T.) ;
#17590=EDGE_CURVE('',#13919,#13917,#11455,.T.) ;
#17591=EDGE_CURVE('',#13920,#13921,#11456,.T.) ;
#17592=EDGE_CURVE('',#13921,#13922,#11457,.T.) ;
#17593=EDGE_CURVE('',#13922,#13920,#11458,.T.) ;
#17594=EDGE_CURVE('',#13923,#13924,#11459,.T.) ;
#17595=EDGE_CURVE('',#13924,#13925,#11460,.T.) ;
#17596=EDGE_CURVE('',#13925,#13926,#11461,.T.) ;
#17597=EDGE_CURVE('',#13925,#13927,#11462,.T.) ;
#17598=EDGE_CURVE('',#13927,#13923,#11463,.T.) ;
#17599=EDGE_CURVE('',#13928,#13929,#11464,.T.) ;
#17600=EDGE_CURVE('',#13929,#13930,#11465,.T.) ;
#17601=EDGE_CURVE('',#13930,#13928,#11466,.T.) ;
#17602=EDGE_CURVE('',#13931,#13932,#11467,.T.) ;
#17603=EDGE_CURVE('',#13932,#13933,#11468,.T.) ;
#17604=EDGE_CURVE('',#13933,#13931,#11469,.T.) ;
#17605=EDGE_CURVE('',#13934,#13935,#11470,.T.) ;
#17606=EDGE_CURVE('',#13935,#13936,#11471,.T.) ;
#17607=EDGE_CURVE('',#13936,#13934,#11472,.T.) ;
#17608=EDGE_CURVE('',#13937,#13938,#11473,.T.) ;
#17609=EDGE_CURVE('',#13938,#13939,#11474,.T.) ;
#17610=EDGE_CURVE('',#13940,#13939,#11475,.T.) ;
#17611=EDGE_CURVE('',#13939,#13941,#11476,.T.) ;
#17612=EDGE_CURVE('',#13941,#13937,#11477,.T.) ;
#17613=EDGE_CURVE('',#13942,#13943,#11478,.T.) ;
#17614=EDGE_CURVE('',#13943,#13944,#11479,.T.) ;
#17615=EDGE_CURVE('',#13944,#13942,#11480,.T.) ;
#17616=EDGE_CURVE('',#13945,#13946,#11481,.T.) ;
#17617=EDGE_CURVE('',#13946,#13947,#11482,.T.) ;
#17618=EDGE_CURVE('',#13947,#13945,#11483,.T.) ;
#17619=EDGE_CURVE('',#13948,#13949,#11484,.T.) ;
#17620=EDGE_CURVE('',#13949,#13950,#11485,.T.) ;
#17621=EDGE_CURVE('',#13950,#13948,#11486,.T.) ;
#17622=EDGE_CURVE('',#13951,#13952,#11487,.T.) ;
#17623=EDGE_CURVE('',#13952,#13953,#11488,.T.) ;
#17624=EDGE_CURVE('',#13953,#13954,#11489,.T.) ;
#17625=EDGE_CURVE('',#13953,#13955,#11490,.T.) ;
#17626=EDGE_CURVE('',#13955,#13951,#11491,.T.) ;
#17627=EDGE_CURVE('',#13956,#13957,#11492,.T.) ;
#17628=EDGE_CURVE('',#13957,#13958,#11493,.T.) ;
#17629=EDGE_CURVE('',#13958,#13956,#11494,.T.) ;
#17630=EDGE_CURVE('',#13959,#13960,#11495,.T.) ;
#17631=EDGE_CURVE('',#13960,#13961,#11496,.T.) ;
#17632=EDGE_CURVE('',#13961,#13959,#11497,.T.) ;
#17633=EDGE_CURVE('',#13962,#13963,#11498,.T.) ;
#17634=EDGE_CURVE('',#13963,#13964,#11499,.T.) ;
#17635=EDGE_CURVE('',#13964,#13962,#11500,.T.) ;
#17636=EDGE_CURVE('',#13965,#13966,#11501,.T.) ;
#17637=EDGE_CURVE('',#13966,#13967,#11502,.T.) ;
#17638=EDGE_CURVE('',#13968,#13967,#11503,.T.) ;
#17639=EDGE_CURVE('',#13967,#13969,#11504,.T.) ;
#17640=EDGE_CURVE('',#13969,#13965,#11505,.T.) ;
#17641=EDGE_CURVE('',#13970,#13971,#11506,.T.) ;
#17642=EDGE_CURVE('',#13971,#13972,#11507,.T.) ;
#17643=EDGE_CURVE('',#13972,#13970,#11508,.T.) ;
#17644=EDGE_CURVE('',#13973,#13974,#11509,.T.) ;
#17645=EDGE_CURVE('',#13974,#13975,#11510,.T.) ;
#17646=EDGE_CURVE('',#13975,#13973,#11511,.T.) ;
#17647=EDGE_CURVE('',#13976,#13977,#11512,.T.) ;
#17648=EDGE_CURVE('',#13977,#13978,#11513,.T.) ;
#17649=EDGE_CURVE('',#13978,#13976,#11514,.T.) ;
#17650=EDGE_CURVE('',#13979,#13980,#11515,.T.) ;
#17651=EDGE_CURVE('',#13980,#13981,#11516,.T.) ;
#17652=EDGE_CURVE('',#13981,#13982,#11517,.T.) ;
#17653=EDGE_CURVE('',#13981,#13983,#11518,.T.) ;
#17654=EDGE_CURVE('',#13983,#13979,#11519,.T.) ;
#17655=EDGE_CURVE('',#13984,#13985,#11520,.T.) ;
#17656=EDGE_CURVE('',#13985,#13986,#11521,.T.) ;
#17657=EDGE_CURVE('',#13986,#13984,#11522,.T.) ;
#17658=EDGE_CURVE('',#13987,#13988,#11523,.T.) ;
#17659=EDGE_CURVE('',#13988,#13989,#11524,.T.) ;
#17660=EDGE_CURVE('',#13989,#13987,#11525,.T.) ;
#17661=EDGE_CURVE('',#13990,#13991,#11526,.T.) ;
#17662=EDGE_CURVE('',#13991,#13992,#11527,.T.) ;
#17663=EDGE_CURVE('',#13992,#13990,#11528,.T.) ;
#17664=EDGE_CURVE('',#13993,#13994,#11529,.T.) ;
#17665=EDGE_CURVE('',#13994,#13995,#11530,.T.) ;
#17666=EDGE_CURVE('',#13996,#13995,#11531,.T.) ;
#17667=EDGE_CURVE('',#13995,#13997,#11532,.T.) ;
#17668=EDGE_CURVE('',#13997,#13993,#11533,.T.) ;
#17669=EDGE_CURVE('',#13998,#13999,#11534,.T.) ;
#17670=EDGE_CURVE('',#13999,#14000,#11535,.T.) ;
#17671=EDGE_CURVE('',#14000,#13998,#11536,.T.) ;
#17672=EDGE_CURVE('',#14001,#14002,#11537,.T.) ;
#17673=EDGE_CURVE('',#14002,#14003,#11538,.T.) ;
#17674=EDGE_CURVE('',#14003,#14001,#11539,.T.) ;
#17675=EDGE_CURVE('',#14004,#14005,#11540,.T.) ;
#17676=EDGE_CURVE('',#14005,#14006,#11541,.T.) ;
#17677=EDGE_CURVE('',#14006,#14004,#11542,.T.) ;
#17678=EDGE_CURVE('',#14007,#14008,#11543,.T.) ;
#17679=EDGE_CURVE('',#14008,#14009,#11544,.T.) ;
#17680=EDGE_CURVE('',#14009,#14010,#11545,.T.) ;
#17681=EDGE_CURVE('',#14009,#14011,#11546,.T.) ;
#17682=EDGE_CURVE('',#14011,#14007,#11547,.T.) ;
#17683=EDGE_CURVE('',#14012,#14013,#11548,.T.) ;
#17684=EDGE_CURVE('',#14013,#14014,#11549,.T.) ;
#17685=EDGE_CURVE('',#14014,#14012,#11550,.T.) ;
#17686=EDGE_CURVE('',#14015,#14016,#11551,.T.) ;
#17687=EDGE_CURVE('',#14016,#14017,#11552,.T.) ;
#17688=EDGE_CURVE('',#14017,#14015,#11553,.T.) ;
#17689=EDGE_CURVE('',#14018,#14019,#11554,.T.) ;
#17690=EDGE_CURVE('',#14019,#14020,#11555,.T.) ;
#17691=EDGE_CURVE('',#14020,#14018,#11556,.T.) ;
#17692=EDGE_CURVE('',#14021,#14022,#11557,.T.) ;
#17693=EDGE_CURVE('',#14022,#14023,#11558,.T.) ;
#17694=EDGE_CURVE('',#14024,#14023,#11559,.T.) ;
#17695=EDGE_CURVE('',#14023,#14025,#11560,.T.) ;
#17696=EDGE_CURVE('',#14025,#14021,#11561,.T.) ;
#17697=EDGE_CURVE('',#14026,#14027,#11562,.T.) ;
#17698=EDGE_CURVE('',#14027,#14028,#11563,.T.) ;
#17699=EDGE_CURVE('',#14028,#14026,#11564,.T.) ;
#17700=EDGE_CURVE('',#14029,#14030,#11565,.T.) ;
#17701=EDGE_CURVE('',#14030,#14031,#11566,.T.) ;
#17702=EDGE_CURVE('',#14031,#14029,#11567,.T.) ;
#17703=EDGE_CURVE('',#14032,#14033,#11568,.T.) ;
#17704=EDGE_CURVE('',#14033,#14034,#11569,.T.) ;
#17705=EDGE_CURVE('',#14034,#14032,#11570,.T.) ;
#17706=EDGE_CURVE('',#14035,#14036,#11571,.T.) ;
#17707=EDGE_CURVE('',#14036,#14037,#11572,.T.) ;
#17708=EDGE_CURVE('',#14037,#14038,#11573,.T.) ;
#17709=EDGE_CURVE('',#14037,#14039,#11574,.T.) ;
#17710=EDGE_CURVE('',#14039,#14035,#11575,.T.) ;
#17711=EDGE_CURVE('',#14040,#14041,#11576,.T.) ;
#17712=EDGE_CURVE('',#14041,#14042,#11577,.T.) ;
#17713=EDGE_CURVE('',#14042,#14040,#11578,.T.) ;
#17714=EDGE_CURVE('',#14043,#14044,#11579,.T.) ;
#17715=EDGE_CURVE('',#14044,#14045,#11580,.T.) ;
#17716=EDGE_CURVE('',#14045,#14043,#11581,.T.) ;
#17717=EDGE_CURVE('',#14046,#14047,#11582,.T.) ;
#17718=EDGE_CURVE('',#14047,#14048,#11583,.T.) ;
#17719=EDGE_CURVE('',#14048,#14046,#11584,.T.) ;
#17720=EDGE_CURVE('',#14049,#14050,#11585,.T.) ;
#17721=EDGE_CURVE('',#14050,#14051,#11586,.T.) ;
#17722=EDGE_CURVE('',#14052,#14051,#11587,.T.) ;
#17723=EDGE_CURVE('',#14051,#14053,#11588,.T.) ;
#17724=EDGE_CURVE('',#14053,#14049,#11589,.T.) ;
#17725=EDGE_CURVE('',#14054,#14055,#11590,.T.) ;
#17726=EDGE_CURVE('',#14055,#14056,#11591,.T.) ;
#17727=EDGE_CURVE('',#14056,#14054,#11592,.T.) ;
#17728=EDGE_CURVE('',#14057,#14058,#11593,.T.) ;
#17729=EDGE_CURVE('',#14058,#14059,#11594,.T.) ;
#17730=EDGE_CURVE('',#14059,#14057,#11595,.T.) ;
#17731=EDGE_CURVE('',#14060,#14061,#11596,.T.) ;
#17732=EDGE_CURVE('',#14061,#14062,#11597,.T.) ;
#17733=EDGE_CURVE('',#14062,#14060,#11598,.T.) ;
#17734=EDGE_CURVE('',#14063,#14064,#11599,.T.) ;
#17735=EDGE_CURVE('',#14064,#14065,#11600,.T.) ;
#17736=EDGE_CURVE('',#14065,#14066,#11601,.T.) ;
#17737=EDGE_CURVE('',#14065,#14067,#11602,.T.) ;
#17738=EDGE_CURVE('',#14067,#14063,#11603,.T.) ;
#17739=EDGE_CURVE('',#14068,#14069,#11604,.T.) ;
#17740=EDGE_CURVE('',#14069,#14070,#11605,.T.) ;
#17741=EDGE_CURVE('',#14070,#14068,#11606,.T.) ;
#17742=EDGE_CURVE('',#14071,#14072,#11607,.T.) ;
#17743=EDGE_CURVE('',#14072,#14073,#11608,.T.) ;
#17744=EDGE_CURVE('',#14073,#14071,#11609,.T.) ;
#17745=EDGE_CURVE('',#14074,#14075,#11610,.T.) ;
#17746=EDGE_CURVE('',#14075,#14076,#11611,.T.) ;
#17747=EDGE_CURVE('',#14076,#14074,#11612,.T.) ;
#17748=EDGE_CURVE('',#14077,#14078,#11613,.T.) ;
#17749=EDGE_CURVE('',#14078,#14079,#11614,.T.) ;
#17750=EDGE_CURVE('',#14080,#14079,#11615,.T.) ;
#17751=EDGE_CURVE('',#14079,#14081,#11616,.T.) ;
#17752=EDGE_CURVE('',#14081,#14077,#11617,.T.) ;
#17753=EDGE_CURVE('',#14082,#14083,#11618,.T.) ;
#17754=EDGE_CURVE('',#14083,#14084,#11619,.T.) ;
#17755=EDGE_CURVE('',#14084,#14082,#11620,.T.) ;
#17756=EDGE_CURVE('',#14085,#14086,#11621,.T.) ;
#17757=EDGE_CURVE('',#14086,#14087,#11622,.T.) ;
#17758=EDGE_CURVE('',#14087,#14085,#11623,.T.) ;
#17759=EDGE_CURVE('',#14088,#14089,#11624,.T.) ;
#17760=EDGE_CURVE('',#14089,#14090,#11625,.T.) ;
#17761=EDGE_CURVE('',#14090,#14088,#11626,.T.) ;
#17762=EDGE_CURVE('',#14091,#14092,#11627,.T.) ;
#17763=EDGE_CURVE('',#14092,#14093,#11628,.T.) ;
#17764=EDGE_CURVE('',#14093,#14094,#11629,.T.) ;
#17765=EDGE_CURVE('',#14093,#14095,#11630,.T.) ;
#17766=EDGE_CURVE('',#14095,#14091,#11631,.T.) ;
#17767=EDGE_CURVE('',#14096,#14097,#11632,.T.) ;
#17768=EDGE_CURVE('',#14097,#14098,#11633,.T.) ;
#17769=EDGE_CURVE('',#14098,#14096,#11634,.T.) ;
#17770=EDGE_CURVE('',#14099,#14100,#11635,.T.) ;
#17771=EDGE_CURVE('',#14100,#14101,#11636,.T.) ;
#17772=EDGE_CURVE('',#14101,#14099,#11637,.T.) ;
#17773=EDGE_CURVE('',#14102,#14103,#11638,.T.) ;
#17774=EDGE_CURVE('',#14103,#14104,#11639,.T.) ;
#17775=EDGE_CURVE('',#14104,#14102,#11640,.T.) ;
#17776=EDGE_CURVE('',#14105,#14106,#11641,.T.) ;
#17777=EDGE_CURVE('',#14106,#14107,#11642,.T.) ;
#17778=EDGE_CURVE('',#14108,#14107,#11643,.T.) ;
#17779=EDGE_CURVE('',#14107,#14109,#11644,.T.) ;
#17780=EDGE_CURVE('',#14109,#14105,#11645,.T.) ;
#17781=EDGE_CURVE('',#14110,#14111,#11646,.T.) ;
#17782=EDGE_CURVE('',#14111,#14112,#11647,.T.) ;
#17783=EDGE_CURVE('',#14112,#14110,#11648,.T.) ;
#17784=EDGE_CURVE('',#14113,#14114,#11649,.T.) ;
#17785=EDGE_CURVE('',#14114,#14115,#11650,.T.) ;
#17786=EDGE_CURVE('',#14115,#14113,#11651,.T.) ;
#17787=EDGE_CURVE('',#14116,#14117,#11652,.T.) ;
#17788=EDGE_CURVE('',#14117,#14118,#11653,.T.) ;
#17789=EDGE_CURVE('',#14118,#14116,#11654,.T.) ;
#17790=EDGE_CURVE('',#14119,#14120,#11655,.T.) ;
#17791=EDGE_CURVE('',#14120,#14121,#11656,.T.) ;
#17792=EDGE_CURVE('',#14121,#14122,#11657,.T.) ;
#17793=EDGE_CURVE('',#14121,#14123,#11658,.T.) ;
#17794=EDGE_CURVE('',#14123,#14119,#11659,.T.) ;
#17795=EDGE_CURVE('',#14124,#14125,#11660,.T.) ;
#17796=EDGE_CURVE('',#14125,#14126,#11661,.T.) ;
#17797=EDGE_CURVE('',#14126,#14124,#11662,.T.) ;
#17798=EDGE_CURVE('',#14127,#14128,#11663,.T.) ;
#17799=EDGE_CURVE('',#14128,#14129,#11664,.T.) ;
#17800=EDGE_CURVE('',#14129,#14127,#11665,.T.) ;
#17801=EDGE_CURVE('',#14130,#14131,#11666,.T.) ;
#17802=EDGE_CURVE('',#14131,#14132,#11667,.T.) ;
#17803=EDGE_CURVE('',#14132,#14130,#11668,.T.) ;
#17804=EDGE_CURVE('',#14133,#14134,#11669,.T.) ;
#17805=EDGE_CURVE('',#14134,#14135,#11670,.T.) ;
#17806=EDGE_CURVE('',#14136,#14135,#11671,.T.) ;
#17807=EDGE_CURVE('',#14135,#14137,#11672,.T.) ;
#17808=EDGE_CURVE('',#14137,#14133,#11673,.T.) ;
#17809=EDGE_CURVE('',#14138,#14139,#11674,.T.) ;
#17810=EDGE_CURVE('',#14139,#14140,#11675,.T.) ;
#17811=EDGE_CURVE('',#14140,#14138,#11676,.T.) ;
#17812=EDGE_CURVE('',#14141,#14142,#11677,.T.) ;
#17813=EDGE_CURVE('',#14142,#14143,#11678,.T.) ;
#17814=EDGE_CURVE('',#14143,#14141,#11679,.T.) ;
#17815=EDGE_CURVE('',#14144,#14145,#11680,.T.) ;
#17816=EDGE_CURVE('',#14145,#14146,#11681,.T.) ;
#17817=EDGE_CURVE('',#14146,#14144,#11682,.T.) ;
#17818=EDGE_CURVE('',#14147,#14148,#11683,.T.) ;
#17819=EDGE_CURVE('',#14148,#14149,#11684,.T.) ;
#17820=EDGE_CURVE('',#14149,#14150,#11685,.T.) ;
#17821=EDGE_CURVE('',#14149,#14151,#11686,.T.) ;
#17822=EDGE_CURVE('',#14151,#14147,#11687,.T.) ;
#17823=EDGE_CURVE('',#14152,#14153,#11688,.T.) ;
#17824=EDGE_CURVE('',#14153,#14154,#11689,.T.) ;
#17825=EDGE_CURVE('',#14154,#14152,#11690,.T.) ;
#17826=EDGE_CURVE('',#14155,#14156,#11691,.T.) ;
#17827=EDGE_CURVE('',#14156,#14157,#11692,.T.) ;
#17828=EDGE_CURVE('',#14157,#14155,#11693,.T.) ;
#17829=EDGE_CURVE('',#14158,#14159,#11694,.T.) ;
#17830=EDGE_CURVE('',#14159,#14160,#11695,.T.) ;
#17831=EDGE_CURVE('',#14160,#14158,#11696,.T.) ;
#17832=EDGE_CURVE('',#14161,#14162,#11697,.T.) ;
#17833=EDGE_CURVE('',#14162,#14163,#11698,.T.) ;
#17834=EDGE_CURVE('',#14164,#14163,#11699,.T.) ;
#17835=EDGE_CURVE('',#14163,#14165,#11700,.T.) ;
#17836=EDGE_CURVE('',#14165,#14161,#11701,.T.) ;
#17837=EDGE_CURVE('',#14166,#14167,#11702,.T.) ;
#17838=EDGE_CURVE('',#14167,#14168,#11703,.T.) ;
#17839=EDGE_CURVE('',#14168,#14166,#11704,.T.) ;
#17840=EDGE_CURVE('',#14169,#14170,#11705,.T.) ;
#17841=EDGE_CURVE('',#14170,#14171,#11706,.T.) ;
#17842=EDGE_CURVE('',#14171,#14169,#11707,.T.) ;
#17843=EDGE_CURVE('',#14172,#14173,#11708,.T.) ;
#17844=EDGE_CURVE('',#14173,#14174,#11709,.T.) ;
#17845=EDGE_CURVE('',#14174,#14172,#11710,.T.) ;
#17846=EDGE_CURVE('',#14175,#14176,#11711,.T.) ;
#17847=EDGE_CURVE('',#14176,#14177,#11712,.T.) ;
#17848=EDGE_CURVE('',#14177,#14178,#11713,.T.) ;
#17849=EDGE_CURVE('',#14177,#14179,#11714,.T.) ;
#17850=EDGE_CURVE('',#14179,#14175,#11715,.T.) ;
#17851=EDGE_CURVE('',#14180,#14181,#11716,.T.) ;
#17852=EDGE_CURVE('',#14181,#14182,#11717,.T.) ;
#17853=EDGE_CURVE('',#14182,#14180,#11718,.T.) ;
#17854=EDGE_CURVE('',#14183,#14184,#11719,.T.) ;
#17855=EDGE_CURVE('',#14184,#14185,#11720,.T.) ;
#17856=EDGE_CURVE('',#14185,#14183,#11721,.T.) ;
#17857=EDGE_CURVE('',#14186,#14187,#11722,.T.) ;
#17858=EDGE_CURVE('',#14187,#14188,#11723,.T.) ;
#17859=EDGE_CURVE('',#14188,#14186,#11724,.T.) ;
#17860=EDGE_CURVE('',#14189,#14190,#11725,.T.) ;
#17861=EDGE_CURVE('',#14190,#14191,#11726,.T.) ;
#17862=EDGE_CURVE('',#14192,#14191,#11727,.T.) ;
#17863=EDGE_CURVE('',#14191,#14193,#11728,.T.) ;
#17864=EDGE_CURVE('',#14193,#14189,#11729,.T.) ;
#17865=EDGE_CURVE('',#14194,#14195,#11730,.T.) ;
#17866=EDGE_CURVE('',#14195,#14196,#11731,.T.) ;
#17867=EDGE_CURVE('',#14196,#14194,#11732,.T.) ;
#17868=EDGE_CURVE('',#14197,#14198,#11733,.T.) ;
#17869=EDGE_CURVE('',#14198,#14199,#11734,.T.) ;
#17870=EDGE_CURVE('',#14199,#14197,#11735,.T.) ;
#17871=EDGE_CURVE('',#14200,#14201,#11736,.T.) ;
#17872=EDGE_CURVE('',#14201,#14202,#11737,.T.) ;
#17873=EDGE_CURVE('',#14202,#14200,#11738,.T.) ;
#17874=EDGE_CURVE('',#14203,#14204,#11739,.T.) ;
#17875=EDGE_CURVE('',#14204,#14205,#11740,.T.) ;
#17876=EDGE_CURVE('',#14205,#14206,#11741,.T.) ;
#17877=EDGE_CURVE('',#14205,#14207,#11742,.T.) ;
#17878=EDGE_CURVE('',#14207,#14203,#11743,.T.) ;
#17879=EDGE_CURVE('',#14208,#14209,#11744,.T.) ;
#17880=EDGE_CURVE('',#14209,#14210,#11745,.T.) ;
#17881=EDGE_CURVE('',#14210,#14208,#11746,.T.) ;
#17882=EDGE_CURVE('',#14211,#14212,#11747,.T.) ;
#17883=EDGE_CURVE('',#14212,#14213,#11748,.T.) ;
#17884=EDGE_CURVE('',#14213,#14211,#11749,.T.) ;
#17885=EDGE_CURVE('',#14214,#14215,#11750,.T.) ;
#17886=EDGE_CURVE('',#14215,#14216,#11751,.T.) ;
#17887=EDGE_CURVE('',#14216,#14214,#11752,.T.) ;
#17888=EDGE_CURVE('',#13766,#13777,#421,.T.) ;
#17889=EDGE_CURVE('',#13767,#13779,#422,.T.) ;
#17890=EDGE_CURVE('',#13778,#14217,#7909,.T.) ;
#17891=EDGE_CURVE('',#13781,#14217,#423,.T.) ;
#17892=EDGE_CURVE('',#14217,#13780,#424,.T.) ;
#17893=EDGE_CURVE('',#13782,#14218,#7910,.T.) ;
#17894=EDGE_CURVE('',#13784,#14218,#425,.T.) ;
#17895=EDGE_CURVE('',#14218,#13783,#426,.T.) ;
#17896=EDGE_CURVE('',#13787,#14219,#7911,.T.) ;
#17897=EDGE_CURVE('',#13789,#14219,#427,.T.) ;
#17898=EDGE_CURVE('',#14219,#13788,#428,.T.) ;
#17899=EDGE_CURVE('',#13790,#14220,#7912,.T.) ;
#17900=EDGE_CURVE('',#13792,#14220,#429,.T.) ;
#17901=EDGE_CURVE('',#14220,#13791,#430,.T.) ;
#17902=EDGE_CURVE('',#13793,#14221,#7913,.T.) ;
#17903=EDGE_CURVE('',#13795,#14221,#431,.T.) ;
#17904=EDGE_CURVE('',#14221,#13794,#432,.T.) ;
#17905=EDGE_CURVE('',#13796,#14222,#7914,.T.) ;
#17906=EDGE_CURVE('',#13798,#14222,#433,.T.) ;
#17907=EDGE_CURVE('',#14222,#13797,#434,.T.) ;
#17908=EDGE_CURVE('',#13801,#14223,#7915,.T.) ;
#17909=EDGE_CURVE('',#13803,#14223,#435,.T.) ;
#17910=EDGE_CURVE('',#14223,#13802,#436,.T.) ;
#17911=EDGE_CURVE('',#13804,#14224,#7916,.T.) ;
#17912=EDGE_CURVE('',#13806,#14224,#437,.T.) ;
#17913=EDGE_CURVE('',#14224,#13805,#438,.T.) ;
#17914=EDGE_CURVE('',#13807,#14225,#7917,.T.) ;
#17915=EDGE_CURVE('',#13809,#14225,#439,.T.) ;
#17916=EDGE_CURVE('',#14225,#13808,#440,.T.) ;
#17917=EDGE_CURVE('',#13810,#14226,#7918,.T.) ;
#17918=EDGE_CURVE('',#13812,#14226,#441,.T.) ;
#17919=EDGE_CURVE('',#14226,#13811,#442,.T.) ;
#17920=EDGE_CURVE('',#13815,#14227,#7919,.T.) ;
#17921=EDGE_CURVE('',#13817,#14227,#443,.T.) ;
#17922=EDGE_CURVE('',#14227,#13816,#444,.T.) ;
#17923=EDGE_CURVE('',#13818,#14228,#7920,.T.) ;
#17924=EDGE_CURVE('',#13820,#14228,#445,.T.) ;
#17925=EDGE_CURVE('',#14228,#13819,#446,.T.) ;
#17926=EDGE_CURVE('',#13821,#14229,#7921,.T.) ;
#17927=EDGE_CURVE('',#13823,#14229,#447,.T.) ;
#17928=EDGE_CURVE('',#14229,#13822,#448,.T.) ;
#17929=EDGE_CURVE('',#13824,#14230,#7922,.T.) ;
#17930=EDGE_CURVE('',#13826,#14230,#449,.T.) ;
#17931=EDGE_CURVE('',#14230,#13825,#450,.T.) ;
#17932=EDGE_CURVE('',#13829,#14231,#7923,.T.) ;
#17933=EDGE_CURVE('',#13831,#14231,#451,.T.) ;
#17934=EDGE_CURVE('',#14231,#13830,#452,.T.) ;
#17935=EDGE_CURVE('',#13832,#14232,#7924,.T.) ;
#17936=EDGE_CURVE('',#13834,#14232,#453,.T.) ;
#17937=EDGE_CURVE('',#14232,#13833,#454,.T.) ;
#17938=EDGE_CURVE('',#13835,#14233,#7925,.T.) ;
#17939=EDGE_CURVE('',#13837,#14233,#455,.T.) ;
#17940=EDGE_CURVE('',#14233,#13836,#456,.T.) ;
#17941=EDGE_CURVE('',#13838,#14234,#7926,.T.) ;
#17942=EDGE_CURVE('',#13840,#14234,#457,.T.) ;
#17943=EDGE_CURVE('',#14234,#13839,#458,.T.) ;
#17944=EDGE_CURVE('',#13843,#14235,#7927,.T.) ;
#17945=EDGE_CURVE('',#13845,#14235,#459,.T.) ;
#17946=EDGE_CURVE('',#14235,#13844,#460,.T.) ;
#17947=EDGE_CURVE('',#13846,#14236,#7928,.T.) ;
#17948=EDGE_CURVE('',#13848,#14236,#461,.T.) ;
#17949=EDGE_CURVE('',#14236,#13847,#462,.T.) ;
#17950=EDGE_CURVE('',#13849,#14237,#7929,.T.) ;
#17951=EDGE_CURVE('',#13851,#14237,#463,.T.) ;
#17952=EDGE_CURVE('',#14237,#13850,#464,.T.) ;
#17953=EDGE_CURVE('',#13852,#14238,#7930,.T.) ;
#17954=EDGE_CURVE('',#13854,#14238,#465,.T.) ;
#17955=EDGE_CURVE('',#14238,#13853,#466,.T.) ;
#17956=EDGE_CURVE('',#13857,#14239,#7931,.T.) ;
#17957=EDGE_CURVE('',#13859,#14239,#467,.T.) ;
#17958=EDGE_CURVE('',#14239,#13858,#468,.T.) ;
#17959=EDGE_CURVE('',#13860,#14240,#7932,.T.) ;
#17960=EDGE_CURVE('',#13862,#14240,#469,.T.) ;
#17961=EDGE_CURVE('',#14240,#13861,#470,.T.) ;
#17962=EDGE_CURVE('',#13863,#14241,#7933,.T.) ;
#17963=EDGE_CURVE('',#13865,#14241,#471,.T.) ;
#17964=EDGE_CURVE('',#14241,#13864,#472,.T.) ;
#17965=EDGE_CURVE('',#13866,#14242,#7934,.T.) ;
#17966=EDGE_CURVE('',#13868,#14242,#473,.T.) ;
#17967=EDGE_CURVE('',#14242,#13867,#474,.T.) ;
#17968=EDGE_CURVE('',#13871,#14243,#7935,.T.) ;
#17969=EDGE_CURVE('',#13873,#14243,#475,.T.) ;
#17970=EDGE_CURVE('',#14243,#13872,#476,.T.) ;
#17971=EDGE_CURVE('',#13874,#14244,#7936,.T.) ;
#17972=EDGE_CURVE('',#13876,#14244,#477,.T.) ;
#17973=EDGE_CURVE('',#14244,#13875,#478,.T.) ;
#17974=EDGE_CURVE('',#13877,#14245,#7937,.T.) ;
#17975=EDGE_CURVE('',#13879,#14245,#479,.T.) ;
#17976=EDGE_CURVE('',#14245,#13878,#480,.T.) ;
#17977=EDGE_CURVE('',#13880,#14246,#7938,.T.) ;
#17978=EDGE_CURVE('',#13882,#14246,#481,.T.) ;
#17979=EDGE_CURVE('',#14246,#13881,#482,.T.) ;
#17980=EDGE_CURVE('',#13885,#14247,#7939,.T.) ;
#17981=EDGE_CURVE('',#13887,#14247,#483,.T.) ;
#17982=EDGE_CURVE('',#14247,#13886,#484,.T.) ;
#17983=EDGE_CURVE('',#13888,#14248,#7940,.T.) ;
#17984=EDGE_CURVE('',#13890,#14248,#485,.T.) ;
#17985=EDGE_CURVE('',#14248,#13889,#486,.T.) ;
#17986=EDGE_CURVE('',#13891,#14249,#7941,.T.) ;
#17987=EDGE_CURVE('',#13893,#14249,#487,.T.) ;
#17988=EDGE_CURVE('',#14249,#13892,#488,.T.) ;
#17989=EDGE_CURVE('',#13894,#14250,#7942,.T.) ;
#17990=EDGE_CURVE('',#13896,#14250,#489,.T.) ;
#17991=EDGE_CURVE('',#14250,#13895,#490,.T.) ;
#17992=EDGE_CURVE('',#13899,#14251,#7943,.T.) ;
#17993=EDGE_CURVE('',#13901,#14251,#491,.T.) ;
#17994=EDGE_CURVE('',#14251,#13900,#492,.T.) ;
#17995=EDGE_CURVE('',#13902,#14252,#7944,.T.) ;
#17996=EDGE_CURVE('',#13904,#14252,#493,.T.) ;
#17997=EDGE_CURVE('',#14252,#13903,#494,.T.) ;
#17998=EDGE_CURVE('',#13905,#14253,#7945,.T.) ;
#17999=EDGE_CURVE('',#13907,#14253,#495,.T.) ;
#18000=EDGE_CURVE('',#14253,#13906,#496,.T.) ;
#18001=EDGE_CURVE('',#13908,#14254,#7946,.T.) ;
#18002=EDGE_CURVE('',#13910,#14254,#497,.T.) ;
#18003=EDGE_CURVE('',#14254,#13909,#498,.T.) ;
#18004=EDGE_CURVE('',#13913,#14255,#7947,.T.) ;
#18005=EDGE_CURVE('',#13915,#14255,#499,.T.) ;
#18006=EDGE_CURVE('',#14255,#13914,#500,.T.) ;
#18007=EDGE_CURVE('',#13916,#14256,#7948,.T.) ;
#18008=EDGE_CURVE('',#13918,#14256,#501,.T.) ;
#18009=EDGE_CURVE('',#14256,#13917,#502,.T.) ;
#18010=EDGE_CURVE('',#13919,#14257,#7949,.T.) ;
#18011=EDGE_CURVE('',#13921,#14257,#503,.T.) ;
#18012=EDGE_CURVE('',#14257,#13920,#504,.T.) ;
#18013=EDGE_CURVE('',#13922,#14258,#7950,.T.) ;
#18014=EDGE_CURVE('',#13924,#14258,#505,.T.) ;
#18015=EDGE_CURVE('',#14258,#13923,#506,.T.) ;
#18016=EDGE_CURVE('',#13927,#14259,#7951,.T.) ;
#18017=EDGE_CURVE('',#13929,#14259,#507,.T.) ;
#18018=EDGE_CURVE('',#14259,#13928,#508,.T.) ;
#18019=EDGE_CURVE('',#13930,#14260,#7952,.T.) ;
#18020=EDGE_CURVE('',#13932,#14260,#509,.T.) ;
#18021=EDGE_CURVE('',#14260,#13931,#510,.T.) ;
#18022=EDGE_CURVE('',#13933,#14261,#7953,.T.) ;
#18023=EDGE_CURVE('',#13935,#14261,#511,.T.) ;
#18024=EDGE_CURVE('',#14261,#13934,#512,.T.) ;
#18025=EDGE_CURVE('',#13936,#14262,#7954,.T.) ;
#18026=EDGE_CURVE('',#13938,#14262,#513,.T.) ;
#18027=EDGE_CURVE('',#14262,#13937,#514,.T.) ;
#18028=EDGE_CURVE('',#13941,#14263,#7955,.T.) ;
#18029=EDGE_CURVE('',#13943,#14263,#515,.T.) ;
#18030=EDGE_CURVE('',#14263,#13942,#516,.T.) ;
#18031=EDGE_CURVE('',#13944,#14264,#7956,.T.) ;
#18032=EDGE_CURVE('',#13946,#14264,#517,.T.) ;
#18033=EDGE_CURVE('',#14264,#13945,#518,.T.) ;
#18034=EDGE_CURVE('',#13947,#14265,#7957,.T.) ;
#18035=EDGE_CURVE('',#13949,#14265,#519,.T.) ;
#18036=EDGE_CURVE('',#14265,#13948,#520,.T.) ;
#18037=EDGE_CURVE('',#13950,#14266,#7958,.T.) ;
#18038=EDGE_CURVE('',#13952,#14266,#521,.T.) ;
#18039=EDGE_CURVE('',#14266,#13951,#522,.T.) ;
#18040=EDGE_CURVE('',#13955,#14267,#7959,.T.) ;
#18041=EDGE_CURVE('',#13957,#14267,#523,.T.) ;
#18042=EDGE_CURVE('',#14267,#13956,#524,.T.) ;
#18043=EDGE_CURVE('',#13958,#14268,#7960,.T.) ;
#18044=EDGE_CURVE('',#13960,#14268,#525,.T.) ;
#18045=EDGE_CURVE('',#14268,#13959,#526,.T.) ;
#18046=EDGE_CURVE('',#13961,#14269,#7961,.T.) ;
#18047=EDGE_CURVE('',#13963,#14269,#527,.T.) ;
#18048=EDGE_CURVE('',#14269,#13962,#528,.T.) ;
#18049=EDGE_CURVE('',#13964,#14270,#7962,.T.) ;
#18050=EDGE_CURVE('',#13966,#14270,#529,.T.) ;
#18051=EDGE_CURVE('',#14270,#13965,#530,.T.) ;
#18052=EDGE_CURVE('',#13969,#14271,#7963,.T.) ;
#18053=EDGE_CURVE('',#13971,#14271,#531,.T.) ;
#18054=EDGE_CURVE('',#14271,#13970,#532,.T.) ;
#18055=EDGE_CURVE('',#13972,#14272,#7964,.T.) ;
#18056=EDGE_CURVE('',#13974,#14272,#533,.T.) ;
#18057=EDGE_CURVE('',#14272,#13973,#534,.T.) ;
#18058=EDGE_CURVE('',#13975,#14273,#7965,.T.) ;
#18059=EDGE_CURVE('',#13977,#14273,#535,.T.) ;
#18060=EDGE_CURVE('',#14273,#13976,#536,.T.) ;
#18061=EDGE_CURVE('',#13978,#14274,#7966,.T.) ;
#18062=EDGE_CURVE('',#13980,#14274,#537,.T.) ;
#18063=EDGE_CURVE('',#14274,#13979,#538,.T.) ;
#18064=EDGE_CURVE('',#13983,#14275,#7967,.T.) ;
#18065=EDGE_CURVE('',#13985,#14275,#539,.T.) ;
#18066=EDGE_CURVE('',#14275,#13984,#540,.T.) ;
#18067=EDGE_CURVE('',#13986,#14276,#7968,.T.) ;
#18068=EDGE_CURVE('',#13988,#14276,#541,.T.) ;
#18069=EDGE_CURVE('',#14276,#13987,#542,.T.) ;
#18070=EDGE_CURVE('',#13989,#14277,#7969,.T.) ;
#18071=EDGE_CURVE('',#13991,#14277,#543,.T.) ;
#18072=EDGE_CURVE('',#14277,#13990,#544,.T.) ;
#18073=EDGE_CURVE('',#13992,#14278,#7970,.T.) ;
#18074=EDGE_CURVE('',#13994,#14278,#545,.T.) ;
#18075=EDGE_CURVE('',#14278,#13993,#546,.T.) ;
#18076=EDGE_CURVE('',#13997,#14279,#7971,.T.) ;
#18077=EDGE_CURVE('',#13999,#14279,#547,.T.) ;
#18078=EDGE_CURVE('',#14279,#13998,#548,.T.) ;
#18079=EDGE_CURVE('',#14000,#14280,#7972,.T.) ;
#18080=EDGE_CURVE('',#14002,#14280,#549,.T.) ;
#18081=EDGE_CURVE('',#14280,#14001,#550,.T.) ;
#18082=EDGE_CURVE('',#14003,#14281,#7973,.T.) ;
#18083=EDGE_CURVE('',#14005,#14281,#551,.T.) ;
#18084=EDGE_CURVE('',#14281,#14004,#552,.T.) ;
#18085=EDGE_CURVE('',#14006,#14282,#7974,.T.) ;
#18086=EDGE_CURVE('',#14008,#14282,#553,.T.) ;
#18087=EDGE_CURVE('',#14282,#14007,#554,.T.) ;
#18088=EDGE_CURVE('',#14011,#14283,#7975,.T.) ;
#18089=EDGE_CURVE('',#14013,#14283,#555,.T.) ;
#18090=EDGE_CURVE('',#14283,#14012,#556,.T.) ;
#18091=EDGE_CURVE('',#14014,#14284,#7976,.T.) ;
#18092=EDGE_CURVE('',#14016,#14284,#557,.T.) ;
#18093=EDGE_CURVE('',#14284,#14015,#558,.T.) ;
#18094=EDGE_CURVE('',#14017,#14285,#7977,.T.) ;
#18095=EDGE_CURVE('',#14019,#14285,#559,.T.) ;
#18096=EDGE_CURVE('',#14285,#14018,#560,.T.) ;
#18097=EDGE_CURVE('',#14020,#14286,#7978,.T.) ;
#18098=EDGE_CURVE('',#14022,#14286,#561,.T.) ;
#18099=EDGE_CURVE('',#14286,#14021,#562,.T.) ;
#18100=EDGE_CURVE('',#14025,#14287,#7979,.T.) ;
#18101=EDGE_CURVE('',#14027,#14287,#563,.T.) ;
#18102=EDGE_CURVE('',#14287,#14026,#564,.T.) ;
#18103=EDGE_CURVE('',#14028,#14288,#7980,.T.) ;
#18104=EDGE_CURVE('',#14030,#14288,#565,.T.) ;
#18105=EDGE_CURVE('',#14288,#14029,#566,.T.) ;
#18106=EDGE_CURVE('',#14031,#14289,#7981,.T.) ;
#18107=EDGE_CURVE('',#14033,#14289,#567,.T.) ;
#18108=EDGE_CURVE('',#14289,#14032,#568,.T.) ;
#18109=EDGE_CURVE('',#14034,#14290,#7982,.T.) ;
#18110=EDGE_CURVE('',#14036,#14290,#569,.T.) ;
#18111=EDGE_CURVE('',#14290,#14035,#570,.T.) ;
#18112=EDGE_CURVE('',#14039,#14291,#7983,.T.) ;
#18113=EDGE_CURVE('',#14041,#14291,#571,.T.) ;
#18114=EDGE_CURVE('',#14291,#14040,#572,.T.) ;
#18115=EDGE_CURVE('',#14042,#14292,#7984,.T.) ;
#18116=EDGE_CURVE('',#14044,#14292,#573,.T.) ;
#18117=EDGE_CURVE('',#14292,#14043,#574,.T.) ;
#18118=EDGE_CURVE('',#14045,#14293,#7985,.T.) ;
#18119=EDGE_CURVE('',#14047,#14293,#575,.T.) ;
#18120=EDGE_CURVE('',#14293,#14046,#576,.T.) ;
#18121=EDGE_CURVE('',#14048,#14294,#7986,.T.) ;
#18122=EDGE_CURVE('',#14050,#14294,#577,.T.) ;
#18123=EDGE_CURVE('',#14294,#14049,#578,.T.) ;
#18124=EDGE_CURVE('',#14053,#14295,#7987,.T.) ;
#18125=EDGE_CURVE('',#14055,#14295,#579,.T.) ;
#18126=EDGE_CURVE('',#14295,#14054,#580,.T.) ;
#18127=EDGE_CURVE('',#14056,#14296,#7988,.T.) ;
#18128=EDGE_CURVE('',#14058,#14296,#581,.T.) ;
#18129=EDGE_CURVE('',#14296,#14057,#582,.T.) ;
#18130=EDGE_CURVE('',#14059,#14297,#7989,.T.) ;
#18131=EDGE_CURVE('',#14061,#14297,#583,.T.) ;
#18132=EDGE_CURVE('',#14297,#14060,#584,.T.) ;
#18133=EDGE_CURVE('',#14062,#14298,#7990,.T.) ;
#18134=EDGE_CURVE('',#14064,#14298,#585,.T.) ;
#18135=EDGE_CURVE('',#14298,#14063,#586,.T.) ;
#18136=EDGE_CURVE('',#14067,#14299,#7991,.T.) ;
#18137=EDGE_CURVE('',#14069,#14299,#587,.T.) ;
#18138=EDGE_CURVE('',#14299,#14068,#588,.T.) ;
#18139=EDGE_CURVE('',#14070,#14300,#7992,.T.) ;
#18140=EDGE_CURVE('',#14072,#14300,#589,.T.) ;
#18141=EDGE_CURVE('',#14300,#14071,#590,.T.) ;
#18142=EDGE_CURVE('',#14073,#14301,#7993,.T.) ;
#18143=EDGE_CURVE('',#14075,#14301,#591,.T.) ;
#18144=EDGE_CURVE('',#14301,#14074,#592,.T.) ;
#18145=EDGE_CURVE('',#14076,#14302,#7994,.T.) ;
#18146=EDGE_CURVE('',#14078,#14302,#593,.T.) ;
#18147=EDGE_CURVE('',#14302,#14077,#594,.T.) ;
#18148=EDGE_CURVE('',#14081,#14303,#7995,.T.) ;
#18149=EDGE_CURVE('',#14083,#14303,#595,.T.) ;
#18150=EDGE_CURVE('',#14303,#14082,#596,.T.) ;
#18151=EDGE_CURVE('',#14084,#14304,#7996,.T.) ;
#18152=EDGE_CURVE('',#14086,#14304,#597,.T.) ;
#18153=EDGE_CURVE('',#14304,#14085,#598,.T.) ;
#18154=EDGE_CURVE('',#14087,#14305,#7997,.T.) ;
#18155=EDGE_CURVE('',#14089,#14305,#599,.T.) ;
#18156=EDGE_CURVE('',#14305,#14088,#600,.T.) ;
#18157=EDGE_CURVE('',#14090,#14306,#7998,.T.) ;
#18158=EDGE_CURVE('',#14092,#14306,#601,.T.) ;
#18159=EDGE_CURVE('',#14306,#14091,#602,.T.) ;
#18160=EDGE_CURVE('',#14095,#14307,#7999,.T.) ;
#18161=EDGE_CURVE('',#14097,#14307,#603,.T.) ;
#18162=EDGE_CURVE('',#14307,#14096,#604,.T.) ;
#18163=EDGE_CURVE('',#14098,#14308,#8000,.T.) ;
#18164=EDGE_CURVE('',#14100,#14308,#605,.T.) ;
#18165=EDGE_CURVE('',#14308,#14099,#606,.T.) ;
#18166=EDGE_CURVE('',#14101,#14309,#8001,.T.) ;
#18167=EDGE_CURVE('',#14103,#14309,#607,.T.) ;
#18168=EDGE_CURVE('',#14309,#14102,#608,.T.) ;
#18169=EDGE_CURVE('',#14104,#14310,#8002,.T.) ;
#18170=EDGE_CURVE('',#14106,#14310,#609,.T.) ;
#18171=EDGE_CURVE('',#14310,#14105,#610,.T.) ;
#18172=EDGE_CURVE('',#14109,#14311,#8003,.T.) ;
#18173=EDGE_CURVE('',#14111,#14311,#611,.T.) ;
#18174=EDGE_CURVE('',#14311,#14110,#612,.T.) ;
#18175=EDGE_CURVE('',#14112,#14312,#8004,.T.) ;
#18176=EDGE_CURVE('',#14114,#14312,#613,.T.) ;
#18177=EDGE_CURVE('',#14312,#14113,#614,.T.) ;
#18178=EDGE_CURVE('',#14115,#14313,#8005,.T.) ;
#18179=EDGE_CURVE('',#14117,#14313,#615,.T.) ;
#18180=EDGE_CURVE('',#14313,#14116,#616,.T.) ;
#18181=EDGE_CURVE('',#14118,#14314,#8006,.T.) ;
#18182=EDGE_CURVE('',#14120,#14314,#617,.T.) ;
#18183=EDGE_CURVE('',#14314,#14119,#618,.T.) ;
#18184=EDGE_CURVE('',#14123,#14315,#8007,.T.) ;
#18185=EDGE_CURVE('',#14125,#14315,#619,.T.) ;
#18186=EDGE_CURVE('',#14315,#14124,#620,.T.) ;
#18187=EDGE_CURVE('',#14126,#14316,#8008,.T.) ;
#18188=EDGE_CURVE('',#14128,#14316,#621,.T.) ;
#18189=EDGE_CURVE('',#14316,#14127,#622,.T.) ;
#18190=EDGE_CURVE('',#14129,#14317,#8009,.T.) ;
#18191=EDGE_CURVE('',#14131,#14317,#623,.T.) ;
#18192=EDGE_CURVE('',#14317,#14130,#624,.T.) ;
#18193=EDGE_CURVE('',#14132,#14318,#8010,.T.) ;
#18194=EDGE_CURVE('',#14134,#14318,#625,.T.) ;
#18195=EDGE_CURVE('',#14318,#14133,#626,.T.) ;
#18196=EDGE_CURVE('',#14137,#14319,#8011,.T.) ;
#18197=EDGE_CURVE('',#14139,#14319,#627,.T.) ;
#18198=EDGE_CURVE('',#14319,#14138,#628,.T.) ;
#18199=EDGE_CURVE('',#14140,#14320,#8012,.T.) ;
#18200=EDGE_CURVE('',#14142,#14320,#629,.T.) ;
#18201=EDGE_CURVE('',#14320,#14141,#630,.T.) ;
#18202=EDGE_CURVE('',#14143,#14321,#8013,.T.) ;
#18203=EDGE_CURVE('',#14145,#14321,#631,.T.) ;
#18204=EDGE_CURVE('',#14321,#14144,#632,.T.) ;
#18205=EDGE_CURVE('',#14146,#14322,#8014,.T.) ;
#18206=EDGE_CURVE('',#14148,#14322,#633,.T.) ;
#18207=EDGE_CURVE('',#14322,#14147,#634,.T.) ;
#18208=EDGE_CURVE('',#14151,#14323,#8015,.T.) ;
#18209=EDGE_CURVE('',#14153,#14323,#635,.T.) ;
#18210=EDGE_CURVE('',#14323,#14152,#636,.T.) ;
#18211=EDGE_CURVE('',#14154,#14324,#8016,.T.) ;
#18212=EDGE_CURVE('',#14156,#14324,#637,.T.) ;
#18213=EDGE_CURVE('',#14324,#14155,#638,.T.) ;
#18214=EDGE_CURVE('',#14157,#14325,#8017,.T.) ;
#18215=EDGE_CURVE('',#14159,#14325,#639,.T.) ;
#18216=EDGE_CURVE('',#14325,#14158,#640,.T.) ;
#18217=EDGE_CURVE('',#14160,#14326,#8018,.T.) ;
#18218=EDGE_CURVE('',#14162,#14326,#641,.T.) ;
#18219=EDGE_CURVE('',#14326,#14161,#642,.T.) ;
#18220=EDGE_CURVE('',#14165,#14327,#8019,.T.) ;
#18221=EDGE_CURVE('',#14167,#14327,#643,.T.) ;
#18222=EDGE_CURVE('',#14327,#14166,#644,.T.) ;
#18223=EDGE_CURVE('',#14168,#14328,#8020,.T.) ;
#18224=EDGE_CURVE('',#14170,#14328,#645,.T.) ;
#18225=EDGE_CURVE('',#14328,#14169,#646,.T.) ;
#18226=EDGE_CURVE('',#14171,#14329,#8021,.T.) ;
#18227=EDGE_CURVE('',#14173,#14329,#647,.T.) ;
#18228=EDGE_CURVE('',#14329,#14172,#648,.T.) ;
#18229=EDGE_CURVE('',#14174,#14330,#8022,.T.) ;
#18230=EDGE_CURVE('',#14176,#14330,#649,.T.) ;
#18231=EDGE_CURVE('',#14330,#14175,#650,.T.) ;
#18232=EDGE_CURVE('',#14179,#14331,#8023,.T.) ;
#18233=EDGE_CURVE('',#14181,#14331,#651,.T.) ;
#18234=EDGE_CURVE('',#14331,#14180,#652,.T.) ;
#18235=EDGE_CURVE('',#14182,#14332,#8024,.T.) ;
#18236=EDGE_CURVE('',#14184,#14332,#653,.T.) ;
#18237=EDGE_CURVE('',#14332,#14183,#654,.T.) ;
#18238=EDGE_CURVE('',#14185,#14333,#8025,.T.) ;
#18239=EDGE_CURVE('',#14187,#14333,#655,.T.) ;
#18240=EDGE_CURVE('',#14333,#14186,#656,.T.) ;
#18241=EDGE_CURVE('',#14188,#14334,#8026,.T.) ;
#18242=EDGE_CURVE('',#14190,#14334,#657,.T.) ;
#18243=EDGE_CURVE('',#14334,#14189,#658,.T.) ;
#18244=EDGE_CURVE('',#14193,#14335,#8027,.T.) ;
#18245=EDGE_CURVE('',#14195,#14335,#659,.T.) ;
#18246=EDGE_CURVE('',#14335,#14194,#660,.T.) ;
#18247=EDGE_CURVE('',#14196,#14336,#8028,.T.) ;
#18248=EDGE_CURVE('',#14198,#14336,#661,.T.) ;
#18249=EDGE_CURVE('',#14336,#14197,#662,.T.) ;
#18250=EDGE_CURVE('',#14199,#14337,#8029,.T.) ;
#18251=EDGE_CURVE('',#14201,#14337,#663,.T.) ;
#18252=EDGE_CURVE('',#14337,#14200,#664,.T.) ;
#18253=EDGE_CURVE('',#14202,#14338,#8030,.T.) ;
#18254=EDGE_CURVE('',#14204,#14338,#665,.T.) ;
#18255=EDGE_CURVE('',#14338,#14203,#666,.T.) ;
#18256=EDGE_CURVE('',#14207,#14339,#8031,.T.) ;
#18257=EDGE_CURVE('',#14209,#14339,#667,.T.) ;
#18258=EDGE_CURVE('',#14339,#14208,#668,.T.) ;
#18259=EDGE_CURVE('',#14210,#14340,#8032,.T.) ;
#18260=EDGE_CURVE('',#14212,#14340,#669,.T.) ;
#18261=EDGE_CURVE('',#14340,#14211,#670,.T.) ;
#18262=EDGE_CURVE('',#14213,#14341,#8033,.T.) ;
#18263=EDGE_CURVE('',#14215,#14341,#671,.T.) ;
#18264=EDGE_CURVE('',#14341,#14214,#672,.T.) ;
#18265=EDGE_CURVE('',#14216,#14342,#8034,.T.) ;
#18266=EDGE_CURVE('',#14342,#14342,#11753,.T.) ;
#18267=EDGE_CURVE('',#14343,#14343,#11754,.T.) ;
#18268=EDGE_CURVE('',#14343,#14344,#8035,.T.) ;
#18269=EDGE_CURVE('',#14345,#14344,#33,.T.) ;
#18270=EDGE_CURVE('',#14345,#14346,#8036,.T.) ;
#18271=EDGE_CURVE('',#14346,#14346,#11755,.T.) ;
#18272=EDGE_CURVE('',#14347,#14345,#34,.T.) ;
#18273=EDGE_CURVE('',#14344,#14347,#35,.T.) ;
#18274=EDGE_CURVE('',#14348,#14348,#11756,.T.) ;
#18275=EDGE_CURVE('',#14348,#14349,#8037,.T.) ;
#18276=EDGE_CURVE('',#14349,#14349,#11757,.T.) ;
#18277=EDGE_CURVE('',#14345,#14350,#8038,.T.) ;
#18278=EDGE_CURVE('',#14350,#14350,#11758,.T.) ;
#24295=ORIENTED_EDGE('',*,*,#17413,.F.) ;
#24296=ORIENTED_EDGE('',*,*,#17414,.T.) ;
#24297=ORIENTED_EDGE('',*,*,#17415,.F.) ;
#24298=ORIENTED_EDGE('',*,*,#17414,.F.) ;
#24299=ORIENTED_EDGE('',*,*,#17416,.F.) ;
#24300=ORIENTED_EDGE('',*,*,#17417,.F.) ;
#24301=ORIENTED_EDGE('',*,*,#17418,.F.) ;
#24302=ORIENTED_EDGE('',*,*,#17419,.T.) ;
#24303=ORIENTED_EDGE('',*,*,#17420,.F.) ;
#24304=ORIENTED_EDGE('',*,*,#17419,.F.) ;
#24305=ORIENTED_EDGE('',*,*,#17415,.T.) ;
#24306=ORIENTED_EDGE('',*,*,#17418,.T.) ;
#24307=ORIENTED_EDGE('',*,*,#17413,.T.) ;
#24308=ORIENTED_EDGE('',*,*,#17420,.T.) ;
#24309=ORIENTED_EDGE('',*,*,#17421,.F.) ;
#24310=ORIENTED_EDGE('',*,*,#17422,.T.) ;
#24311=ORIENTED_EDGE('',*,*,#17417,.T.) ;
#24312=ORIENTED_EDGE('',*,*,#17416,.T.) ;
#24313=ORIENTED_EDGE('',*,*,#17422,.F.) ;
#24314=ORIENTED_EDGE('',*,*,#17421,.T.) ;
#24315=ORIENTED_EDGE('',*,*,#17423,.F.) ;
#24316=ORIENTED_EDGE('',*,*,#17424,.T.) ;
#24317=ORIENTED_EDGE('',*,*,#17425,.F.) ;
#24318=ORIENTED_EDGE('',*,*,#17424,.F.) ;
#24319=ORIENTED_EDGE('',*,*,#17426,.F.) ;
#24320=ORIENTED_EDGE('',*,*,#17427,.T.) ;
#24321=ORIENTED_EDGE('',*,*,#17428,.F.) ;
#24322=ORIENTED_EDGE('',*,*,#17427,.F.) ;
#24323=ORIENTED_EDGE('',*,*,#17428,.T.) ;
#24324=ORIENTED_EDGE('',*,*,#17423,.T.) ;
#24325=ORIENTED_EDGE('',*,*,#17426,.T.) ;
#24326=ORIENTED_EDGE('',*,*,#17425,.T.) ;
#24327=ORIENTED_EDGE('',*,*,#17429,.F.) ;
#24328=ORIENTED_EDGE('',*,*,#17430,.F.) ;
#24329=ORIENTED_EDGE('',*,*,#17431,.F.) ;
#24330=ORIENTED_EDGE('',*,*,#17432,.F.) ;
#24331=ORIENTED_EDGE('',*,*,#17433,.F.) ;
#24332=ORIENTED_EDGE('',*,*,#17434,.T.) ;
#24333=ORIENTED_EDGE('',*,*,#17435,.F.) ;
#24334=ORIENTED_EDGE('',*,*,#17434,.F.) ;
#24335=ORIENTED_EDGE('',*,*,#17436,.F.) ;
#24336=ORIENTED_EDGE('',*,*,#17437,.T.) ;
#24337=ORIENTED_EDGE('',*,*,#17438,.F.) ;
#24338=ORIENTED_EDGE('',*,*,#17437,.F.) ;
#24339=ORIENTED_EDGE('',*,*,#17438,.T.) ;
#24340=ORIENTED_EDGE('',*,*,#17439,.F.) ;
#24341=ORIENTED_EDGE('',*,*,#17433,.T.) ;
#24342=ORIENTED_EDGE('',*,*,#17440,.F.) ;
#24343=ORIENTED_EDGE('',*,*,#17441,.F.) ;
#24344=ORIENTED_EDGE('',*,*,#17442,.F.) ;
#24345=ORIENTED_EDGE('',*,*,#17443,.F.) ;
#24346=ORIENTED_EDGE('',*,*,#17444,.F.) ;
#24347=ORIENTED_EDGE('',*,*,#17436,.T.) ;
#24348=ORIENTED_EDGE('',*,*,#17435,.T.) ;
#24349=ORIENTED_EDGE('',*,*,#17429,.T.) ;
#24350=ORIENTED_EDGE('',*,*,#17439,.T.) ;
#24351=ORIENTED_EDGE('',*,*,#17445,.T.) ;
#24352=ORIENTED_EDGE('',*,*,#17443,.T.) ;
#24353=ORIENTED_EDGE('',*,*,#17446,.T.) ;
#24354=ORIENTED_EDGE('',*,*,#17447,.T.) ;
#24355=ORIENTED_EDGE('',*,*,#17441,.T.) ;
#24356=ORIENTED_EDGE('',*,*,#17448,.T.) ;
#24357=ORIENTED_EDGE('',*,*,#17449,.T.) ;
#24358=ORIENTED_EDGE('',*,*,#17450,.T.) ;
#24359=ORIENTED_EDGE('',*,*,#17451,.T.) ;
#24360=ORIENTED_EDGE('',*,*,#17452,.T.) ;
#24361=ORIENTED_EDGE('',*,*,#17453,.T.) ;
#24362=ORIENTED_EDGE('',*,*,#17454,.T.) ;
#24363=ORIENTED_EDGE('',*,*,#17455,.T.) ;
#24364=ORIENTED_EDGE('',*,*,#17456,.T.) ;
#24365=ORIENTED_EDGE('',*,*,#17456,.F.) ;
#24366=ORIENTED_EDGE('',*,*,#17457,.T.) ;
#24367=ORIENTED_EDGE('',*,*,#17458,.T.) ;
#24368=ORIENTED_EDGE('',*,*,#17459,.T.) ;
#24369=ORIENTED_EDGE('',*,*,#17460,.T.) ;
#24370=ORIENTED_EDGE('',*,*,#17461,.T.) ;
#24371=ORIENTED_EDGE('',*,*,#17462,.T.) ;
#24372=ORIENTED_EDGE('',*,*,#17463,.T.) ;
#24373=ORIENTED_EDGE('',*,*,#17464,.T.) ;
#24374=ORIENTED_EDGE('',*,*,#17465,.T.) ;
#24375=ORIENTED_EDGE('',*,*,#17466,.T.) ;
#24376=ORIENTED_EDGE('',*,*,#17467,.T.) ;
#24377=ORIENTED_EDGE('',*,*,#17468,.T.) ;
#24378=ORIENTED_EDGE('',*,*,#17469,.T.) ;
#24379=ORIENTED_EDGE('',*,*,#17470,.F.) ;
#24380=ORIENTED_EDGE('',*,*,#17470,.T.) ;
#24381=ORIENTED_EDGE('',*,*,#17471,.T.) ;
#24382=ORIENTED_EDGE('',*,*,#17472,.T.) ;
#24383=ORIENTED_EDGE('',*,*,#17473,.T.) ;
#24384=ORIENTED_EDGE('',*,*,#17474,.T.) ;
#24385=ORIENTED_EDGE('',*,*,#17475,.T.) ;
#24386=ORIENTED_EDGE('',*,*,#17476,.T.) ;
#24387=ORIENTED_EDGE('',*,*,#17477,.T.) ;
#24388=ORIENTED_EDGE('',*,*,#17478,.T.) ;
#24389=ORIENTED_EDGE('',*,*,#17479,.T.) ;
#24390=ORIENTED_EDGE('',*,*,#17480,.T.) ;
#24391=ORIENTED_EDGE('',*,*,#17481,.T.) ;
#24392=ORIENTED_EDGE('',*,*,#17482,.T.) ;
#24393=ORIENTED_EDGE('',*,*,#17483,.T.) ;
#24394=ORIENTED_EDGE('',*,*,#17484,.T.) ;
#24395=ORIENTED_EDGE('',*,*,#17484,.F.) ;
#24396=ORIENTED_EDGE('',*,*,#17485,.T.) ;
#24397=ORIENTED_EDGE('',*,*,#17486,.T.) ;
#24398=ORIENTED_EDGE('',*,*,#17487,.T.) ;
#24399=ORIENTED_EDGE('',*,*,#17488,.T.) ;
#24400=ORIENTED_EDGE('',*,*,#17489,.T.) ;
#24401=ORIENTED_EDGE('',*,*,#17490,.T.) ;
#24402=ORIENTED_EDGE('',*,*,#17491,.T.) ;
#24403=ORIENTED_EDGE('',*,*,#17492,.T.) ;
#24404=ORIENTED_EDGE('',*,*,#17493,.T.) ;
#24405=ORIENTED_EDGE('',*,*,#17494,.T.) ;
#24406=ORIENTED_EDGE('',*,*,#17495,.T.) ;
#24407=ORIENTED_EDGE('',*,*,#17496,.T.) ;
#24408=ORIENTED_EDGE('',*,*,#17497,.T.) ;
#24409=ORIENTED_EDGE('',*,*,#17498,.F.) ;
#24410=ORIENTED_EDGE('',*,*,#17498,.T.) ;
#24411=ORIENTED_EDGE('',*,*,#17499,.T.) ;
#24412=ORIENTED_EDGE('',*,*,#17500,.T.) ;
#24413=ORIENTED_EDGE('',*,*,#17501,.T.) ;
#24414=ORIENTED_EDGE('',*,*,#17502,.T.) ;
#24415=ORIENTED_EDGE('',*,*,#17503,.T.) ;
#24416=ORIENTED_EDGE('',*,*,#17504,.T.) ;
#24417=ORIENTED_EDGE('',*,*,#17505,.T.) ;
#24418=ORIENTED_EDGE('',*,*,#17506,.T.) ;
#24419=ORIENTED_EDGE('',*,*,#17507,.T.) ;
#24420=ORIENTED_EDGE('',*,*,#17508,.T.) ;
#24421=ORIENTED_EDGE('',*,*,#17509,.T.) ;
#24422=ORIENTED_EDGE('',*,*,#17510,.T.) ;
#24423=ORIENTED_EDGE('',*,*,#17511,.T.) ;
#24424=ORIENTED_EDGE('',*,*,#17512,.T.) ;
#24425=ORIENTED_EDGE('',*,*,#17512,.F.) ;
#24426=ORIENTED_EDGE('',*,*,#17513,.T.) ;
#24427=ORIENTED_EDGE('',*,*,#17514,.T.) ;
#24428=ORIENTED_EDGE('',*,*,#17515,.T.) ;
#24429=ORIENTED_EDGE('',*,*,#17516,.T.) ;
#24430=ORIENTED_EDGE('',*,*,#17517,.T.) ;
#24431=ORIENTED_EDGE('',*,*,#17518,.T.) ;
#24432=ORIENTED_EDGE('',*,*,#17519,.T.) ;
#24433=ORIENTED_EDGE('',*,*,#17520,.T.) ;
#24434=ORIENTED_EDGE('',*,*,#17521,.T.) ;
#24435=ORIENTED_EDGE('',*,*,#17522,.T.) ;
#24436=ORIENTED_EDGE('',*,*,#17523,.T.) ;
#24437=ORIENTED_EDGE('',*,*,#17524,.T.) ;
#24438=ORIENTED_EDGE('',*,*,#17525,.T.) ;
#24439=ORIENTED_EDGE('',*,*,#17526,.F.) ;
#24440=ORIENTED_EDGE('',*,*,#17526,.T.) ;
#24441=ORIENTED_EDGE('',*,*,#17527,.T.) ;
#24442=ORIENTED_EDGE('',*,*,#17528,.T.) ;
#24443=ORIENTED_EDGE('',*,*,#17529,.T.) ;
#24444=ORIENTED_EDGE('',*,*,#17530,.T.) ;
#24445=ORIENTED_EDGE('',*,*,#17531,.T.) ;
#24446=ORIENTED_EDGE('',*,*,#17532,.T.) ;
#24447=ORIENTED_EDGE('',*,*,#17533,.T.) ;
#24448=ORIENTED_EDGE('',*,*,#17534,.T.) ;
#24449=ORIENTED_EDGE('',*,*,#17535,.T.) ;
#24450=ORIENTED_EDGE('',*,*,#17536,.T.) ;
#24451=ORIENTED_EDGE('',*,*,#17537,.T.) ;
#24452=ORIENTED_EDGE('',*,*,#17538,.T.) ;
#24453=ORIENTED_EDGE('',*,*,#17539,.T.) ;
#24454=ORIENTED_EDGE('',*,*,#17540,.T.) ;
#24455=ORIENTED_EDGE('',*,*,#17540,.F.) ;
#24456=ORIENTED_EDGE('',*,*,#17541,.T.) ;
#24457=ORIENTED_EDGE('',*,*,#17542,.T.) ;
#24458=ORIENTED_EDGE('',*,*,#17543,.T.) ;
#24459=ORIENTED_EDGE('',*,*,#17544,.T.) ;
#24460=ORIENTED_EDGE('',*,*,#17545,.T.) ;
#24461=ORIENTED_EDGE('',*,*,#17546,.T.) ;
#24462=ORIENTED_EDGE('',*,*,#17547,.T.) ;
#24463=ORIENTED_EDGE('',*,*,#17548,.T.) ;
#24464=ORIENTED_EDGE('',*,*,#17549,.T.) ;
#24465=ORIENTED_EDGE('',*,*,#17550,.T.) ;
#24466=ORIENTED_EDGE('',*,*,#17551,.T.) ;
#24467=ORIENTED_EDGE('',*,*,#17552,.T.) ;
#24468=ORIENTED_EDGE('',*,*,#17553,.T.) ;
#24469=ORIENTED_EDGE('',*,*,#17554,.F.) ;
#24470=ORIENTED_EDGE('',*,*,#17554,.T.) ;
#24471=ORIENTED_EDGE('',*,*,#17555,.T.) ;
#24472=ORIENTED_EDGE('',*,*,#17556,.T.) ;
#24473=ORIENTED_EDGE('',*,*,#17557,.T.) ;
#24474=ORIENTED_EDGE('',*,*,#17558,.T.) ;
#24475=ORIENTED_EDGE('',*,*,#17559,.T.) ;
#24476=ORIENTED_EDGE('',*,*,#17560,.T.) ;
#24477=ORIENTED_EDGE('',*,*,#17561,.T.) ;
#24478=ORIENTED_EDGE('',*,*,#17562,.T.) ;
#24479=ORIENTED_EDGE('',*,*,#17563,.T.) ;
#24480=ORIENTED_EDGE('',*,*,#17564,.T.) ;
#24481=ORIENTED_EDGE('',*,*,#17565,.T.) ;
#24482=ORIENTED_EDGE('',*,*,#17566,.T.) ;
#24483=ORIENTED_EDGE('',*,*,#17567,.T.) ;
#24484=ORIENTED_EDGE('',*,*,#17568,.T.) ;
#24485=ORIENTED_EDGE('',*,*,#17568,.F.) ;
#24486=ORIENTED_EDGE('',*,*,#17569,.T.) ;
#24487=ORIENTED_EDGE('',*,*,#17570,.T.) ;
#24488=ORIENTED_EDGE('',*,*,#17571,.T.) ;
#24489=ORIENTED_EDGE('',*,*,#17572,.T.) ;
#24490=ORIENTED_EDGE('',*,*,#17573,.T.) ;
#24491=ORIENTED_EDGE('',*,*,#17574,.T.) ;
#24492=ORIENTED_EDGE('',*,*,#17575,.T.) ;
#24493=ORIENTED_EDGE('',*,*,#17576,.T.) ;
#24494=ORIENTED_EDGE('',*,*,#17577,.T.) ;
#24495=ORIENTED_EDGE('',*,*,#17578,.T.) ;
#24496=ORIENTED_EDGE('',*,*,#17579,.T.) ;
#24497=ORIENTED_EDGE('',*,*,#17580,.T.) ;
#24498=ORIENTED_EDGE('',*,*,#17581,.T.) ;
#24499=ORIENTED_EDGE('',*,*,#17582,.F.) ;
#24500=ORIENTED_EDGE('',*,*,#17582,.T.) ;
#24501=ORIENTED_EDGE('',*,*,#17583,.T.) ;
#24502=ORIENTED_EDGE('',*,*,#17584,.T.) ;
#24503=ORIENTED_EDGE('',*,*,#17585,.T.) ;
#24504=ORIENTED_EDGE('',*,*,#17586,.T.) ;
#24505=ORIENTED_EDGE('',*,*,#17587,.T.) ;
#24506=ORIENTED_EDGE('',*,*,#17588,.T.) ;
#24507=ORIENTED_EDGE('',*,*,#17589,.T.) ;
#24508=ORIENTED_EDGE('',*,*,#17590,.T.) ;
#24509=ORIENTED_EDGE('',*,*,#17591,.T.) ;
#24510=ORIENTED_EDGE('',*,*,#17592,.T.) ;
#24511=ORIENTED_EDGE('',*,*,#17593,.T.) ;
#24512=ORIENTED_EDGE('',*,*,#17594,.T.) ;
#24513=ORIENTED_EDGE('',*,*,#17595,.T.) ;
#24514=ORIENTED_EDGE('',*,*,#17596,.T.) ;
#24515=ORIENTED_EDGE('',*,*,#17596,.F.) ;
#24516=ORIENTED_EDGE('',*,*,#17597,.T.) ;
#24517=ORIENTED_EDGE('',*,*,#17598,.T.) ;
#24518=ORIENTED_EDGE('',*,*,#17599,.T.) ;
#24519=ORIENTED_EDGE('',*,*,#17600,.T.) ;
#24520=ORIENTED_EDGE('',*,*,#17601,.T.) ;
#24521=ORIENTED_EDGE('',*,*,#17602,.T.) ;
#24522=ORIENTED_EDGE('',*,*,#17603,.T.) ;
#24523=ORIENTED_EDGE('',*,*,#17604,.T.) ;
#24524=ORIENTED_EDGE('',*,*,#17605,.T.) ;
#24525=ORIENTED_EDGE('',*,*,#17606,.T.) ;
#24526=ORIENTED_EDGE('',*,*,#17607,.T.) ;
#24527=ORIENTED_EDGE('',*,*,#17608,.T.) ;
#24528=ORIENTED_EDGE('',*,*,#17609,.T.) ;
#24529=ORIENTED_EDGE('',*,*,#17610,.F.) ;
#24530=ORIENTED_EDGE('',*,*,#17610,.T.) ;
#24531=ORIENTED_EDGE('',*,*,#17611,.T.) ;
#24532=ORIENTED_EDGE('',*,*,#17612,.T.) ;
#24533=ORIENTED_EDGE('',*,*,#17613,.T.) ;
#24534=ORIENTED_EDGE('',*,*,#17614,.T.) ;
#24535=ORIENTED_EDGE('',*,*,#17615,.T.) ;
#24536=ORIENTED_EDGE('',*,*,#17616,.T.) ;
#24537=ORIENTED_EDGE('',*,*,#17617,.T.) ;
#24538=ORIENTED_EDGE('',*,*,#17618,.T.) ;
#24539=ORIENTED_EDGE('',*,*,#17619,.T.) ;
#24540=ORIENTED_EDGE('',*,*,#17620,.T.) ;
#24541=ORIENTED_EDGE('',*,*,#17621,.T.) ;
#24542=ORIENTED_EDGE('',*,*,#17622,.T.) ;
#24543=ORIENTED_EDGE('',*,*,#17623,.T.) ;
#24544=ORIENTED_EDGE('',*,*,#17624,.T.) ;
#24545=ORIENTED_EDGE('',*,*,#17624,.F.) ;
#24546=ORIENTED_EDGE('',*,*,#17625,.T.) ;
#24547=ORIENTED_EDGE('',*,*,#17626,.T.) ;
#24548=ORIENTED_EDGE('',*,*,#17627,.T.) ;
#24549=ORIENTED_EDGE('',*,*,#17628,.T.) ;
#24550=ORIENTED_EDGE('',*,*,#17629,.T.) ;
#24551=ORIENTED_EDGE('',*,*,#17630,.T.) ;
#24552=ORIENTED_EDGE('',*,*,#17631,.T.) ;
#24553=ORIENTED_EDGE('',*,*,#17632,.T.) ;
#24554=ORIENTED_EDGE('',*,*,#17633,.T.) ;
#24555=ORIENTED_EDGE('',*,*,#17634,.T.) ;
#24556=ORIENTED_EDGE('',*,*,#17635,.T.) ;
#24557=ORIENTED_EDGE('',*,*,#17636,.T.) ;
#24558=ORIENTED_EDGE('',*,*,#17637,.T.) ;
#24559=ORIENTED_EDGE('',*,*,#17638,.F.) ;
#24560=ORIENTED_EDGE('',*,*,#17638,.T.) ;
#24561=ORIENTED_EDGE('',*,*,#17639,.T.) ;
#24562=ORIENTED_EDGE('',*,*,#17640,.T.) ;
#24563=ORIENTED_EDGE('',*,*,#17641,.T.) ;
#24564=ORIENTED_EDGE('',*,*,#17642,.T.) ;
#24565=ORIENTED_EDGE('',*,*,#17643,.T.) ;
#24566=ORIENTED_EDGE('',*,*,#17644,.T.) ;
#24567=ORIENTED_EDGE('',*,*,#17645,.T.) ;
#24568=ORIENTED_EDGE('',*,*,#17646,.T.) ;
#24569=ORIENTED_EDGE('',*,*,#17647,.T.) ;
#24570=ORIENTED_EDGE('',*,*,#17648,.T.) ;
#24571=ORIENTED_EDGE('',*,*,#17649,.T.) ;
#24572=ORIENTED_EDGE('',*,*,#17650,.T.) ;
#24573=ORIENTED_EDGE('',*,*,#17651,.T.) ;
#24574=ORIENTED_EDGE('',*,*,#17652,.T.) ;
#24575=ORIENTED_EDGE('',*,*,#17652,.F.) ;
#24576=ORIENTED_EDGE('',*,*,#17653,.T.) ;
#24577=ORIENTED_EDGE('',*,*,#17654,.T.) ;
#24578=ORIENTED_EDGE('',*,*,#17655,.T.) ;
#24579=ORIENTED_EDGE('',*,*,#17656,.T.) ;
#24580=ORIENTED_EDGE('',*,*,#17657,.T.) ;
#24581=ORIENTED_EDGE('',*,*,#17658,.T.) ;
#24582=ORIENTED_EDGE('',*,*,#17659,.T.) ;
#24583=ORIENTED_EDGE('',*,*,#17660,.T.) ;
#24584=ORIENTED_EDGE('',*,*,#17661,.T.) ;
#24585=ORIENTED_EDGE('',*,*,#17662,.T.) ;
#24586=ORIENTED_EDGE('',*,*,#17663,.T.) ;
#24587=ORIENTED_EDGE('',*,*,#17664,.T.) ;
#24588=ORIENTED_EDGE('',*,*,#17665,.T.) ;
#24589=ORIENTED_EDGE('',*,*,#17666,.F.) ;
#24590=ORIENTED_EDGE('',*,*,#17666,.T.) ;
#24591=ORIENTED_EDGE('',*,*,#17667,.T.) ;
#24592=ORIENTED_EDGE('',*,*,#17668,.T.) ;
#24593=ORIENTED_EDGE('',*,*,#17669,.T.) ;
#24594=ORIENTED_EDGE('',*,*,#17670,.T.) ;
#24595=ORIENTED_EDGE('',*,*,#17671,.T.) ;
#24596=ORIENTED_EDGE('',*,*,#17672,.T.) ;
#24597=ORIENTED_EDGE('',*,*,#17673,.T.) ;
#24598=ORIENTED_EDGE('',*,*,#17674,.T.) ;
#24599=ORIENTED_EDGE('',*,*,#17675,.T.) ;
#24600=ORIENTED_EDGE('',*,*,#17676,.T.) ;
#24601=ORIENTED_EDGE('',*,*,#17677,.T.) ;
#24602=ORIENTED_EDGE('',*,*,#17678,.T.) ;
#24603=ORIENTED_EDGE('',*,*,#17679,.T.) ;
#24604=ORIENTED_EDGE('',*,*,#17680,.T.) ;
#24605=ORIENTED_EDGE('',*,*,#17680,.F.) ;
#24606=ORIENTED_EDGE('',*,*,#17681,.T.) ;
#24607=ORIENTED_EDGE('',*,*,#17682,.T.) ;
#24608=ORIENTED_EDGE('',*,*,#17683,.T.) ;
#24609=ORIENTED_EDGE('',*,*,#17684,.T.) ;
#24610=ORIENTED_EDGE('',*,*,#17685,.T.) ;
#24611=ORIENTED_EDGE('',*,*,#17686,.T.) ;
#24612=ORIENTED_EDGE('',*,*,#17687,.T.) ;
#24613=ORIENTED_EDGE('',*,*,#17688,.T.) ;
#24614=ORIENTED_EDGE('',*,*,#17689,.T.) ;
#24615=ORIENTED_EDGE('',*,*,#17690,.T.) ;
#24616=ORIENTED_EDGE('',*,*,#17691,.T.) ;
#24617=ORIENTED_EDGE('',*,*,#17692,.T.) ;
#24618=ORIENTED_EDGE('',*,*,#17693,.T.) ;
#24619=ORIENTED_EDGE('',*,*,#17694,.F.) ;
#24620=ORIENTED_EDGE('',*,*,#17694,.T.) ;
#24621=ORIENTED_EDGE('',*,*,#17695,.T.) ;
#24622=ORIENTED_EDGE('',*,*,#17696,.T.) ;
#24623=ORIENTED_EDGE('',*,*,#17697,.T.) ;
#24624=ORIENTED_EDGE('',*,*,#17698,.T.) ;
#24625=ORIENTED_EDGE('',*,*,#17699,.T.) ;
#24626=ORIENTED_EDGE('',*,*,#17700,.T.) ;
#24627=ORIENTED_EDGE('',*,*,#17701,.T.) ;
#24628=ORIENTED_EDGE('',*,*,#17702,.T.) ;
#24629=ORIENTED_EDGE('',*,*,#17703,.T.) ;
#24630=ORIENTED_EDGE('',*,*,#17704,.T.) ;
#24631=ORIENTED_EDGE('',*,*,#17705,.T.) ;
#24632=ORIENTED_EDGE('',*,*,#17706,.T.) ;
#24633=ORIENTED_EDGE('',*,*,#17707,.T.) ;
#24634=ORIENTED_EDGE('',*,*,#17708,.T.) ;
#24635=ORIENTED_EDGE('',*,*,#17708,.F.) ;
#24636=ORIENTED_EDGE('',*,*,#17709,.T.) ;
#24637=ORIENTED_EDGE('',*,*,#17710,.T.) ;
#24638=ORIENTED_EDGE('',*,*,#17711,.T.) ;
#24639=ORIENTED_EDGE('',*,*,#17712,.T.) ;
#24640=ORIENTED_EDGE('',*,*,#17713,.T.) ;
#24641=ORIENTED_EDGE('',*,*,#17714,.T.) ;
#24642=ORIENTED_EDGE('',*,*,#17715,.T.) ;
#24643=ORIENTED_EDGE('',*,*,#17716,.T.) ;
#24644=ORIENTED_EDGE('',*,*,#17717,.T.) ;
#24645=ORIENTED_EDGE('',*,*,#17718,.T.) ;
#24646=ORIENTED_EDGE('',*,*,#17719,.T.) ;
#24647=ORIENTED_EDGE('',*,*,#17720,.T.) ;
#24648=ORIENTED_EDGE('',*,*,#17721,.T.) ;
#24649=ORIENTED_EDGE('',*,*,#17722,.F.) ;
#24650=ORIENTED_EDGE('',*,*,#17722,.T.) ;
#24651=ORIENTED_EDGE('',*,*,#17723,.T.) ;
#24652=ORIENTED_EDGE('',*,*,#17724,.T.) ;
#24653=ORIENTED_EDGE('',*,*,#17725,.T.) ;
#24654=ORIENTED_EDGE('',*,*,#17726,.T.) ;
#24655=ORIENTED_EDGE('',*,*,#17727,.T.) ;
#24656=ORIENTED_EDGE('',*,*,#17728,.T.) ;
#24657=ORIENTED_EDGE('',*,*,#17729,.T.) ;
#24658=ORIENTED_EDGE('',*,*,#17730,.T.) ;
#24659=ORIENTED_EDGE('',*,*,#17731,.T.) ;
#24660=ORIENTED_EDGE('',*,*,#17732,.T.) ;
#24661=ORIENTED_EDGE('',*,*,#17733,.T.) ;
#24662=ORIENTED_EDGE('',*,*,#17734,.T.) ;
#24663=ORIENTED_EDGE('',*,*,#17735,.T.) ;
#24664=ORIENTED_EDGE('',*,*,#17736,.T.) ;
#24665=ORIENTED_EDGE('',*,*,#17736,.F.) ;
#24666=ORIENTED_EDGE('',*,*,#17737,.T.) ;
#24667=ORIENTED_EDGE('',*,*,#17738,.T.) ;
#24668=ORIENTED_EDGE('',*,*,#17739,.T.) ;
#24669=ORIENTED_EDGE('',*,*,#17740,.T.) ;
#24670=ORIENTED_EDGE('',*,*,#17741,.T.) ;
#24671=ORIENTED_EDGE('',*,*,#17742,.T.) ;
#24672=ORIENTED_EDGE('',*,*,#17743,.T.) ;
#24673=ORIENTED_EDGE('',*,*,#17744,.T.) ;
#24674=ORIENTED_EDGE('',*,*,#17745,.T.) ;
#24675=ORIENTED_EDGE('',*,*,#17746,.T.) ;
#24676=ORIENTED_EDGE('',*,*,#17747,.T.) ;
#24677=ORIENTED_EDGE('',*,*,#17748,.T.) ;
#24678=ORIENTED_EDGE('',*,*,#17749,.T.) ;
#24679=ORIENTED_EDGE('',*,*,#17750,.F.) ;
#24680=ORIENTED_EDGE('',*,*,#17750,.T.) ;
#24681=ORIENTED_EDGE('',*,*,#17751,.T.) ;
#24682=ORIENTED_EDGE('',*,*,#17752,.T.) ;
#24683=ORIENTED_EDGE('',*,*,#17753,.T.) ;
#24684=ORIENTED_EDGE('',*,*,#17754,.T.) ;
#24685=ORIENTED_EDGE('',*,*,#17755,.T.) ;
#24686=ORIENTED_EDGE('',*,*,#17756,.T.) ;
#24687=ORIENTED_EDGE('',*,*,#17757,.T.) ;
#24688=ORIENTED_EDGE('',*,*,#17758,.T.) ;
#24689=ORIENTED_EDGE('',*,*,#17759,.T.) ;
#24690=ORIENTED_EDGE('',*,*,#17760,.T.) ;
#24691=ORIENTED_EDGE('',*,*,#17761,.T.) ;
#24692=ORIENTED_EDGE('',*,*,#17762,.T.) ;
#24693=ORIENTED_EDGE('',*,*,#17763,.T.) ;
#24694=ORIENTED_EDGE('',*,*,#17764,.T.) ;
#24695=ORIENTED_EDGE('',*,*,#17764,.F.) ;
#24696=ORIENTED_EDGE('',*,*,#17765,.T.) ;
#24697=ORIENTED_EDGE('',*,*,#17766,.T.) ;
#24698=ORIENTED_EDGE('',*,*,#17767,.T.) ;
#24699=ORIENTED_EDGE('',*,*,#17768,.T.) ;
#24700=ORIENTED_EDGE('',*,*,#17769,.T.) ;
#24701=ORIENTED_EDGE('',*,*,#17770,.T.) ;
#24702=ORIENTED_EDGE('',*,*,#17771,.T.) ;
#24703=ORIENTED_EDGE('',*,*,#17772,.T.) ;
#24704=ORIENTED_EDGE('',*,*,#17773,.T.) ;
#24705=ORIENTED_EDGE('',*,*,#17774,.T.) ;
#24706=ORIENTED_EDGE('',*,*,#17775,.T.) ;
#24707=ORIENTED_EDGE('',*,*,#17776,.T.) ;
#24708=ORIENTED_EDGE('',*,*,#17777,.T.) ;
#24709=ORIENTED_EDGE('',*,*,#17778,.F.) ;
#24710=ORIENTED_EDGE('',*,*,#17778,.T.) ;
#24711=ORIENTED_EDGE('',*,*,#17779,.T.) ;
#24712=ORIENTED_EDGE('',*,*,#17780,.T.) ;
#24713=ORIENTED_EDGE('',*,*,#17781,.T.) ;
#24714=ORIENTED_EDGE('',*,*,#17782,.T.) ;
#24715=ORIENTED_EDGE('',*,*,#17783,.T.) ;
#24716=ORIENTED_EDGE('',*,*,#17784,.T.) ;
#24717=ORIENTED_EDGE('',*,*,#17785,.T.) ;
#24718=ORIENTED_EDGE('',*,*,#17786,.T.) ;
#24719=ORIENTED_EDGE('',*,*,#17787,.T.) ;
#24720=ORIENTED_EDGE('',*,*,#17788,.T.) ;
#24721=ORIENTED_EDGE('',*,*,#17789,.T.) ;
#24722=ORIENTED_EDGE('',*,*,#17790,.T.) ;
#24723=ORIENTED_EDGE('',*,*,#17791,.T.) ;
#24724=ORIENTED_EDGE('',*,*,#17792,.T.) ;
#24725=ORIENTED_EDGE('',*,*,#17792,.F.) ;
#24726=ORIENTED_EDGE('',*,*,#17793,.T.) ;
#24727=ORIENTED_EDGE('',*,*,#17794,.T.) ;
#24728=ORIENTED_EDGE('',*,*,#17795,.T.) ;
#24729=ORIENTED_EDGE('',*,*,#17796,.T.) ;
#24730=ORIENTED_EDGE('',*,*,#17797,.T.) ;
#24731=ORIENTED_EDGE('',*,*,#17798,.T.) ;
#24732=ORIENTED_EDGE('',*,*,#17799,.T.) ;
#24733=ORIENTED_EDGE('',*,*,#17800,.T.) ;
#24734=ORIENTED_EDGE('',*,*,#17801,.T.) ;
#24735=ORIENTED_EDGE('',*,*,#17802,.T.) ;
#24736=ORIENTED_EDGE('',*,*,#17803,.T.) ;
#24737=ORIENTED_EDGE('',*,*,#17804,.T.) ;
#24738=ORIENTED_EDGE('',*,*,#17805,.T.) ;
#24739=ORIENTED_EDGE('',*,*,#17806,.F.) ;
#24740=ORIENTED_EDGE('',*,*,#17806,.T.) ;
#24741=ORIENTED_EDGE('',*,*,#17807,.T.) ;
#24742=ORIENTED_EDGE('',*,*,#17808,.T.) ;
#24743=ORIENTED_EDGE('',*,*,#17809,.T.) ;
#24744=ORIENTED_EDGE('',*,*,#17810,.T.) ;
#24745=ORIENTED_EDGE('',*,*,#17811,.T.) ;
#24746=ORIENTED_EDGE('',*,*,#17812,.T.) ;
#24747=ORIENTED_EDGE('',*,*,#17813,.T.) ;
#24748=ORIENTED_EDGE('',*,*,#17814,.T.) ;
#24749=ORIENTED_EDGE('',*,*,#17815,.T.) ;
#24750=ORIENTED_EDGE('',*,*,#17816,.T.) ;
#24751=ORIENTED_EDGE('',*,*,#17817,.T.) ;
#24752=ORIENTED_EDGE('',*,*,#17818,.T.) ;
#24753=ORIENTED_EDGE('',*,*,#17819,.T.) ;
#24754=ORIENTED_EDGE('',*,*,#17820,.T.) ;
#24755=ORIENTED_EDGE('',*,*,#17820,.F.) ;
#24756=ORIENTED_EDGE('',*,*,#17821,.T.) ;
#24757=ORIENTED_EDGE('',*,*,#17822,.T.) ;
#24758=ORIENTED_EDGE('',*,*,#17823,.T.) ;
#24759=ORIENTED_EDGE('',*,*,#17824,.T.) ;
#24760=ORIENTED_EDGE('',*,*,#17825,.T.) ;
#24761=ORIENTED_EDGE('',*,*,#17826,.T.) ;
#24762=ORIENTED_EDGE('',*,*,#17827,.T.) ;
#24763=ORIENTED_EDGE('',*,*,#17828,.T.) ;
#24764=ORIENTED_EDGE('',*,*,#17829,.T.) ;
#24765=ORIENTED_EDGE('',*,*,#17830,.T.) ;
#24766=ORIENTED_EDGE('',*,*,#17831,.T.) ;
#24767=ORIENTED_EDGE('',*,*,#17832,.T.) ;
#24768=ORIENTED_EDGE('',*,*,#17833,.T.) ;
#24769=ORIENTED_EDGE('',*,*,#17834,.F.) ;
#24770=ORIENTED_EDGE('',*,*,#17834,.T.) ;
#24771=ORIENTED_EDGE('',*,*,#17835,.T.) ;
#24772=ORIENTED_EDGE('',*,*,#17836,.T.) ;
#24773=ORIENTED_EDGE('',*,*,#17837,.T.) ;
#24774=ORIENTED_EDGE('',*,*,#17838,.T.) ;
#24775=ORIENTED_EDGE('',*,*,#17839,.T.) ;
#24776=ORIENTED_EDGE('',*,*,#17840,.T.) ;
#24777=ORIENTED_EDGE('',*,*,#17841,.T.) ;
#24778=ORIENTED_EDGE('',*,*,#17842,.T.) ;
#24779=ORIENTED_EDGE('',*,*,#17843,.T.) ;
#24780=ORIENTED_EDGE('',*,*,#17844,.T.) ;
#24781=ORIENTED_EDGE('',*,*,#17845,.T.) ;
#24782=ORIENTED_EDGE('',*,*,#17846,.T.) ;
#24783=ORIENTED_EDGE('',*,*,#17847,.T.) ;
#24784=ORIENTED_EDGE('',*,*,#17848,.T.) ;
#24785=ORIENTED_EDGE('',*,*,#17848,.F.) ;
#24786=ORIENTED_EDGE('',*,*,#17849,.T.) ;
#24787=ORIENTED_EDGE('',*,*,#17850,.T.) ;
#24788=ORIENTED_EDGE('',*,*,#17851,.T.) ;
#24789=ORIENTED_EDGE('',*,*,#17852,.T.) ;
#24790=ORIENTED_EDGE('',*,*,#17853,.T.) ;
#24791=ORIENTED_EDGE('',*,*,#17854,.T.) ;
#24792=ORIENTED_EDGE('',*,*,#17855,.T.) ;
#24793=ORIENTED_EDGE('',*,*,#17856,.T.) ;
#24794=ORIENTED_EDGE('',*,*,#17857,.T.) ;
#24795=ORIENTED_EDGE('',*,*,#17858,.T.) ;
#24796=ORIENTED_EDGE('',*,*,#17859,.T.) ;
#24797=ORIENTED_EDGE('',*,*,#17860,.T.) ;
#24798=ORIENTED_EDGE('',*,*,#17861,.T.) ;
#24799=ORIENTED_EDGE('',*,*,#17862,.F.) ;
#24800=ORIENTED_EDGE('',*,*,#17862,.T.) ;
#24801=ORIENTED_EDGE('',*,*,#17863,.T.) ;
#24802=ORIENTED_EDGE('',*,*,#17864,.T.) ;
#24803=ORIENTED_EDGE('',*,*,#17865,.T.) ;
#24804=ORIENTED_EDGE('',*,*,#17866,.T.) ;
#24805=ORIENTED_EDGE('',*,*,#17867,.T.) ;
#24806=ORIENTED_EDGE('',*,*,#17868,.T.) ;
#24807=ORIENTED_EDGE('',*,*,#17869,.T.) ;
#24808=ORIENTED_EDGE('',*,*,#17870,.T.) ;
#24809=ORIENTED_EDGE('',*,*,#17871,.T.) ;
#24810=ORIENTED_EDGE('',*,*,#17872,.T.) ;
#24811=ORIENTED_EDGE('',*,*,#17873,.T.) ;
#24812=ORIENTED_EDGE('',*,*,#17874,.T.) ;
#24813=ORIENTED_EDGE('',*,*,#17875,.T.) ;
#24814=ORIENTED_EDGE('',*,*,#17876,.T.) ;
#24815=ORIENTED_EDGE('',*,*,#17876,.F.) ;
#24816=ORIENTED_EDGE('',*,*,#17877,.T.) ;
#24817=ORIENTED_EDGE('',*,*,#17878,.T.) ;
#24818=ORIENTED_EDGE('',*,*,#17879,.T.) ;
#24819=ORIENTED_EDGE('',*,*,#17880,.T.) ;
#24820=ORIENTED_EDGE('',*,*,#17881,.T.) ;
#24821=ORIENTED_EDGE('',*,*,#17882,.T.) ;
#24822=ORIENTED_EDGE('',*,*,#17883,.T.) ;
#24823=ORIENTED_EDGE('',*,*,#17884,.T.) ;
#24824=ORIENTED_EDGE('',*,*,#17885,.T.) ;
#24825=ORIENTED_EDGE('',*,*,#17886,.T.) ;
#24826=ORIENTED_EDGE('',*,*,#17887,.T.) ;
#24827=ORIENTED_EDGE('',*,*,#17430,.T.) ;
#24828=ORIENTED_EDGE('',*,*,#17445,.F.) ;
#24829=ORIENTED_EDGE('',*,*,#17444,.T.) ;
#24830=ORIENTED_EDGE('',*,*,#17447,.F.) ;
#24831=ORIENTED_EDGE('',*,*,#17888,.F.) ;
#24832=ORIENTED_EDGE('',*,*,#17431,.T.) ;
#24833=ORIENTED_EDGE('',*,*,#17888,.T.) ;
#24834=ORIENTED_EDGE('',*,*,#17446,.F.) ;
#24835=ORIENTED_EDGE('',*,*,#17442,.T.) ;
#24836=ORIENTED_EDGE('',*,*,#17450,.F.) ;
#24837=ORIENTED_EDGE('',*,*,#17889,.F.) ;
#24838=ORIENTED_EDGE('',*,*,#17432,.T.) ;
#24839=ORIENTED_EDGE('',*,*,#17889,.T.) ;
#24840=ORIENTED_EDGE('',*,*,#17449,.F.) ;
#24841=ORIENTED_EDGE('',*,*,#17890,.T.) ;
#24842=ORIENTED_EDGE('',*,*,#17891,.F.) ;
#24843=ORIENTED_EDGE('',*,*,#17451,.F.) ;
#24844=ORIENTED_EDGE('',*,*,#17892,.F.) ;
#24845=ORIENTED_EDGE('',*,*,#17890,.F.) ;
#24846=ORIENTED_EDGE('',*,*,#17448,.F.) ;
#24847=ORIENTED_EDGE('',*,*,#17440,.T.) ;
#24848=ORIENTED_EDGE('',*,*,#17891,.T.) ;
#24849=ORIENTED_EDGE('',*,*,#17892,.T.) ;
#24850=ORIENTED_EDGE('',*,*,#17453,.F.) ;
#24851=ORIENTED_EDGE('',*,*,#17893,.T.) ;
#24852=ORIENTED_EDGE('',*,*,#17894,.F.) ;
#24853=ORIENTED_EDGE('',*,*,#17454,.F.) ;
#24854=ORIENTED_EDGE('',*,*,#17895,.F.) ;
#24855=ORIENTED_EDGE('',*,*,#17893,.F.) ;
#24856=ORIENTED_EDGE('',*,*,#17452,.F.) ;
#24857=ORIENTED_EDGE('',*,*,#17894,.T.) ;
#24858=ORIENTED_EDGE('',*,*,#17895,.T.) ;
#24859=ORIENTED_EDGE('',*,*,#17458,.F.) ;
#24860=ORIENTED_EDGE('',*,*,#17896,.T.) ;
#24861=ORIENTED_EDGE('',*,*,#17897,.F.) ;
#24862=ORIENTED_EDGE('',*,*,#17459,.F.) ;
#24863=ORIENTED_EDGE('',*,*,#17898,.F.) ;
#24864=ORIENTED_EDGE('',*,*,#17896,.F.) ;
#24865=ORIENTED_EDGE('',*,*,#17457,.F.) ;
#24866=ORIENTED_EDGE('',*,*,#17455,.F.) ;
#24867=ORIENTED_EDGE('',*,*,#17897,.T.) ;
#24868=ORIENTED_EDGE('',*,*,#17898,.T.) ;
#24869=ORIENTED_EDGE('',*,*,#17461,.F.) ;
#24870=ORIENTED_EDGE('',*,*,#17899,.T.) ;
#24871=ORIENTED_EDGE('',*,*,#17900,.F.) ;
#24872=ORIENTED_EDGE('',*,*,#17462,.F.) ;
#24873=ORIENTED_EDGE('',*,*,#17901,.F.) ;
#24874=ORIENTED_EDGE('',*,*,#17899,.F.) ;
#24875=ORIENTED_EDGE('',*,*,#17460,.F.) ;
#24876=ORIENTED_EDGE('',*,*,#17900,.T.) ;
#24877=ORIENTED_EDGE('',*,*,#17901,.T.) ;
#24878=ORIENTED_EDGE('',*,*,#17464,.F.) ;
#24879=ORIENTED_EDGE('',*,*,#17902,.T.) ;
#24880=ORIENTED_EDGE('',*,*,#17903,.F.) ;
#24881=ORIENTED_EDGE('',*,*,#17465,.F.) ;
#24882=ORIENTED_EDGE('',*,*,#17904,.F.) ;
#24883=ORIENTED_EDGE('',*,*,#17902,.F.) ;
#24884=ORIENTED_EDGE('',*,*,#17463,.F.) ;
#24885=ORIENTED_EDGE('',*,*,#17903,.T.) ;
#24886=ORIENTED_EDGE('',*,*,#17904,.T.) ;
#24887=ORIENTED_EDGE('',*,*,#17467,.F.) ;
#24888=ORIENTED_EDGE('',*,*,#17905,.T.) ;
#24889=ORIENTED_EDGE('',*,*,#17906,.F.) ;
#24890=ORIENTED_EDGE('',*,*,#17468,.F.) ;
#24891=ORIENTED_EDGE('',*,*,#17907,.F.) ;
#24892=ORIENTED_EDGE('',*,*,#17905,.F.) ;
#24893=ORIENTED_EDGE('',*,*,#17466,.F.) ;
#24894=ORIENTED_EDGE('',*,*,#17906,.T.) ;
#24895=ORIENTED_EDGE('',*,*,#17907,.T.) ;
#24896=ORIENTED_EDGE('',*,*,#17472,.F.) ;
#24897=ORIENTED_EDGE('',*,*,#17908,.T.) ;
#24898=ORIENTED_EDGE('',*,*,#17909,.F.) ;
#24899=ORIENTED_EDGE('',*,*,#17473,.F.) ;
#24900=ORIENTED_EDGE('',*,*,#17910,.F.) ;
#24901=ORIENTED_EDGE('',*,*,#17908,.F.) ;
#24902=ORIENTED_EDGE('',*,*,#17471,.F.) ;
#24903=ORIENTED_EDGE('',*,*,#17469,.F.) ;
#24904=ORIENTED_EDGE('',*,*,#17909,.T.) ;
#24905=ORIENTED_EDGE('',*,*,#17910,.T.) ;
#24906=ORIENTED_EDGE('',*,*,#17475,.F.) ;
#24907=ORIENTED_EDGE('',*,*,#17911,.T.) ;
#24908=ORIENTED_EDGE('',*,*,#17912,.F.) ;
#24909=ORIENTED_EDGE('',*,*,#17476,.F.) ;
#24910=ORIENTED_EDGE('',*,*,#17913,.F.) ;
#24911=ORIENTED_EDGE('',*,*,#17911,.F.) ;
#24912=ORIENTED_EDGE('',*,*,#17474,.F.) ;
#24913=ORIENTED_EDGE('',*,*,#17912,.T.) ;
#24914=ORIENTED_EDGE('',*,*,#17913,.T.) ;
#24915=ORIENTED_EDGE('',*,*,#17478,.F.) ;
#24916=ORIENTED_EDGE('',*,*,#17914,.T.) ;
#24917=ORIENTED_EDGE('',*,*,#17915,.F.) ;
#24918=ORIENTED_EDGE('',*,*,#17479,.F.) ;
#24919=ORIENTED_EDGE('',*,*,#17916,.F.) ;
#24920=ORIENTED_EDGE('',*,*,#17914,.F.) ;
#24921=ORIENTED_EDGE('',*,*,#17477,.F.) ;
#24922=ORIENTED_EDGE('',*,*,#17915,.T.) ;
#24923=ORIENTED_EDGE('',*,*,#17916,.T.) ;
#24924=ORIENTED_EDGE('',*,*,#17481,.F.) ;
#24925=ORIENTED_EDGE('',*,*,#17917,.T.) ;
#24926=ORIENTED_EDGE('',*,*,#17918,.F.) ;
#24927=ORIENTED_EDGE('',*,*,#17482,.F.) ;
#24928=ORIENTED_EDGE('',*,*,#17919,.F.) ;
#24929=ORIENTED_EDGE('',*,*,#17917,.F.) ;
#24930=ORIENTED_EDGE('',*,*,#17480,.F.) ;
#24931=ORIENTED_EDGE('',*,*,#17918,.T.) ;
#24932=ORIENTED_EDGE('',*,*,#17919,.T.) ;
#24933=ORIENTED_EDGE('',*,*,#17486,.F.) ;
#24934=ORIENTED_EDGE('',*,*,#17920,.T.) ;
#24935=ORIENTED_EDGE('',*,*,#17921,.F.) ;
#24936=ORIENTED_EDGE('',*,*,#17487,.F.) ;
#24937=ORIENTED_EDGE('',*,*,#17922,.F.) ;
#24938=ORIENTED_EDGE('',*,*,#17920,.F.) ;
#24939=ORIENTED_EDGE('',*,*,#17485,.F.) ;
#24940=ORIENTED_EDGE('',*,*,#17483,.F.) ;
#24941=ORIENTED_EDGE('',*,*,#17921,.T.) ;
#24942=ORIENTED_EDGE('',*,*,#17922,.T.) ;
#24943=ORIENTED_EDGE('',*,*,#17489,.F.) ;
#24944=ORIENTED_EDGE('',*,*,#17923,.T.) ;
#24945=ORIENTED_EDGE('',*,*,#17924,.F.) ;
#24946=ORIENTED_EDGE('',*,*,#17490,.F.) ;
#24947=ORIENTED_EDGE('',*,*,#17925,.F.) ;
#24948=ORIENTED_EDGE('',*,*,#17923,.F.) ;
#24949=ORIENTED_EDGE('',*,*,#17488,.F.) ;
#24950=ORIENTED_EDGE('',*,*,#17924,.T.) ;
#24951=ORIENTED_EDGE('',*,*,#17925,.T.) ;
#24952=ORIENTED_EDGE('',*,*,#17492,.F.) ;
#24953=ORIENTED_EDGE('',*,*,#17926,.T.) ;
#24954=ORIENTED_EDGE('',*,*,#17927,.F.) ;
#24955=ORIENTED_EDGE('',*,*,#17493,.F.) ;
#24956=ORIENTED_EDGE('',*,*,#17928,.F.) ;
#24957=ORIENTED_EDGE('',*,*,#17926,.F.) ;
#24958=ORIENTED_EDGE('',*,*,#17491,.F.) ;
#24959=ORIENTED_EDGE('',*,*,#17927,.T.) ;
#24960=ORIENTED_EDGE('',*,*,#17928,.T.) ;
#24961=ORIENTED_EDGE('',*,*,#17495,.F.) ;
#24962=ORIENTED_EDGE('',*,*,#17929,.T.) ;
#24963=ORIENTED_EDGE('',*,*,#17930,.F.) ;
#24964=ORIENTED_EDGE('',*,*,#17496,.F.) ;
#24965=ORIENTED_EDGE('',*,*,#17931,.F.) ;
#24966=ORIENTED_EDGE('',*,*,#17929,.F.) ;
#24967=ORIENTED_EDGE('',*,*,#17494,.F.) ;
#24968=ORIENTED_EDGE('',*,*,#17930,.T.) ;
#24969=ORIENTED_EDGE('',*,*,#17931,.T.) ;
#24970=ORIENTED_EDGE('',*,*,#17500,.F.) ;
#24971=ORIENTED_EDGE('',*,*,#17932,.T.) ;
#24972=ORIENTED_EDGE('',*,*,#17933,.F.) ;
#24973=ORIENTED_EDGE('',*,*,#17501,.F.) ;
#24974=ORIENTED_EDGE('',*,*,#17934,.F.) ;
#24975=ORIENTED_EDGE('',*,*,#17932,.F.) ;
#24976=ORIENTED_EDGE('',*,*,#17499,.F.) ;
#24977=ORIENTED_EDGE('',*,*,#17497,.F.) ;
#24978=ORIENTED_EDGE('',*,*,#17933,.T.) ;
#24979=ORIENTED_EDGE('',*,*,#17934,.T.) ;
#24980=ORIENTED_EDGE('',*,*,#17503,.F.) ;
#24981=ORIENTED_EDGE('',*,*,#17935,.T.) ;
#24982=ORIENTED_EDGE('',*,*,#17936,.F.) ;
#24983=ORIENTED_EDGE('',*,*,#17504,.F.) ;
#24984=ORIENTED_EDGE('',*,*,#17937,.F.) ;
#24985=ORIENTED_EDGE('',*,*,#17935,.F.) ;
#24986=ORIENTED_EDGE('',*,*,#17502,.F.) ;
#24987=ORIENTED_EDGE('',*,*,#17936,.T.) ;
#24988=ORIENTED_EDGE('',*,*,#17937,.T.) ;
#24989=ORIENTED_EDGE('',*,*,#17506,.F.) ;
#24990=ORIENTED_EDGE('',*,*,#17938,.T.) ;
#24991=ORIENTED_EDGE('',*,*,#17939,.F.) ;
#24992=ORIENTED_EDGE('',*,*,#17507,.F.) ;
#24993=ORIENTED_EDGE('',*,*,#17940,.F.) ;
#24994=ORIENTED_EDGE('',*,*,#17938,.F.) ;
#24995=ORIENTED_EDGE('',*,*,#17505,.F.) ;
#24996=ORIENTED_EDGE('',*,*,#17939,.T.) ;
#24997=ORIENTED_EDGE('',*,*,#17940,.T.) ;
#24998=ORIENTED_EDGE('',*,*,#17509,.F.) ;
#24999=ORIENTED_EDGE('',*,*,#17941,.T.) ;
#25000=ORIENTED_EDGE('',*,*,#17942,.F.) ;
#25001=ORIENTED_EDGE('',*,*,#17510,.F.) ;
#25002=ORIENTED_EDGE('',*,*,#17943,.F.) ;
#25003=ORIENTED_EDGE('',*,*,#17941,.F.) ;
#25004=ORIENTED_EDGE('',*,*,#17508,.F.) ;
#25005=ORIENTED_EDGE('',*,*,#17942,.T.) ;
#25006=ORIENTED_EDGE('',*,*,#17943,.T.) ;
#25007=ORIENTED_EDGE('',*,*,#17514,.F.) ;
#25008=ORIENTED_EDGE('',*,*,#17944,.T.) ;
#25009=ORIENTED_EDGE('',*,*,#17945,.F.) ;
#25010=ORIENTED_EDGE('',*,*,#17515,.F.) ;
#25011=ORIENTED_EDGE('',*,*,#17946,.F.) ;
#25012=ORIENTED_EDGE('',*,*,#17944,.F.) ;
#25013=ORIENTED_EDGE('',*,*,#17513,.F.) ;
#25014=ORIENTED_EDGE('',*,*,#17511,.F.) ;
#25015=ORIENTED_EDGE('',*,*,#17945,.T.) ;
#25016=ORIENTED_EDGE('',*,*,#17946,.T.) ;
#25017=ORIENTED_EDGE('',*,*,#17517,.F.) ;
#25018=ORIENTED_EDGE('',*,*,#17947,.T.) ;
#25019=ORIENTED_EDGE('',*,*,#17948,.F.) ;
#25020=ORIENTED_EDGE('',*,*,#17518,.F.) ;
#25021=ORIENTED_EDGE('',*,*,#17949,.F.) ;
#25022=ORIENTED_EDGE('',*,*,#17947,.F.) ;
#25023=ORIENTED_EDGE('',*,*,#17516,.F.) ;
#25024=ORIENTED_EDGE('',*,*,#17948,.T.) ;
#25025=ORIENTED_EDGE('',*,*,#17949,.T.) ;
#25026=ORIENTED_EDGE('',*,*,#17520,.F.) ;
#25027=ORIENTED_EDGE('',*,*,#17950,.T.) ;
#25028=ORIENTED_EDGE('',*,*,#17951,.F.) ;
#25029=ORIENTED_EDGE('',*,*,#17521,.F.) ;
#25030=ORIENTED_EDGE('',*,*,#17952,.F.) ;
#25031=ORIENTED_EDGE('',*,*,#17950,.F.) ;
#25032=ORIENTED_EDGE('',*,*,#17519,.F.) ;
#25033=ORIENTED_EDGE('',*,*,#17951,.T.) ;
#25034=ORIENTED_EDGE('',*,*,#17952,.T.) ;
#25035=ORIENTED_EDGE('',*,*,#17523,.F.) ;
#25036=ORIENTED_EDGE('',*,*,#17953,.T.) ;
#25037=ORIENTED_EDGE('',*,*,#17954,.F.) ;
#25038=ORIENTED_EDGE('',*,*,#17524,.F.) ;
#25039=ORIENTED_EDGE('',*,*,#17955,.F.) ;
#25040=ORIENTED_EDGE('',*,*,#17953,.F.) ;
#25041=ORIENTED_EDGE('',*,*,#17522,.F.) ;
#25042=ORIENTED_EDGE('',*,*,#17954,.T.) ;
#25043=ORIENTED_EDGE('',*,*,#17955,.T.) ;
#25044=ORIENTED_EDGE('',*,*,#17528,.F.) ;
#25045=ORIENTED_EDGE('',*,*,#17956,.T.) ;
#25046=ORIENTED_EDGE('',*,*,#17957,.F.) ;
#25047=ORIENTED_EDGE('',*,*,#17529,.F.) ;
#25048=ORIENTED_EDGE('',*,*,#17958,.F.) ;
#25049=ORIENTED_EDGE('',*,*,#17956,.F.) ;
#25050=ORIENTED_EDGE('',*,*,#17527,.F.) ;
#25051=ORIENTED_EDGE('',*,*,#17525,.F.) ;
#25052=ORIENTED_EDGE('',*,*,#17957,.T.) ;
#25053=ORIENTED_EDGE('',*,*,#17958,.T.) ;
#25054=ORIENTED_EDGE('',*,*,#17531,.F.) ;
#25055=ORIENTED_EDGE('',*,*,#17959,.T.) ;
#25056=ORIENTED_EDGE('',*,*,#17960,.F.) ;
#25057=ORIENTED_EDGE('',*,*,#17532,.F.) ;
#25058=ORIENTED_EDGE('',*,*,#17961,.F.) ;
#25059=ORIENTED_EDGE('',*,*,#17959,.F.) ;
#25060=ORIENTED_EDGE('',*,*,#17530,.F.) ;
#25061=ORIENTED_EDGE('',*,*,#17960,.T.) ;
#25062=ORIENTED_EDGE('',*,*,#17961,.T.) ;
#25063=ORIENTED_EDGE('',*,*,#17534,.F.) ;
#25064=ORIENTED_EDGE('',*,*,#17962,.T.) ;
#25065=ORIENTED_EDGE('',*,*,#17963,.F.) ;
#25066=ORIENTED_EDGE('',*,*,#17535,.F.) ;
#25067=ORIENTED_EDGE('',*,*,#17964,.F.) ;
#25068=ORIENTED_EDGE('',*,*,#17962,.F.) ;
#25069=ORIENTED_EDGE('',*,*,#17533,.F.) ;
#25070=ORIENTED_EDGE('',*,*,#17963,.T.) ;
#25071=ORIENTED_EDGE('',*,*,#17964,.T.) ;
#25072=ORIENTED_EDGE('',*,*,#17537,.F.) ;
#25073=ORIENTED_EDGE('',*,*,#17965,.T.) ;
#25074=ORIENTED_EDGE('',*,*,#17966,.F.) ;
#25075=ORIENTED_EDGE('',*,*,#17538,.F.) ;
#25076=ORIENTED_EDGE('',*,*,#17967,.F.) ;
#25077=ORIENTED_EDGE('',*,*,#17965,.F.) ;
#25078=ORIENTED_EDGE('',*,*,#17536,.F.) ;
#25079=ORIENTED_EDGE('',*,*,#17966,.T.) ;
#25080=ORIENTED_EDGE('',*,*,#17967,.T.) ;
#25081=ORIENTED_EDGE('',*,*,#17542,.F.) ;
#25082=ORIENTED_EDGE('',*,*,#17968,.T.) ;
#25083=ORIENTED_EDGE('',*,*,#17969,.F.) ;
#25084=ORIENTED_EDGE('',*,*,#17543,.F.) ;
#25085=ORIENTED_EDGE('',*,*,#17970,.F.) ;
#25086=ORIENTED_EDGE('',*,*,#17968,.F.) ;
#25087=ORIENTED_EDGE('',*,*,#17541,.F.) ;
#25088=ORIENTED_EDGE('',*,*,#17539,.F.) ;
#25089=ORIENTED_EDGE('',*,*,#17969,.T.) ;
#25090=ORIENTED_EDGE('',*,*,#17970,.T.) ;
#25091=ORIENTED_EDGE('',*,*,#17545,.F.) ;
#25092=ORIENTED_EDGE('',*,*,#17971,.T.) ;
#25093=ORIENTED_EDGE('',*,*,#17972,.F.) ;
#25094=ORIENTED_EDGE('',*,*,#17546,.F.) ;
#25095=ORIENTED_EDGE('',*,*,#17973,.F.) ;
#25096=ORIENTED_EDGE('',*,*,#17971,.F.) ;
#25097=ORIENTED_EDGE('',*,*,#17544,.F.) ;
#25098=ORIENTED_EDGE('',*,*,#17972,.T.) ;
#25099=ORIENTED_EDGE('',*,*,#17973,.T.) ;
#25100=ORIENTED_EDGE('',*,*,#17548,.F.) ;
#25101=ORIENTED_EDGE('',*,*,#17974,.T.) ;
#25102=ORIENTED_EDGE('',*,*,#17975,.F.) ;
#25103=ORIENTED_EDGE('',*,*,#17549,.F.) ;
#25104=ORIENTED_EDGE('',*,*,#17976,.F.) ;
#25105=ORIENTED_EDGE('',*,*,#17974,.F.) ;
#25106=ORIENTED_EDGE('',*,*,#17547,.F.) ;
#25107=ORIENTED_EDGE('',*,*,#17975,.T.) ;
#25108=ORIENTED_EDGE('',*,*,#17976,.T.) ;
#25109=ORIENTED_EDGE('',*,*,#17551,.F.) ;
#25110=ORIENTED_EDGE('',*,*,#17977,.T.) ;
#25111=ORIENTED_EDGE('',*,*,#17978,.F.) ;
#25112=ORIENTED_EDGE('',*,*,#17552,.F.) ;
#25113=ORIENTED_EDGE('',*,*,#17979,.F.) ;
#25114=ORIENTED_EDGE('',*,*,#17977,.F.) ;
#25115=ORIENTED_EDGE('',*,*,#17550,.F.) ;
#25116=ORIENTED_EDGE('',*,*,#17978,.T.) ;
#25117=ORIENTED_EDGE('',*,*,#17979,.T.) ;
#25118=ORIENTED_EDGE('',*,*,#17556,.F.) ;
#25119=ORIENTED_EDGE('',*,*,#17980,.T.) ;
#25120=ORIENTED_EDGE('',*,*,#17981,.F.) ;
#25121=ORIENTED_EDGE('',*,*,#17557,.F.) ;
#25122=ORIENTED_EDGE('',*,*,#17982,.F.) ;
#25123=ORIENTED_EDGE('',*,*,#17980,.F.) ;
#25124=ORIENTED_EDGE('',*,*,#17555,.F.) ;
#25125=ORIENTED_EDGE('',*,*,#17553,.F.) ;
#25126=ORIENTED_EDGE('',*,*,#17981,.T.) ;
#25127=ORIENTED_EDGE('',*,*,#17982,.T.) ;
#25128=ORIENTED_EDGE('',*,*,#17559,.F.) ;
#25129=ORIENTED_EDGE('',*,*,#17983,.T.) ;
#25130=ORIENTED_EDGE('',*,*,#17984,.F.) ;
#25131=ORIENTED_EDGE('',*,*,#17560,.F.) ;
#25132=ORIENTED_EDGE('',*,*,#17985,.F.) ;
#25133=ORIENTED_EDGE('',*,*,#17983,.F.) ;
#25134=ORIENTED_EDGE('',*,*,#17558,.F.) ;
#25135=ORIENTED_EDGE('',*,*,#17984,.T.) ;
#25136=ORIENTED_EDGE('',*,*,#17985,.T.) ;
#25137=ORIENTED_EDGE('',*,*,#17562,.F.) ;
#25138=ORIENTED_EDGE('',*,*,#17986,.T.) ;
#25139=ORIENTED_EDGE('',*,*,#17987,.F.) ;
#25140=ORIENTED_EDGE('',*,*,#17563,.F.) ;
#25141=ORIENTED_EDGE('',*,*,#17988,.F.) ;
#25142=ORIENTED_EDGE('',*,*,#17986,.F.) ;
#25143=ORIENTED_EDGE('',*,*,#17561,.F.) ;
#25144=ORIENTED_EDGE('',*,*,#17987,.T.) ;
#25145=ORIENTED_EDGE('',*,*,#17988,.T.) ;
#25146=ORIENTED_EDGE('',*,*,#17565,.F.) ;
#25147=ORIENTED_EDGE('',*,*,#17989,.T.) ;
#25148=ORIENTED_EDGE('',*,*,#17990,.F.) ;
#25149=ORIENTED_EDGE('',*,*,#17566,.F.) ;
#25150=ORIENTED_EDGE('',*,*,#17991,.F.) ;
#25151=ORIENTED_EDGE('',*,*,#17989,.F.) ;
#25152=ORIENTED_EDGE('',*,*,#17564,.F.) ;
#25153=ORIENTED_EDGE('',*,*,#17990,.T.) ;
#25154=ORIENTED_EDGE('',*,*,#17991,.T.) ;
#25155=ORIENTED_EDGE('',*,*,#17570,.F.) ;
#25156=ORIENTED_EDGE('',*,*,#17992,.T.) ;
#25157=ORIENTED_EDGE('',*,*,#17993,.F.) ;
#25158=ORIENTED_EDGE('',*,*,#17571,.F.) ;
#25159=ORIENTED_EDGE('',*,*,#17994,.F.) ;
#25160=ORIENTED_EDGE('',*,*,#17992,.F.) ;
#25161=ORIENTED_EDGE('',*,*,#17569,.F.) ;
#25162=ORIENTED_EDGE('',*,*,#17567,.F.) ;
#25163=ORIENTED_EDGE('',*,*,#17993,.T.) ;
#25164=ORIENTED_EDGE('',*,*,#17994,.T.) ;
#25165=ORIENTED_EDGE('',*,*,#17573,.F.) ;
#25166=ORIENTED_EDGE('',*,*,#17995,.T.) ;
#25167=ORIENTED_EDGE('',*,*,#17996,.F.) ;
#25168=ORIENTED_EDGE('',*,*,#17574,.F.) ;
#25169=ORIENTED_EDGE('',*,*,#17997,.F.) ;
#25170=ORIENTED_EDGE('',*,*,#17995,.F.) ;
#25171=ORIENTED_EDGE('',*,*,#17572,.F.) ;
#25172=ORIENTED_EDGE('',*,*,#17996,.T.) ;
#25173=ORIENTED_EDGE('',*,*,#17997,.T.) ;
#25174=ORIENTED_EDGE('',*,*,#17576,.F.) ;
#25175=ORIENTED_EDGE('',*,*,#17998,.T.) ;
#25176=ORIENTED_EDGE('',*,*,#17999,.F.) ;
#25177=ORIENTED_EDGE('',*,*,#17577,.F.) ;
#25178=ORIENTED_EDGE('',*,*,#18000,.F.) ;
#25179=ORIENTED_EDGE('',*,*,#17998,.F.) ;
#25180=ORIENTED_EDGE('',*,*,#17575,.F.) ;
#25181=ORIENTED_EDGE('',*,*,#17999,.T.) ;
#25182=ORIENTED_EDGE('',*,*,#18000,.T.) ;
#25183=ORIENTED_EDGE('',*,*,#17579,.F.) ;
#25184=ORIENTED_EDGE('',*,*,#18001,.T.) ;
#25185=ORIENTED_EDGE('',*,*,#18002,.F.) ;
#25186=ORIENTED_EDGE('',*,*,#17580,.F.) ;
#25187=ORIENTED_EDGE('',*,*,#18003,.F.) ;
#25188=ORIENTED_EDGE('',*,*,#18001,.F.) ;
#25189=ORIENTED_EDGE('',*,*,#17578,.F.) ;
#25190=ORIENTED_EDGE('',*,*,#18002,.T.) ;
#25191=ORIENTED_EDGE('',*,*,#18003,.T.) ;
#25192=ORIENTED_EDGE('',*,*,#17584,.F.) ;
#25193=ORIENTED_EDGE('',*,*,#18004,.T.) ;
#25194=ORIENTED_EDGE('',*,*,#18005,.F.) ;
#25195=ORIENTED_EDGE('',*,*,#17585,.F.) ;
#25196=ORIENTED_EDGE('',*,*,#18006,.F.) ;
#25197=ORIENTED_EDGE('',*,*,#18004,.F.) ;
#25198=ORIENTED_EDGE('',*,*,#17583,.F.) ;
#25199=ORIENTED_EDGE('',*,*,#17581,.F.) ;
#25200=ORIENTED_EDGE('',*,*,#18005,.T.) ;
#25201=ORIENTED_EDGE('',*,*,#18006,.T.) ;
#25202=ORIENTED_EDGE('',*,*,#17587,.F.) ;
#25203=ORIENTED_EDGE('',*,*,#18007,.T.) ;
#25204=ORIENTED_EDGE('',*,*,#18008,.F.) ;
#25205=ORIENTED_EDGE('',*,*,#17588,.F.) ;
#25206=ORIENTED_EDGE('',*,*,#18009,.F.) ;
#25207=ORIENTED_EDGE('',*,*,#18007,.F.) ;
#25208=ORIENTED_EDGE('',*,*,#17586,.F.) ;
#25209=ORIENTED_EDGE('',*,*,#18008,.T.) ;
#25210=ORIENTED_EDGE('',*,*,#18009,.T.) ;
#25211=ORIENTED_EDGE('',*,*,#17590,.F.) ;
#25212=ORIENTED_EDGE('',*,*,#18010,.T.) ;
#25213=ORIENTED_EDGE('',*,*,#18011,.F.) ;
#25214=ORIENTED_EDGE('',*,*,#17591,.F.) ;
#25215=ORIENTED_EDGE('',*,*,#18012,.F.) ;
#25216=ORIENTED_EDGE('',*,*,#18010,.F.) ;
#25217=ORIENTED_EDGE('',*,*,#17589,.F.) ;
#25218=ORIENTED_EDGE('',*,*,#18011,.T.) ;
#25219=ORIENTED_EDGE('',*,*,#18012,.T.) ;
#25220=ORIENTED_EDGE('',*,*,#17593,.F.) ;
#25221=ORIENTED_EDGE('',*,*,#18013,.T.) ;
#25222=ORIENTED_EDGE('',*,*,#18014,.F.) ;
#25223=ORIENTED_EDGE('',*,*,#17594,.F.) ;
#25224=ORIENTED_EDGE('',*,*,#18015,.F.) ;
#25225=ORIENTED_EDGE('',*,*,#18013,.F.) ;
#25226=ORIENTED_EDGE('',*,*,#17592,.F.) ;
#25227=ORIENTED_EDGE('',*,*,#18014,.T.) ;
#25228=ORIENTED_EDGE('',*,*,#18015,.T.) ;
#25229=ORIENTED_EDGE('',*,*,#17598,.F.) ;
#25230=ORIENTED_EDGE('',*,*,#18016,.T.) ;
#25231=ORIENTED_EDGE('',*,*,#18017,.F.) ;
#25232=ORIENTED_EDGE('',*,*,#17599,.F.) ;
#25233=ORIENTED_EDGE('',*,*,#18018,.F.) ;
#25234=ORIENTED_EDGE('',*,*,#18016,.F.) ;
#25235=ORIENTED_EDGE('',*,*,#17597,.F.) ;
#25236=ORIENTED_EDGE('',*,*,#17595,.F.) ;
#25237=ORIENTED_EDGE('',*,*,#18017,.T.) ;
#25238=ORIENTED_EDGE('',*,*,#18018,.T.) ;
#25239=ORIENTED_EDGE('',*,*,#17601,.F.) ;
#25240=ORIENTED_EDGE('',*,*,#18019,.T.) ;
#25241=ORIENTED_EDGE('',*,*,#18020,.F.) ;
#25242=ORIENTED_EDGE('',*,*,#17602,.F.) ;
#25243=ORIENTED_EDGE('',*,*,#18021,.F.) ;
#25244=ORIENTED_EDGE('',*,*,#18019,.F.) ;
#25245=ORIENTED_EDGE('',*,*,#17600,.F.) ;
#25246=ORIENTED_EDGE('',*,*,#18020,.T.) ;
#25247=ORIENTED_EDGE('',*,*,#18021,.T.) ;
#25248=ORIENTED_EDGE('',*,*,#17604,.F.) ;
#25249=ORIENTED_EDGE('',*,*,#18022,.T.) ;
#25250=ORIENTED_EDGE('',*,*,#18023,.F.) ;
#25251=ORIENTED_EDGE('',*,*,#17605,.F.) ;
#25252=ORIENTED_EDGE('',*,*,#18024,.F.) ;
#25253=ORIENTED_EDGE('',*,*,#18022,.F.) ;
#25254=ORIENTED_EDGE('',*,*,#17603,.F.) ;
#25255=ORIENTED_EDGE('',*,*,#18023,.T.) ;
#25256=ORIENTED_EDGE('',*,*,#18024,.T.) ;
#25257=ORIENTED_EDGE('',*,*,#17607,.F.) ;
#25258=ORIENTED_EDGE('',*,*,#18025,.T.) ;
#25259=ORIENTED_EDGE('',*,*,#18026,.F.) ;
#25260=ORIENTED_EDGE('',*,*,#17608,.F.) ;
#25261=ORIENTED_EDGE('',*,*,#18027,.F.) ;
#25262=ORIENTED_EDGE('',*,*,#18025,.F.) ;
#25263=ORIENTED_EDGE('',*,*,#17606,.F.) ;
#25264=ORIENTED_EDGE('',*,*,#18026,.T.) ;
#25265=ORIENTED_EDGE('',*,*,#18027,.T.) ;
#25266=ORIENTED_EDGE('',*,*,#17612,.F.) ;
#25267=ORIENTED_EDGE('',*,*,#18028,.T.) ;
#25268=ORIENTED_EDGE('',*,*,#18029,.F.) ;
#25269=ORIENTED_EDGE('',*,*,#17613,.F.) ;
#25270=ORIENTED_EDGE('',*,*,#18030,.F.) ;
#25271=ORIENTED_EDGE('',*,*,#18028,.F.) ;
#25272=ORIENTED_EDGE('',*,*,#17611,.F.) ;
#25273=ORIENTED_EDGE('',*,*,#17609,.F.) ;
#25274=ORIENTED_EDGE('',*,*,#18029,.T.) ;
#25275=ORIENTED_EDGE('',*,*,#18030,.T.) ;
#25276=ORIENTED_EDGE('',*,*,#17615,.F.) ;
#25277=ORIENTED_EDGE('',*,*,#18031,.T.) ;
#25278=ORIENTED_EDGE('',*,*,#18032,.F.) ;
#25279=ORIENTED_EDGE('',*,*,#17616,.F.) ;
#25280=ORIENTED_EDGE('',*,*,#18033,.F.) ;
#25281=ORIENTED_EDGE('',*,*,#18031,.F.) ;
#25282=ORIENTED_EDGE('',*,*,#17614,.F.) ;
#25283=ORIENTED_EDGE('',*,*,#18032,.T.) ;
#25284=ORIENTED_EDGE('',*,*,#18033,.T.) ;
#25285=ORIENTED_EDGE('',*,*,#17618,.F.) ;
#25286=ORIENTED_EDGE('',*,*,#18034,.T.) ;
#25287=ORIENTED_EDGE('',*,*,#18035,.F.) ;
#25288=ORIENTED_EDGE('',*,*,#17619,.F.) ;
#25289=ORIENTED_EDGE('',*,*,#18036,.F.) ;
#25290=ORIENTED_EDGE('',*,*,#18034,.F.) ;
#25291=ORIENTED_EDGE('',*,*,#17617,.F.) ;
#25292=ORIENTED_EDGE('',*,*,#18035,.T.) ;
#25293=ORIENTED_EDGE('',*,*,#18036,.T.) ;
#25294=ORIENTED_EDGE('',*,*,#17621,.F.) ;
#25295=ORIENTED_EDGE('',*,*,#18037,.T.) ;
#25296=ORIENTED_EDGE('',*,*,#18038,.F.) ;
#25297=ORIENTED_EDGE('',*,*,#17622,.F.) ;
#25298=ORIENTED_EDGE('',*,*,#18039,.F.) ;
#25299=ORIENTED_EDGE('',*,*,#18037,.F.) ;
#25300=ORIENTED_EDGE('',*,*,#17620,.F.) ;
#25301=ORIENTED_EDGE('',*,*,#18038,.T.) ;
#25302=ORIENTED_EDGE('',*,*,#18039,.T.) ;
#25303=ORIENTED_EDGE('',*,*,#17626,.F.) ;
#25304=ORIENTED_EDGE('',*,*,#18040,.T.) ;
#25305=ORIENTED_EDGE('',*,*,#18041,.F.) ;
#25306=ORIENTED_EDGE('',*,*,#17627,.F.) ;
#25307=ORIENTED_EDGE('',*,*,#18042,.F.) ;
#25308=ORIENTED_EDGE('',*,*,#18040,.F.) ;
#25309=ORIENTED_EDGE('',*,*,#17625,.F.) ;
#25310=ORIENTED_EDGE('',*,*,#17623,.F.) ;
#25311=ORIENTED_EDGE('',*,*,#18041,.T.) ;
#25312=ORIENTED_EDGE('',*,*,#18042,.T.) ;
#25313=ORIENTED_EDGE('',*,*,#17629,.F.) ;
#25314=ORIENTED_EDGE('',*,*,#18043,.T.) ;
#25315=ORIENTED_EDGE('',*,*,#18044,.F.) ;
#25316=ORIENTED_EDGE('',*,*,#17630,.F.) ;
#25317=ORIENTED_EDGE('',*,*,#18045,.F.) ;
#25318=ORIENTED_EDGE('',*,*,#18043,.F.) ;
#25319=ORIENTED_EDGE('',*,*,#17628,.F.) ;
#25320=ORIENTED_EDGE('',*,*,#18044,.T.) ;
#25321=ORIENTED_EDGE('',*,*,#18045,.T.) ;
#25322=ORIENTED_EDGE('',*,*,#17632,.F.) ;
#25323=ORIENTED_EDGE('',*,*,#18046,.T.) ;
#25324=ORIENTED_EDGE('',*,*,#18047,.F.) ;
#25325=ORIENTED_EDGE('',*,*,#17633,.F.) ;
#25326=ORIENTED_EDGE('',*,*,#18048,.F.) ;
#25327=ORIENTED_EDGE('',*,*,#18046,.F.) ;
#25328=ORIENTED_EDGE('',*,*,#17631,.F.) ;
#25329=ORIENTED_EDGE('',*,*,#18047,.T.) ;
#25330=ORIENTED_EDGE('',*,*,#18048,.T.) ;
#25331=ORIENTED_EDGE('',*,*,#17635,.F.) ;
#25332=ORIENTED_EDGE('',*,*,#18049,.T.) ;
#25333=ORIENTED_EDGE('',*,*,#18050,.F.) ;
#25334=ORIENTED_EDGE('',*,*,#17636,.F.) ;
#25335=ORIENTED_EDGE('',*,*,#18051,.F.) ;
#25336=ORIENTED_EDGE('',*,*,#18049,.F.) ;
#25337=ORIENTED_EDGE('',*,*,#17634,.F.) ;
#25338=ORIENTED_EDGE('',*,*,#18050,.T.) ;
#25339=ORIENTED_EDGE('',*,*,#18051,.T.) ;
#25340=ORIENTED_EDGE('',*,*,#17640,.F.) ;
#25341=ORIENTED_EDGE('',*,*,#18052,.T.) ;
#25342=ORIENTED_EDGE('',*,*,#18053,.F.) ;
#25343=ORIENTED_EDGE('',*,*,#17641,.F.) ;
#25344=ORIENTED_EDGE('',*,*,#18054,.F.) ;
#25345=ORIENTED_EDGE('',*,*,#18052,.F.) ;
#25346=ORIENTED_EDGE('',*,*,#17639,.F.) ;
#25347=ORIENTED_EDGE('',*,*,#17637,.F.) ;
#25348=ORIENTED_EDGE('',*,*,#18053,.T.) ;
#25349=ORIENTED_EDGE('',*,*,#18054,.T.) ;
#25350=ORIENTED_EDGE('',*,*,#17643,.F.) ;
#25351=ORIENTED_EDGE('',*,*,#18055,.T.) ;
#25352=ORIENTED_EDGE('',*,*,#18056,.F.) ;
#25353=ORIENTED_EDGE('',*,*,#17644,.F.) ;
#25354=ORIENTED_EDGE('',*,*,#18057,.F.) ;
#25355=ORIENTED_EDGE('',*,*,#18055,.F.) ;
#25356=ORIENTED_EDGE('',*,*,#17642,.F.) ;
#25357=ORIENTED_EDGE('',*,*,#18056,.T.) ;
#25358=ORIENTED_EDGE('',*,*,#18057,.T.) ;
#25359=ORIENTED_EDGE('',*,*,#17646,.F.) ;
#25360=ORIENTED_EDGE('',*,*,#18058,.T.) ;
#25361=ORIENTED_EDGE('',*,*,#18059,.F.) ;
#25362=ORIENTED_EDGE('',*,*,#17647,.F.) ;
#25363=ORIENTED_EDGE('',*,*,#18060,.F.) ;
#25364=ORIENTED_EDGE('',*,*,#18058,.F.) ;
#25365=ORIENTED_EDGE('',*,*,#17645,.F.) ;
#25366=ORIENTED_EDGE('',*,*,#18059,.T.) ;
#25367=ORIENTED_EDGE('',*,*,#18060,.T.) ;
#25368=ORIENTED_EDGE('',*,*,#17649,.F.) ;
#25369=ORIENTED_EDGE('',*,*,#18061,.T.) ;
#25370=ORIENTED_EDGE('',*,*,#18062,.F.) ;
#25371=ORIENTED_EDGE('',*,*,#17650,.F.) ;
#25372=ORIENTED_EDGE('',*,*,#18063,.F.) ;
#25373=ORIENTED_EDGE('',*,*,#18061,.F.) ;
#25374=ORIENTED_EDGE('',*,*,#17648,.F.) ;
#25375=ORIENTED_EDGE('',*,*,#18062,.T.) ;
#25376=ORIENTED_EDGE('',*,*,#18063,.T.) ;
#25377=ORIENTED_EDGE('',*,*,#17654,.F.) ;
#25378=ORIENTED_EDGE('',*,*,#18064,.T.) ;
#25379=ORIENTED_EDGE('',*,*,#18065,.F.) ;
#25380=ORIENTED_EDGE('',*,*,#17655,.F.) ;
#25381=ORIENTED_EDGE('',*,*,#18066,.F.) ;
#25382=ORIENTED_EDGE('',*,*,#18064,.F.) ;
#25383=ORIENTED_EDGE('',*,*,#17653,.F.) ;
#25384=ORIENTED_EDGE('',*,*,#17651,.F.) ;
#25385=ORIENTED_EDGE('',*,*,#18065,.T.) ;
#25386=ORIENTED_EDGE('',*,*,#18066,.T.) ;
#25387=ORIENTED_EDGE('',*,*,#17657,.F.) ;
#25388=ORIENTED_EDGE('',*,*,#18067,.T.) ;
#25389=ORIENTED_EDGE('',*,*,#18068,.F.) ;
#25390=ORIENTED_EDGE('',*,*,#17658,.F.) ;
#25391=ORIENTED_EDGE('',*,*,#18069,.F.) ;
#25392=ORIENTED_EDGE('',*,*,#18067,.F.) ;
#25393=ORIENTED_EDGE('',*,*,#17656,.F.) ;
#25394=ORIENTED_EDGE('',*,*,#18068,.T.) ;
#25395=ORIENTED_EDGE('',*,*,#18069,.T.) ;
#25396=ORIENTED_EDGE('',*,*,#17660,.F.) ;
#25397=ORIENTED_EDGE('',*,*,#18070,.T.) ;
#25398=ORIENTED_EDGE('',*,*,#18071,.F.) ;
#25399=ORIENTED_EDGE('',*,*,#17661,.F.) ;
#25400=ORIENTED_EDGE('',*,*,#18072,.F.) ;
#25401=ORIENTED_EDGE('',*,*,#18070,.F.) ;
#25402=ORIENTED_EDGE('',*,*,#17659,.F.) ;
#25403=ORIENTED_EDGE('',*,*,#18071,.T.) ;
#25404=ORIENTED_EDGE('',*,*,#18072,.T.) ;
#25405=ORIENTED_EDGE('',*,*,#17663,.F.) ;
#25406=ORIENTED_EDGE('',*,*,#18073,.T.) ;
#25407=ORIENTED_EDGE('',*,*,#18074,.F.) ;
#25408=ORIENTED_EDGE('',*,*,#17664,.F.) ;
#25409=ORIENTED_EDGE('',*,*,#18075,.F.) ;
#25410=ORIENTED_EDGE('',*,*,#18073,.F.) ;
#25411=ORIENTED_EDGE('',*,*,#17662,.F.) ;
#25412=ORIENTED_EDGE('',*,*,#18074,.T.) ;
#25413=ORIENTED_EDGE('',*,*,#18075,.T.) ;
#25414=ORIENTED_EDGE('',*,*,#17668,.F.) ;
#25415=ORIENTED_EDGE('',*,*,#18076,.T.) ;
#25416=ORIENTED_EDGE('',*,*,#18077,.F.) ;
#25417=ORIENTED_EDGE('',*,*,#17669,.F.) ;
#25418=ORIENTED_EDGE('',*,*,#18078,.F.) ;
#25419=ORIENTED_EDGE('',*,*,#18076,.F.) ;
#25420=ORIENTED_EDGE('',*,*,#17667,.F.) ;
#25421=ORIENTED_EDGE('',*,*,#17665,.F.) ;
#25422=ORIENTED_EDGE('',*,*,#18077,.T.) ;
#25423=ORIENTED_EDGE('',*,*,#18078,.T.) ;
#25424=ORIENTED_EDGE('',*,*,#17671,.F.) ;
#25425=ORIENTED_EDGE('',*,*,#18079,.T.) ;
#25426=ORIENTED_EDGE('',*,*,#18080,.F.) ;
#25427=ORIENTED_EDGE('',*,*,#17672,.F.) ;
#25428=ORIENTED_EDGE('',*,*,#18081,.F.) ;
#25429=ORIENTED_EDGE('',*,*,#18079,.F.) ;
#25430=ORIENTED_EDGE('',*,*,#17670,.F.) ;
#25431=ORIENTED_EDGE('',*,*,#18080,.T.) ;
#25432=ORIENTED_EDGE('',*,*,#18081,.T.) ;
#25433=ORIENTED_EDGE('',*,*,#17674,.F.) ;
#25434=ORIENTED_EDGE('',*,*,#18082,.T.) ;
#25435=ORIENTED_EDGE('',*,*,#18083,.F.) ;
#25436=ORIENTED_EDGE('',*,*,#17675,.F.) ;
#25437=ORIENTED_EDGE('',*,*,#18084,.F.) ;
#25438=ORIENTED_EDGE('',*,*,#18082,.F.) ;
#25439=ORIENTED_EDGE('',*,*,#17673,.F.) ;
#25440=ORIENTED_EDGE('',*,*,#18083,.T.) ;
#25441=ORIENTED_EDGE('',*,*,#18084,.T.) ;
#25442=ORIENTED_EDGE('',*,*,#17677,.F.) ;
#25443=ORIENTED_EDGE('',*,*,#18085,.T.) ;
#25444=ORIENTED_EDGE('',*,*,#18086,.F.) ;
#25445=ORIENTED_EDGE('',*,*,#17678,.F.) ;
#25446=ORIENTED_EDGE('',*,*,#18087,.F.) ;
#25447=ORIENTED_EDGE('',*,*,#18085,.F.) ;
#25448=ORIENTED_EDGE('',*,*,#17676,.F.) ;
#25449=ORIENTED_EDGE('',*,*,#18086,.T.) ;
#25450=ORIENTED_EDGE('',*,*,#18087,.T.) ;
#25451=ORIENTED_EDGE('',*,*,#17682,.F.) ;
#25452=ORIENTED_EDGE('',*,*,#18088,.T.) ;
#25453=ORIENTED_EDGE('',*,*,#18089,.F.) ;
#25454=ORIENTED_EDGE('',*,*,#17683,.F.) ;
#25455=ORIENTED_EDGE('',*,*,#18090,.F.) ;
#25456=ORIENTED_EDGE('',*,*,#18088,.F.) ;
#25457=ORIENTED_EDGE('',*,*,#17681,.F.) ;
#25458=ORIENTED_EDGE('',*,*,#17679,.F.) ;
#25459=ORIENTED_EDGE('',*,*,#18089,.T.) ;
#25460=ORIENTED_EDGE('',*,*,#18090,.T.) ;
#25461=ORIENTED_EDGE('',*,*,#17685,.F.) ;
#25462=ORIENTED_EDGE('',*,*,#18091,.T.) ;
#25463=ORIENTED_EDGE('',*,*,#18092,.F.) ;
#25464=ORIENTED_EDGE('',*,*,#17686,.F.) ;
#25465=ORIENTED_EDGE('',*,*,#18093,.F.) ;
#25466=ORIENTED_EDGE('',*,*,#18091,.F.) ;
#25467=ORIENTED_EDGE('',*,*,#17684,.F.) ;
#25468=ORIENTED_EDGE('',*,*,#18092,.T.) ;
#25469=ORIENTED_EDGE('',*,*,#18093,.T.) ;
#25470=ORIENTED_EDGE('',*,*,#17688,.F.) ;
#25471=ORIENTED_EDGE('',*,*,#18094,.T.) ;
#25472=ORIENTED_EDGE('',*,*,#18095,.F.) ;
#25473=ORIENTED_EDGE('',*,*,#17689,.F.) ;
#25474=ORIENTED_EDGE('',*,*,#18096,.F.) ;
#25475=ORIENTED_EDGE('',*,*,#18094,.F.) ;
#25476=ORIENTED_EDGE('',*,*,#17687,.F.) ;
#25477=ORIENTED_EDGE('',*,*,#18095,.T.) ;
#25478=ORIENTED_EDGE('',*,*,#18096,.T.) ;
#25479=ORIENTED_EDGE('',*,*,#17691,.F.) ;
#25480=ORIENTED_EDGE('',*,*,#18097,.T.) ;
#25481=ORIENTED_EDGE('',*,*,#18098,.F.) ;
#25482=ORIENTED_EDGE('',*,*,#17692,.F.) ;
#25483=ORIENTED_EDGE('',*,*,#18099,.F.) ;
#25484=ORIENTED_EDGE('',*,*,#18097,.F.) ;
#25485=ORIENTED_EDGE('',*,*,#17690,.F.) ;
#25486=ORIENTED_EDGE('',*,*,#18098,.T.) ;
#25487=ORIENTED_EDGE('',*,*,#18099,.T.) ;
#25488=ORIENTED_EDGE('',*,*,#17696,.F.) ;
#25489=ORIENTED_EDGE('',*,*,#18100,.T.) ;
#25490=ORIENTED_EDGE('',*,*,#18101,.F.) ;
#25491=ORIENTED_EDGE('',*,*,#17697,.F.) ;
#25492=ORIENTED_EDGE('',*,*,#18102,.F.) ;
#25493=ORIENTED_EDGE('',*,*,#18100,.F.) ;
#25494=ORIENTED_EDGE('',*,*,#17695,.F.) ;
#25495=ORIENTED_EDGE('',*,*,#17693,.F.) ;
#25496=ORIENTED_EDGE('',*,*,#18101,.T.) ;
#25497=ORIENTED_EDGE('',*,*,#18102,.T.) ;
#25498=ORIENTED_EDGE('',*,*,#17699,.F.) ;
#25499=ORIENTED_EDGE('',*,*,#18103,.T.) ;
#25500=ORIENTED_EDGE('',*,*,#18104,.F.) ;
#25501=ORIENTED_EDGE('',*,*,#17700,.F.) ;
#25502=ORIENTED_EDGE('',*,*,#18105,.F.) ;
#25503=ORIENTED_EDGE('',*,*,#18103,.F.) ;
#25504=ORIENTED_EDGE('',*,*,#17698,.F.) ;
#25505=ORIENTED_EDGE('',*,*,#18104,.T.) ;
#25506=ORIENTED_EDGE('',*,*,#18105,.T.) ;
#25507=ORIENTED_EDGE('',*,*,#17702,.F.) ;
#25508=ORIENTED_EDGE('',*,*,#18106,.T.) ;
#25509=ORIENTED_EDGE('',*,*,#18107,.F.) ;
#25510=ORIENTED_EDGE('',*,*,#17703,.F.) ;
#25511=ORIENTED_EDGE('',*,*,#18108,.F.) ;
#25512=ORIENTED_EDGE('',*,*,#18106,.F.) ;
#25513=ORIENTED_EDGE('',*,*,#17701,.F.) ;
#25514=ORIENTED_EDGE('',*,*,#18107,.T.) ;
#25515=ORIENTED_EDGE('',*,*,#18108,.T.) ;
#25516=ORIENTED_EDGE('',*,*,#17705,.F.) ;
#25517=ORIENTED_EDGE('',*,*,#18109,.T.) ;
#25518=ORIENTED_EDGE('',*,*,#18110,.F.) ;
#25519=ORIENTED_EDGE('',*,*,#17706,.F.) ;
#25520=ORIENTED_EDGE('',*,*,#18111,.F.) ;
#25521=ORIENTED_EDGE('',*,*,#18109,.F.) ;
#25522=ORIENTED_EDGE('',*,*,#17704,.F.) ;
#25523=ORIENTED_EDGE('',*,*,#18110,.T.) ;
#25524=ORIENTED_EDGE('',*,*,#18111,.T.) ;
#25525=ORIENTED_EDGE('',*,*,#17710,.F.) ;
#25526=ORIENTED_EDGE('',*,*,#18112,.T.) ;
#25527=ORIENTED_EDGE('',*,*,#18113,.F.) ;
#25528=ORIENTED_EDGE('',*,*,#17711,.F.) ;
#25529=ORIENTED_EDGE('',*,*,#18114,.F.) ;
#25530=ORIENTED_EDGE('',*,*,#18112,.F.) ;
#25531=ORIENTED_EDGE('',*,*,#17709,.F.) ;
#25532=ORIENTED_EDGE('',*,*,#17707,.F.) ;
#25533=ORIENTED_EDGE('',*,*,#18113,.T.) ;
#25534=ORIENTED_EDGE('',*,*,#18114,.T.) ;
#25535=ORIENTED_EDGE('',*,*,#17713,.F.) ;
#25536=ORIENTED_EDGE('',*,*,#18115,.T.) ;
#25537=ORIENTED_EDGE('',*,*,#18116,.F.) ;
#25538=ORIENTED_EDGE('',*,*,#17714,.F.) ;
#25539=ORIENTED_EDGE('',*,*,#18117,.F.) ;
#25540=ORIENTED_EDGE('',*,*,#18115,.F.) ;
#25541=ORIENTED_EDGE('',*,*,#17712,.F.) ;
#25542=ORIENTED_EDGE('',*,*,#18116,.T.) ;
#25543=ORIENTED_EDGE('',*,*,#18117,.T.) ;
#25544=ORIENTED_EDGE('',*,*,#17716,.F.) ;
#25545=ORIENTED_EDGE('',*,*,#18118,.T.) ;
#25546=ORIENTED_EDGE('',*,*,#18119,.F.) ;
#25547=ORIENTED_EDGE('',*,*,#17717,.F.) ;
#25548=ORIENTED_EDGE('',*,*,#18120,.F.) ;
#25549=ORIENTED_EDGE('',*,*,#18118,.F.) ;
#25550=ORIENTED_EDGE('',*,*,#17715,.F.) ;
#25551=ORIENTED_EDGE('',*,*,#18119,.T.) ;
#25552=ORIENTED_EDGE('',*,*,#18120,.T.) ;
#25553=ORIENTED_EDGE('',*,*,#17719,.F.) ;
#25554=ORIENTED_EDGE('',*,*,#18121,.T.) ;
#25555=ORIENTED_EDGE('',*,*,#18122,.F.) ;
#25556=ORIENTED_EDGE('',*,*,#17720,.F.) ;
#25557=ORIENTED_EDGE('',*,*,#18123,.F.) ;
#25558=ORIENTED_EDGE('',*,*,#18121,.F.) ;
#25559=ORIENTED_EDGE('',*,*,#17718,.F.) ;
#25560=ORIENTED_EDGE('',*,*,#18122,.T.) ;
#25561=ORIENTED_EDGE('',*,*,#18123,.T.) ;
#25562=ORIENTED_EDGE('',*,*,#17724,.F.) ;
#25563=ORIENTED_EDGE('',*,*,#18124,.T.) ;
#25564=ORIENTED_EDGE('',*,*,#18125,.F.) ;
#25565=ORIENTED_EDGE('',*,*,#17725,.F.) ;
#25566=ORIENTED_EDGE('',*,*,#18126,.F.) ;
#25567=ORIENTED_EDGE('',*,*,#18124,.F.) ;
#25568=ORIENTED_EDGE('',*,*,#17723,.F.) ;
#25569=ORIENTED_EDGE('',*,*,#17721,.F.) ;
#25570=ORIENTED_EDGE('',*,*,#18125,.T.) ;
#25571=ORIENTED_EDGE('',*,*,#18126,.T.) ;
#25572=ORIENTED_EDGE('',*,*,#17727,.F.) ;
#25573=ORIENTED_EDGE('',*,*,#18127,.T.) ;
#25574=ORIENTED_EDGE('',*,*,#18128,.F.) ;
#25575=ORIENTED_EDGE('',*,*,#17728,.F.) ;
#25576=ORIENTED_EDGE('',*,*,#18129,.F.) ;
#25577=ORIENTED_EDGE('',*,*,#18127,.F.) ;
#25578=ORIENTED_EDGE('',*,*,#17726,.F.) ;
#25579=ORIENTED_EDGE('',*,*,#18128,.T.) ;
#25580=ORIENTED_EDGE('',*,*,#18129,.T.) ;
#25581=ORIENTED_EDGE('',*,*,#17730,.F.) ;
#25582=ORIENTED_EDGE('',*,*,#18130,.T.) ;
#25583=ORIENTED_EDGE('',*,*,#18131,.F.) ;
#25584=ORIENTED_EDGE('',*,*,#17731,.F.) ;
#25585=ORIENTED_EDGE('',*,*,#18132,.F.) ;
#25586=ORIENTED_EDGE('',*,*,#18130,.F.) ;
#25587=ORIENTED_EDGE('',*,*,#17729,.F.) ;
#25588=ORIENTED_EDGE('',*,*,#18131,.T.) ;
#25589=ORIENTED_EDGE('',*,*,#18132,.T.) ;
#25590=ORIENTED_EDGE('',*,*,#17733,.F.) ;
#25591=ORIENTED_EDGE('',*,*,#18133,.T.) ;
#25592=ORIENTED_EDGE('',*,*,#18134,.F.) ;
#25593=ORIENTED_EDGE('',*,*,#17734,.F.) ;
#25594=ORIENTED_EDGE('',*,*,#18135,.F.) ;
#25595=ORIENTED_EDGE('',*,*,#18133,.F.) ;
#25596=ORIENTED_EDGE('',*,*,#17732,.F.) ;
#25597=ORIENTED_EDGE('',*,*,#18134,.T.) ;
#25598=ORIENTED_EDGE('',*,*,#18135,.T.) ;
#25599=ORIENTED_EDGE('',*,*,#17738,.F.) ;
#25600=ORIENTED_EDGE('',*,*,#18136,.T.) ;
#25601=ORIENTED_EDGE('',*,*,#18137,.F.) ;
#25602=ORIENTED_EDGE('',*,*,#17739,.F.) ;
#25603=ORIENTED_EDGE('',*,*,#18138,.F.) ;
#25604=ORIENTED_EDGE('',*,*,#18136,.F.) ;
#25605=ORIENTED_EDGE('',*,*,#17737,.F.) ;
#25606=ORIENTED_EDGE('',*,*,#17735,.F.) ;
#25607=ORIENTED_EDGE('',*,*,#18137,.T.) ;
#25608=ORIENTED_EDGE('',*,*,#18138,.T.) ;
#25609=ORIENTED_EDGE('',*,*,#17741,.F.) ;
#25610=ORIENTED_EDGE('',*,*,#18139,.T.) ;
#25611=ORIENTED_EDGE('',*,*,#18140,.F.) ;
#25612=ORIENTED_EDGE('',*,*,#17742,.F.) ;
#25613=ORIENTED_EDGE('',*,*,#18141,.F.) ;
#25614=ORIENTED_EDGE('',*,*,#18139,.F.) ;
#25615=ORIENTED_EDGE('',*,*,#17740,.F.) ;
#25616=ORIENTED_EDGE('',*,*,#18140,.T.) ;
#25617=ORIENTED_EDGE('',*,*,#18141,.T.) ;
#25618=ORIENTED_EDGE('',*,*,#17744,.F.) ;
#25619=ORIENTED_EDGE('',*,*,#18142,.T.) ;
#25620=ORIENTED_EDGE('',*,*,#18143,.F.) ;
#25621=ORIENTED_EDGE('',*,*,#17745,.F.) ;
#25622=ORIENTED_EDGE('',*,*,#18144,.F.) ;
#25623=ORIENTED_EDGE('',*,*,#18142,.F.) ;
#25624=ORIENTED_EDGE('',*,*,#17743,.F.) ;
#25625=ORIENTED_EDGE('',*,*,#18143,.T.) ;
#25626=ORIENTED_EDGE('',*,*,#18144,.T.) ;
#25627=ORIENTED_EDGE('',*,*,#17747,.F.) ;
#25628=ORIENTED_EDGE('',*,*,#18145,.T.) ;
#25629=ORIENTED_EDGE('',*,*,#18146,.F.) ;
#25630=ORIENTED_EDGE('',*,*,#17748,.F.) ;
#25631=ORIENTED_EDGE('',*,*,#18147,.F.) ;
#25632=ORIENTED_EDGE('',*,*,#18145,.F.) ;
#25633=ORIENTED_EDGE('',*,*,#17746,.F.) ;
#25634=ORIENTED_EDGE('',*,*,#18146,.T.) ;
#25635=ORIENTED_EDGE('',*,*,#18147,.T.) ;
#25636=ORIENTED_EDGE('',*,*,#17752,.F.) ;
#25637=ORIENTED_EDGE('',*,*,#18148,.T.) ;
#25638=ORIENTED_EDGE('',*,*,#18149,.F.) ;
#25639=ORIENTED_EDGE('',*,*,#17753,.F.) ;
#25640=ORIENTED_EDGE('',*,*,#18150,.F.) ;
#25641=ORIENTED_EDGE('',*,*,#18148,.F.) ;
#25642=ORIENTED_EDGE('',*,*,#17751,.F.) ;
#25643=ORIENTED_EDGE('',*,*,#17749,.F.) ;
#25644=ORIENTED_EDGE('',*,*,#18149,.T.) ;
#25645=ORIENTED_EDGE('',*,*,#18150,.T.) ;
#25646=ORIENTED_EDGE('',*,*,#17755,.F.) ;
#25647=ORIENTED_EDGE('',*,*,#18151,.T.) ;
#25648=ORIENTED_EDGE('',*,*,#18152,.F.) ;
#25649=ORIENTED_EDGE('',*,*,#17756,.F.) ;
#25650=ORIENTED_EDGE('',*,*,#18153,.F.) ;
#25651=ORIENTED_EDGE('',*,*,#18151,.F.) ;
#25652=ORIENTED_EDGE('',*,*,#17754,.F.) ;
#25653=ORIENTED_EDGE('',*,*,#18152,.T.) ;
#25654=ORIENTED_EDGE('',*,*,#18153,.T.) ;
#25655=ORIENTED_EDGE('',*,*,#17758,.F.) ;
#25656=ORIENTED_EDGE('',*,*,#18154,.T.) ;
#25657=ORIENTED_EDGE('',*,*,#18155,.F.) ;
#25658=ORIENTED_EDGE('',*,*,#17759,.F.) ;
#25659=ORIENTED_EDGE('',*,*,#18156,.F.) ;
#25660=ORIENTED_EDGE('',*,*,#18154,.F.) ;
#25661=ORIENTED_EDGE('',*,*,#17757,.F.) ;
#25662=ORIENTED_EDGE('',*,*,#18155,.T.) ;
#25663=ORIENTED_EDGE('',*,*,#18156,.T.) ;
#25664=ORIENTED_EDGE('',*,*,#17761,.F.) ;
#25665=ORIENTED_EDGE('',*,*,#18157,.T.) ;
#25666=ORIENTED_EDGE('',*,*,#18158,.F.) ;
#25667=ORIENTED_EDGE('',*,*,#17762,.F.) ;
#25668=ORIENTED_EDGE('',*,*,#18159,.F.) ;
#25669=ORIENTED_EDGE('',*,*,#18157,.F.) ;
#25670=ORIENTED_EDGE('',*,*,#17760,.F.) ;
#25671=ORIENTED_EDGE('',*,*,#18158,.T.) ;
#25672=ORIENTED_EDGE('',*,*,#18159,.T.) ;
#25673=ORIENTED_EDGE('',*,*,#17766,.F.) ;
#25674=ORIENTED_EDGE('',*,*,#18160,.T.) ;
#25675=ORIENTED_EDGE('',*,*,#18161,.F.) ;
#25676=ORIENTED_EDGE('',*,*,#17767,.F.) ;
#25677=ORIENTED_EDGE('',*,*,#18162,.F.) ;
#25678=ORIENTED_EDGE('',*,*,#18160,.F.) ;
#25679=ORIENTED_EDGE('',*,*,#17765,.F.) ;
#25680=ORIENTED_EDGE('',*,*,#17763,.F.) ;
#25681=ORIENTED_EDGE('',*,*,#18161,.T.) ;
#25682=ORIENTED_EDGE('',*,*,#18162,.T.) ;
#25683=ORIENTED_EDGE('',*,*,#17769,.F.) ;
#25684=ORIENTED_EDGE('',*,*,#18163,.T.) ;
#25685=ORIENTED_EDGE('',*,*,#18164,.F.) ;
#25686=ORIENTED_EDGE('',*,*,#17770,.F.) ;
#25687=ORIENTED_EDGE('',*,*,#18165,.F.) ;
#25688=ORIENTED_EDGE('',*,*,#18163,.F.) ;
#25689=ORIENTED_EDGE('',*,*,#17768,.F.) ;
#25690=ORIENTED_EDGE('',*,*,#18164,.T.) ;
#25691=ORIENTED_EDGE('',*,*,#18165,.T.) ;
#25692=ORIENTED_EDGE('',*,*,#17772,.F.) ;
#25693=ORIENTED_EDGE('',*,*,#18166,.T.) ;
#25694=ORIENTED_EDGE('',*,*,#18167,.F.) ;
#25695=ORIENTED_EDGE('',*,*,#17773,.F.) ;
#25696=ORIENTED_EDGE('',*,*,#18168,.F.) ;
#25697=ORIENTED_EDGE('',*,*,#18166,.F.) ;
#25698=ORIENTED_EDGE('',*,*,#17771,.F.) ;
#25699=ORIENTED_EDGE('',*,*,#18167,.T.) ;
#25700=ORIENTED_EDGE('',*,*,#18168,.T.) ;
#25701=ORIENTED_EDGE('',*,*,#17775,.F.) ;
#25702=ORIENTED_EDGE('',*,*,#18169,.T.) ;
#25703=ORIENTED_EDGE('',*,*,#18170,.F.) ;
#25704=ORIENTED_EDGE('',*,*,#17776,.F.) ;
#25705=ORIENTED_EDGE('',*,*,#18171,.F.) ;
#25706=ORIENTED_EDGE('',*,*,#18169,.F.) ;
#25707=ORIENTED_EDGE('',*,*,#17774,.F.) ;
#25708=ORIENTED_EDGE('',*,*,#18170,.T.) ;
#25709=ORIENTED_EDGE('',*,*,#18171,.T.) ;
#25710=ORIENTED_EDGE('',*,*,#17780,.F.) ;
#25711=ORIENTED_EDGE('',*,*,#18172,.T.) ;
#25712=ORIENTED_EDGE('',*,*,#18173,.F.) ;
#25713=ORIENTED_EDGE('',*,*,#17781,.F.) ;
#25714=ORIENTED_EDGE('',*,*,#18174,.F.) ;
#25715=ORIENTED_EDGE('',*,*,#18172,.F.) ;
#25716=ORIENTED_EDGE('',*,*,#17779,.F.) ;
#25717=ORIENTED_EDGE('',*,*,#17777,.F.) ;
#25718=ORIENTED_EDGE('',*,*,#18173,.T.) ;
#25719=ORIENTED_EDGE('',*,*,#18174,.T.) ;
#25720=ORIENTED_EDGE('',*,*,#17783,.F.) ;
#25721=ORIENTED_EDGE('',*,*,#18175,.T.) ;
#25722=ORIENTED_EDGE('',*,*,#18176,.F.) ;
#25723=ORIENTED_EDGE('',*,*,#17784,.F.) ;
#25724=ORIENTED_EDGE('',*,*,#18177,.F.) ;
#25725=ORIENTED_EDGE('',*,*,#18175,.F.) ;
#25726=ORIENTED_EDGE('',*,*,#17782,.F.) ;
#25727=ORIENTED_EDGE('',*,*,#18176,.T.) ;
#25728=ORIENTED_EDGE('',*,*,#18177,.T.) ;
#25729=ORIENTED_EDGE('',*,*,#17786,.F.) ;
#25730=ORIENTED_EDGE('',*,*,#18178,.T.) ;
#25731=ORIENTED_EDGE('',*,*,#18179,.F.) ;
#25732=ORIENTED_EDGE('',*,*,#17787,.F.) ;
#25733=ORIENTED_EDGE('',*,*,#18180,.F.) ;
#25734=ORIENTED_EDGE('',*,*,#18178,.F.) ;
#25735=ORIENTED_EDGE('',*,*,#17785,.F.) ;
#25736=ORIENTED_EDGE('',*,*,#18179,.T.) ;
#25737=ORIENTED_EDGE('',*,*,#18180,.T.) ;
#25738=ORIENTED_EDGE('',*,*,#17789,.F.) ;
#25739=ORIENTED_EDGE('',*,*,#18181,.T.) ;
#25740=ORIENTED_EDGE('',*,*,#18182,.F.) ;
#25741=ORIENTED_EDGE('',*,*,#17790,.F.) ;
#25742=ORIENTED_EDGE('',*,*,#18183,.F.) ;
#25743=ORIENTED_EDGE('',*,*,#18181,.F.) ;
#25744=ORIENTED_EDGE('',*,*,#17788,.F.) ;
#25745=ORIENTED_EDGE('',*,*,#18182,.T.) ;
#25746=ORIENTED_EDGE('',*,*,#18183,.T.) ;
#25747=ORIENTED_EDGE('',*,*,#17794,.F.) ;
#25748=ORIENTED_EDGE('',*,*,#18184,.T.) ;
#25749=ORIENTED_EDGE('',*,*,#18185,.F.) ;
#25750=ORIENTED_EDGE('',*,*,#17795,.F.) ;
#25751=ORIENTED_EDGE('',*,*,#18186,.F.) ;
#25752=ORIENTED_EDGE('',*,*,#18184,.F.) ;
#25753=ORIENTED_EDGE('',*,*,#17793,.F.) ;
#25754=ORIENTED_EDGE('',*,*,#17791,.F.) ;
#25755=ORIENTED_EDGE('',*,*,#18185,.T.) ;
#25756=ORIENTED_EDGE('',*,*,#18186,.T.) ;
#25757=ORIENTED_EDGE('',*,*,#17797,.F.) ;
#25758=ORIENTED_EDGE('',*,*,#18187,.T.) ;
#25759=ORIENTED_EDGE('',*,*,#18188,.F.) ;
#25760=ORIENTED_EDGE('',*,*,#17798,.F.) ;
#25761=ORIENTED_EDGE('',*,*,#18189,.F.) ;
#25762=ORIENTED_EDGE('',*,*,#18187,.F.) ;
#25763=ORIENTED_EDGE('',*,*,#17796,.F.) ;
#25764=ORIENTED_EDGE('',*,*,#18188,.T.) ;
#25765=ORIENTED_EDGE('',*,*,#18189,.T.) ;
#25766=ORIENTED_EDGE('',*,*,#17800,.F.) ;
#25767=ORIENTED_EDGE('',*,*,#18190,.T.) ;
#25768=ORIENTED_EDGE('',*,*,#18191,.F.) ;
#25769=ORIENTED_EDGE('',*,*,#17801,.F.) ;
#25770=ORIENTED_EDGE('',*,*,#18192,.F.) ;
#25771=ORIENTED_EDGE('',*,*,#18190,.F.) ;
#25772=ORIENTED_EDGE('',*,*,#17799,.F.) ;
#25773=ORIENTED_EDGE('',*,*,#18191,.T.) ;
#25774=ORIENTED_EDGE('',*,*,#18192,.T.) ;
#25775=ORIENTED_EDGE('',*,*,#17803,.F.) ;
#25776=ORIENTED_EDGE('',*,*,#18193,.T.) ;
#25777=ORIENTED_EDGE('',*,*,#18194,.F.) ;
#25778=ORIENTED_EDGE('',*,*,#17804,.F.) ;
#25779=ORIENTED_EDGE('',*,*,#18195,.F.) ;
#25780=ORIENTED_EDGE('',*,*,#18193,.F.) ;
#25781=ORIENTED_EDGE('',*,*,#17802,.F.) ;
#25782=ORIENTED_EDGE('',*,*,#18194,.T.) ;
#25783=ORIENTED_EDGE('',*,*,#18195,.T.) ;
#25784=ORIENTED_EDGE('',*,*,#17808,.F.) ;
#25785=ORIENTED_EDGE('',*,*,#18196,.T.) ;
#25786=ORIENTED_EDGE('',*,*,#18197,.F.) ;
#25787=ORIENTED_EDGE('',*,*,#17809,.F.) ;
#25788=ORIENTED_EDGE('',*,*,#18198,.F.) ;
#25789=ORIENTED_EDGE('',*,*,#18196,.F.) ;
#25790=ORIENTED_EDGE('',*,*,#17807,.F.) ;
#25791=ORIENTED_EDGE('',*,*,#17805,.F.) ;
#25792=ORIENTED_EDGE('',*,*,#18197,.T.) ;
#25793=ORIENTED_EDGE('',*,*,#18198,.T.) ;
#25794=ORIENTED_EDGE('',*,*,#17811,.F.) ;
#25795=ORIENTED_EDGE('',*,*,#18199,.T.) ;
#25796=ORIENTED_EDGE('',*,*,#18200,.F.) ;
#25797=ORIENTED_EDGE('',*,*,#17812,.F.) ;
#25798=ORIENTED_EDGE('',*,*,#18201,.F.) ;
#25799=ORIENTED_EDGE('',*,*,#18199,.F.) ;
#25800=ORIENTED_EDGE('',*,*,#17810,.F.) ;
#25801=ORIENTED_EDGE('',*,*,#18200,.T.) ;
#25802=ORIENTED_EDGE('',*,*,#18201,.T.) ;
#25803=ORIENTED_EDGE('',*,*,#17814,.F.) ;
#25804=ORIENTED_EDGE('',*,*,#18202,.T.) ;
#25805=ORIENTED_EDGE('',*,*,#18203,.F.) ;
#25806=ORIENTED_EDGE('',*,*,#17815,.F.) ;
#25807=ORIENTED_EDGE('',*,*,#18204,.F.) ;
#25808=ORIENTED_EDGE('',*,*,#18202,.F.) ;
#25809=ORIENTED_EDGE('',*,*,#17813,.F.) ;
#25810=ORIENTED_EDGE('',*,*,#18203,.T.) ;
#25811=ORIENTED_EDGE('',*,*,#18204,.T.) ;
#25812=ORIENTED_EDGE('',*,*,#17817,.F.) ;
#25813=ORIENTED_EDGE('',*,*,#18205,.T.) ;
#25814=ORIENTED_EDGE('',*,*,#18206,.F.) ;
#25815=ORIENTED_EDGE('',*,*,#17818,.F.) ;
#25816=ORIENTED_EDGE('',*,*,#18207,.F.) ;
#25817=ORIENTED_EDGE('',*,*,#18205,.F.) ;
#25818=ORIENTED_EDGE('',*,*,#17816,.F.) ;
#25819=ORIENTED_EDGE('',*,*,#18206,.T.) ;
#25820=ORIENTED_EDGE('',*,*,#18207,.T.) ;
#25821=ORIENTED_EDGE('',*,*,#17822,.F.) ;
#25822=ORIENTED_EDGE('',*,*,#18208,.T.) ;
#25823=ORIENTED_EDGE('',*,*,#18209,.F.) ;
#25824=ORIENTED_EDGE('',*,*,#17823,.F.) ;
#25825=ORIENTED_EDGE('',*,*,#18210,.F.) ;
#25826=ORIENTED_EDGE('',*,*,#18208,.F.) ;
#25827=ORIENTED_EDGE('',*,*,#17821,.F.) ;
#25828=ORIENTED_EDGE('',*,*,#17819,.F.) ;
#25829=ORIENTED_EDGE('',*,*,#18209,.T.) ;
#25830=ORIENTED_EDGE('',*,*,#18210,.T.) ;
#25831=ORIENTED_EDGE('',*,*,#17825,.F.) ;
#25832=ORIENTED_EDGE('',*,*,#18211,.T.) ;
#25833=ORIENTED_EDGE('',*,*,#18212,.F.) ;
#25834=ORIENTED_EDGE('',*,*,#17826,.F.) ;
#25835=ORIENTED_EDGE('',*,*,#18213,.F.) ;
#25836=ORIENTED_EDGE('',*,*,#18211,.F.) ;
#25837=ORIENTED_EDGE('',*,*,#17824,.F.) ;
#25838=ORIENTED_EDGE('',*,*,#18212,.T.) ;
#25839=ORIENTED_EDGE('',*,*,#18213,.T.) ;
#25840=ORIENTED_EDGE('',*,*,#17828,.F.) ;
#25841=ORIENTED_EDGE('',*,*,#18214,.T.) ;
#25842=ORIENTED_EDGE('',*,*,#18215,.F.) ;
#25843=ORIENTED_EDGE('',*,*,#17829,.F.) ;
#25844=ORIENTED_EDGE('',*,*,#18216,.F.) ;
#25845=ORIENTED_EDGE('',*,*,#18214,.F.) ;
#25846=ORIENTED_EDGE('',*,*,#17827,.F.) ;
#25847=ORIENTED_EDGE('',*,*,#18215,.T.) ;
#25848=ORIENTED_EDGE('',*,*,#18216,.T.) ;
#25849=ORIENTED_EDGE('',*,*,#17831,.F.) ;
#25850=ORIENTED_EDGE('',*,*,#18217,.T.) ;
#25851=ORIENTED_EDGE('',*,*,#18218,.F.) ;
#25852=ORIENTED_EDGE('',*,*,#17832,.F.) ;
#25853=ORIENTED_EDGE('',*,*,#18219,.F.) ;
#25854=ORIENTED_EDGE('',*,*,#18217,.F.) ;
#25855=ORIENTED_EDGE('',*,*,#17830,.F.) ;
#25856=ORIENTED_EDGE('',*,*,#18218,.T.) ;
#25857=ORIENTED_EDGE('',*,*,#18219,.T.) ;
#25858=ORIENTED_EDGE('',*,*,#17836,.F.) ;
#25859=ORIENTED_EDGE('',*,*,#18220,.T.) ;
#25860=ORIENTED_EDGE('',*,*,#18221,.F.) ;
#25861=ORIENTED_EDGE('',*,*,#17837,.F.) ;
#25862=ORIENTED_EDGE('',*,*,#18222,.F.) ;
#25863=ORIENTED_EDGE('',*,*,#18220,.F.) ;
#25864=ORIENTED_EDGE('',*,*,#17835,.F.) ;
#25865=ORIENTED_EDGE('',*,*,#17833,.F.) ;
#25866=ORIENTED_EDGE('',*,*,#18221,.T.) ;
#25867=ORIENTED_EDGE('',*,*,#18222,.T.) ;
#25868=ORIENTED_EDGE('',*,*,#17839,.F.) ;
#25869=ORIENTED_EDGE('',*,*,#18223,.T.) ;
#25870=ORIENTED_EDGE('',*,*,#18224,.F.) ;
#25871=ORIENTED_EDGE('',*,*,#17840,.F.) ;
#25872=ORIENTED_EDGE('',*,*,#18225,.F.) ;
#25873=ORIENTED_EDGE('',*,*,#18223,.F.) ;
#25874=ORIENTED_EDGE('',*,*,#17838,.F.) ;
#25875=ORIENTED_EDGE('',*,*,#18224,.T.) ;
#25876=ORIENTED_EDGE('',*,*,#18225,.T.) ;
#25877=ORIENTED_EDGE('',*,*,#17842,.F.) ;
#25878=ORIENTED_EDGE('',*,*,#18226,.T.) ;
#25879=ORIENTED_EDGE('',*,*,#18227,.F.) ;
#25880=ORIENTED_EDGE('',*,*,#17843,.F.) ;
#25881=ORIENTED_EDGE('',*,*,#18228,.F.) ;
#25882=ORIENTED_EDGE('',*,*,#18226,.F.) ;
#25883=ORIENTED_EDGE('',*,*,#17841,.F.) ;
#25884=ORIENTED_EDGE('',*,*,#18227,.T.) ;
#25885=ORIENTED_EDGE('',*,*,#18228,.T.) ;
#25886=ORIENTED_EDGE('',*,*,#17845,.F.) ;
#25887=ORIENTED_EDGE('',*,*,#18229,.T.) ;
#25888=ORIENTED_EDGE('',*,*,#18230,.F.) ;
#25889=ORIENTED_EDGE('',*,*,#17846,.F.) ;
#25890=ORIENTED_EDGE('',*,*,#18231,.F.) ;
#25891=ORIENTED_EDGE('',*,*,#18229,.F.) ;
#25892=ORIENTED_EDGE('',*,*,#17844,.F.) ;
#25893=ORIENTED_EDGE('',*,*,#18230,.T.) ;
#25894=ORIENTED_EDGE('',*,*,#18231,.T.) ;
#25895=ORIENTED_EDGE('',*,*,#17850,.F.) ;
#25896=ORIENTED_EDGE('',*,*,#18232,.T.) ;
#25897=ORIENTED_EDGE('',*,*,#18233,.F.) ;
#25898=ORIENTED_EDGE('',*,*,#17851,.F.) ;
#25899=ORIENTED_EDGE('',*,*,#18234,.F.) ;
#25900=ORIENTED_EDGE('',*,*,#18232,.F.) ;
#25901=ORIENTED_EDGE('',*,*,#17849,.F.) ;
#25902=ORIENTED_EDGE('',*,*,#17847,.F.) ;
#25903=ORIENTED_EDGE('',*,*,#18233,.T.) ;
#25904=ORIENTED_EDGE('',*,*,#18234,.T.) ;
#25905=ORIENTED_EDGE('',*,*,#17853,.F.) ;
#25906=ORIENTED_EDGE('',*,*,#18235,.T.) ;
#25907=ORIENTED_EDGE('',*,*,#18236,.F.) ;
#25908=ORIENTED_EDGE('',*,*,#17854,.F.) ;
#25909=ORIENTED_EDGE('',*,*,#18237,.F.) ;
#25910=ORIENTED_EDGE('',*,*,#18235,.F.) ;
#25911=ORIENTED_EDGE('',*,*,#17852,.F.) ;
#25912=ORIENTED_EDGE('',*,*,#18236,.T.) ;
#25913=ORIENTED_EDGE('',*,*,#18237,.T.) ;
#25914=ORIENTED_EDGE('',*,*,#17856,.F.) ;
#25915=ORIENTED_EDGE('',*,*,#18238,.T.) ;
#25916=ORIENTED_EDGE('',*,*,#18239,.F.) ;
#25917=ORIENTED_EDGE('',*,*,#17857,.F.) ;
#25918=ORIENTED_EDGE('',*,*,#18240,.F.) ;
#25919=ORIENTED_EDGE('',*,*,#18238,.F.) ;
#25920=ORIENTED_EDGE('',*,*,#17855,.F.) ;
#25921=ORIENTED_EDGE('',*,*,#18239,.T.) ;
#25922=ORIENTED_EDGE('',*,*,#18240,.T.) ;
#25923=ORIENTED_EDGE('',*,*,#17859,.F.) ;
#25924=ORIENTED_EDGE('',*,*,#18241,.T.) ;
#25925=ORIENTED_EDGE('',*,*,#18242,.F.) ;
#25926=ORIENTED_EDGE('',*,*,#17860,.F.) ;
#25927=ORIENTED_EDGE('',*,*,#18243,.F.) ;
#25928=ORIENTED_EDGE('',*,*,#18241,.F.) ;
#25929=ORIENTED_EDGE('',*,*,#17858,.F.) ;
#25930=ORIENTED_EDGE('',*,*,#18242,.T.) ;
#25931=ORIENTED_EDGE('',*,*,#18243,.T.) ;
#25932=ORIENTED_EDGE('',*,*,#17864,.F.) ;
#25933=ORIENTED_EDGE('',*,*,#18244,.T.) ;
#25934=ORIENTED_EDGE('',*,*,#18245,.F.) ;
#25935=ORIENTED_EDGE('',*,*,#17865,.F.) ;
#25936=ORIENTED_EDGE('',*,*,#18246,.F.) ;
#25937=ORIENTED_EDGE('',*,*,#18244,.F.) ;
#25938=ORIENTED_EDGE('',*,*,#17863,.F.) ;
#25939=ORIENTED_EDGE('',*,*,#17861,.F.) ;
#25940=ORIENTED_EDGE('',*,*,#18245,.T.) ;
#25941=ORIENTED_EDGE('',*,*,#18246,.T.) ;
#25942=ORIENTED_EDGE('',*,*,#17867,.F.) ;
#25943=ORIENTED_EDGE('',*,*,#18247,.T.) ;
#25944=ORIENTED_EDGE('',*,*,#18248,.F.) ;
#25945=ORIENTED_EDGE('',*,*,#17868,.F.) ;
#25946=ORIENTED_EDGE('',*,*,#18249,.F.) ;
#25947=ORIENTED_EDGE('',*,*,#18247,.F.) ;
#25948=ORIENTED_EDGE('',*,*,#17866,.F.) ;
#25949=ORIENTED_EDGE('',*,*,#18248,.T.) ;
#25950=ORIENTED_EDGE('',*,*,#18249,.T.) ;
#25951=ORIENTED_EDGE('',*,*,#17870,.F.) ;
#25952=ORIENTED_EDGE('',*,*,#18250,.T.) ;
#25953=ORIENTED_EDGE('',*,*,#18251,.F.) ;
#25954=ORIENTED_EDGE('',*,*,#17871,.F.) ;
#25955=ORIENTED_EDGE('',*,*,#18252,.F.) ;
#25956=ORIENTED_EDGE('',*,*,#18250,.F.) ;
#25957=ORIENTED_EDGE('',*,*,#17869,.F.) ;
#25958=ORIENTED_EDGE('',*,*,#18251,.T.) ;
#25959=ORIENTED_EDGE('',*,*,#18252,.T.) ;
#25960=ORIENTED_EDGE('',*,*,#17873,.F.) ;
#25961=ORIENTED_EDGE('',*,*,#18253,.T.) ;
#25962=ORIENTED_EDGE('',*,*,#18254,.F.) ;
#25963=ORIENTED_EDGE('',*,*,#17874,.F.) ;
#25964=ORIENTED_EDGE('',*,*,#18255,.F.) ;
#25965=ORIENTED_EDGE('',*,*,#18253,.F.) ;
#25966=ORIENTED_EDGE('',*,*,#17872,.F.) ;
#25967=ORIENTED_EDGE('',*,*,#18254,.T.) ;
#25968=ORIENTED_EDGE('',*,*,#18255,.T.) ;
#25969=ORIENTED_EDGE('',*,*,#17878,.F.) ;
#25970=ORIENTED_EDGE('',*,*,#18256,.T.) ;
#25971=ORIENTED_EDGE('',*,*,#18257,.F.) ;
#25972=ORIENTED_EDGE('',*,*,#17879,.F.) ;
#25973=ORIENTED_EDGE('',*,*,#18258,.F.) ;
#25974=ORIENTED_EDGE('',*,*,#18256,.F.) ;
#25975=ORIENTED_EDGE('',*,*,#17877,.F.) ;
#25976=ORIENTED_EDGE('',*,*,#17875,.F.) ;
#25977=ORIENTED_EDGE('',*,*,#18257,.T.) ;
#25978=ORIENTED_EDGE('',*,*,#18258,.T.) ;
#25979=ORIENTED_EDGE('',*,*,#17881,.F.) ;
#25980=ORIENTED_EDGE('',*,*,#18259,.T.) ;
#25981=ORIENTED_EDGE('',*,*,#18260,.F.) ;
#25982=ORIENTED_EDGE('',*,*,#17882,.F.) ;
#25983=ORIENTED_EDGE('',*,*,#18261,.F.) ;
#25984=ORIENTED_EDGE('',*,*,#18259,.F.) ;
#25985=ORIENTED_EDGE('',*,*,#17880,.F.) ;
#25986=ORIENTED_EDGE('',*,*,#18260,.T.) ;
#25987=ORIENTED_EDGE('',*,*,#18261,.T.) ;
#25988=ORIENTED_EDGE('',*,*,#17884,.F.) ;
#25989=ORIENTED_EDGE('',*,*,#18262,.T.) ;
#25990=ORIENTED_EDGE('',*,*,#18263,.F.) ;
#25991=ORIENTED_EDGE('',*,*,#17885,.F.) ;
#25992=ORIENTED_EDGE('',*,*,#18264,.F.) ;
#25993=ORIENTED_EDGE('',*,*,#18262,.F.) ;
#25994=ORIENTED_EDGE('',*,*,#17883,.F.) ;
#25995=ORIENTED_EDGE('',*,*,#18263,.T.) ;
#25996=ORIENTED_EDGE('',*,*,#18264,.T.) ;
#25997=ORIENTED_EDGE('',*,*,#17887,.F.) ;
#25998=ORIENTED_EDGE('',*,*,#18265,.T.) ;
#25999=ORIENTED_EDGE('',*,*,#18266,.F.) ;
#26000=ORIENTED_EDGE('',*,*,#18265,.F.) ;
#26001=ORIENTED_EDGE('',*,*,#17886,.F.) ;
#26002=ORIENTED_EDGE('',*,*,#18266,.T.) ;
#26003=ORIENTED_EDGE('',*,*,#18267,.F.) ;
#26004=ORIENTED_EDGE('',*,*,#18268,.T.) ;
#26005=ORIENTED_EDGE('',*,*,#18269,.F.) ;
#26006=ORIENTED_EDGE('',*,*,#18270,.T.) ;
#26007=ORIENTED_EDGE('',*,*,#18271,.F.) ;
#26008=ORIENTED_EDGE('',*,*,#18270,.F.) ;
#26009=ORIENTED_EDGE('',*,*,#18272,.F.) ;
#26010=ORIENTED_EDGE('',*,*,#18273,.F.) ;
#26011=ORIENTED_EDGE('',*,*,#18268,.F.) ;
#26012=ORIENTED_EDGE('',*,*,#18274,.F.) ;
#26013=ORIENTED_EDGE('',*,*,#18275,.T.) ;
#26014=ORIENTED_EDGE('',*,*,#18276,.F.) ;
#26015=ORIENTED_EDGE('',*,*,#18275,.F.) ;
#26016=ORIENTED_EDGE('',*,*,#18271,.T.) ;
#26017=ORIENTED_EDGE('',*,*,#18274,.T.) ;
#26018=ORIENTED_EDGE('',*,*,#18267,.T.) ;
#26019=ORIENTED_EDGE('',*,*,#18276,.T.) ;
#26020=ORIENTED_EDGE('',*,*,#18272,.T.) ;
#26021=ORIENTED_EDGE('',*,*,#18277,.T.) ;
#26022=ORIENTED_EDGE('',*,*,#18278,.F.) ;
#26023=ORIENTED_EDGE('',*,*,#18277,.F.) ;
#26024=ORIENTED_EDGE('',*,*,#18269,.T.) ;
#26025=ORIENTED_EDGE('',*,*,#18273,.T.) ;
#26026=ORIENTED_EDGE('',*,*,#18278,.T.) ;
#26895=CYLINDRICAL_SURFACE('',#31070,0.55) ;
#26896=CYLINDRICAL_SURFACE('',#31073,0.25) ;
#26897=CYLINDRICAL_SURFACE('',#31078,0.15) ;
#26898=CYLINDRICAL_SURFACE('',#31081,0.8) ;
#26899=CYLINDRICAL_SURFACE('',#31084,1.1) ;
#26900=CYLINDRICAL_SURFACE('',#31089,0.8) ;
#26901=CYLINDRICAL_SURFACE('',#31093,1.1) ;
#26902=CYLINDRICAL_SURFACE('',#31674,0.15) ;
#26903=CYLINDRICAL_SURFACE('',#31676,0.15) ;
#26904=CYLINDRICAL_SURFACE('',#31678,0.15) ;
#26905=CYLINDRICAL_SURFACE('',#31681,0.15) ;
#26906=CYLINDRICAL_SURFACE('',#31684,0.15) ;
#26907=CYLINDRICAL_SURFACE('',#31687,0.15) ;
#26908=CYLINDRICAL_SURFACE('',#31690,0.15) ;
#26909=CYLINDRICAL_SURFACE('',#31693,0.15) ;
#26910=CYLINDRICAL_SURFACE('',#31696,0.15) ;
#26911=CYLINDRICAL_SURFACE('',#31699,0.15) ;
#26912=CYLINDRICAL_SURFACE('',#31702,0.15) ;
#26913=CYLINDRICAL_SURFACE('',#31705,0.15) ;
#26914=CYLINDRICAL_SURFACE('',#31708,0.15) ;
#26915=CYLINDRICAL_SURFACE('',#31711,0.15) ;
#26916=CYLINDRICAL_SURFACE('',#31714,0.15) ;
#26917=CYLINDRICAL_SURFACE('',#31717,0.15) ;
#26918=CYLINDRICAL_SURFACE('',#31720,0.15) ;
#26919=CYLINDRICAL_SURFACE('',#31723,0.15) ;
#26920=CYLINDRICAL_SURFACE('',#31726,0.15) ;
#26921=CYLINDRICAL_SURFACE('',#31729,0.15) ;
#26922=CYLINDRICAL_SURFACE('',#31732,0.15) ;
#26923=CYLINDRICAL_SURFACE('',#31735,0.15) ;
#26924=CYLINDRICAL_SURFACE('',#31738,0.15) ;
#26925=CYLINDRICAL_SURFACE('',#31741,0.15) ;
#26926=CYLINDRICAL_SURFACE('',#31744,0.15) ;
#26927=CYLINDRICAL_SURFACE('',#31747,0.15) ;
#26928=CYLINDRICAL_SURFACE('',#31750,0.15) ;
#26929=CYLINDRICAL_SURFACE('',#31753,0.15) ;
#26930=CYLINDRICAL_SURFACE('',#31756,0.15) ;
#26931=CYLINDRICAL_SURFACE('',#31759,0.15) ;
#26932=CYLINDRICAL_SURFACE('',#31762,0.15) ;
#26933=CYLINDRICAL_SURFACE('',#31765,0.15) ;
#26934=CYLINDRICAL_SURFACE('',#31768,0.15) ;
#26935=CYLINDRICAL_SURFACE('',#31771,0.15) ;
#26936=CYLINDRICAL_SURFACE('',#31774,0.15) ;
#26937=CYLINDRICAL_SURFACE('',#31777,0.15) ;
#26938=CYLINDRICAL_SURFACE('',#31780,0.15) ;
#26939=CYLINDRICAL_SURFACE('',#31783,0.15) ;
#26940=CYLINDRICAL_SURFACE('',#31786,0.15) ;
#26941=CYLINDRICAL_SURFACE('',#31789,0.15) ;
#26942=CYLINDRICAL_SURFACE('',#31792,0.15) ;
#26943=CYLINDRICAL_SURFACE('',#31795,0.15) ;
#26944=CYLINDRICAL_SURFACE('',#31798,0.15) ;
#26945=CYLINDRICAL_SURFACE('',#31801,0.15) ;
#26946=CYLINDRICAL_SURFACE('',#31804,0.15) ;
#26947=CYLINDRICAL_SURFACE('',#31807,0.15) ;
#26948=CYLINDRICAL_SURFACE('',#31810,0.15) ;
#26949=CYLINDRICAL_SURFACE('',#31813,0.15) ;
#26950=CYLINDRICAL_SURFACE('',#31816,0.15) ;
#26951=CYLINDRICAL_SURFACE('',#31819,0.15) ;
#26952=CYLINDRICAL_SURFACE('',#31822,0.15) ;
#26953=CYLINDRICAL_SURFACE('',#31825,0.15) ;
#26954=CYLINDRICAL_SURFACE('',#31828,0.15) ;
#26955=CYLINDRICAL_SURFACE('',#31831,0.15) ;
#26956=CYLINDRICAL_SURFACE('',#31834,0.15) ;
#26957=CYLINDRICAL_SURFACE('',#31837,0.15) ;
#26958=CYLINDRICAL_SURFACE('',#31840,0.15) ;
#26959=CYLINDRICAL_SURFACE('',#31843,0.15) ;
#26960=CYLINDRICAL_SURFACE('',#31846,0.15) ;
#26961=CYLINDRICAL_SURFACE('',#31849,0.15) ;
#26962=CYLINDRICAL_SURFACE('',#31852,0.15) ;
#26963=CYLINDRICAL_SURFACE('',#31855,0.15) ;
#26964=CYLINDRICAL_SURFACE('',#31858,0.15) ;
#26965=CYLINDRICAL_SURFACE('',#31861,0.15) ;
#26966=CYLINDRICAL_SURFACE('',#31864,0.15) ;
#26967=CYLINDRICAL_SURFACE('',#31867,0.15) ;
#26968=CYLINDRICAL_SURFACE('',#31870,0.15) ;
#26969=CYLINDRICAL_SURFACE('',#31873,0.15) ;
#26970=CYLINDRICAL_SURFACE('',#31876,0.15) ;
#26971=CYLINDRICAL_SURFACE('',#31879,0.15) ;
#26972=CYLINDRICAL_SURFACE('',#31882,0.15) ;
#26973=CYLINDRICAL_SURFACE('',#31885,0.15) ;
#26974=CYLINDRICAL_SURFACE('',#31888,0.15) ;
#26975=CYLINDRICAL_SURFACE('',#31891,0.15) ;
#26976=CYLINDRICAL_SURFACE('',#31894,0.15) ;
#26977=CYLINDRICAL_SURFACE('',#31897,0.15) ;
#26978=CYLINDRICAL_SURFACE('',#31900,0.15) ;
#26979=CYLINDRICAL_SURFACE('',#31903,0.15) ;
#26980=CYLINDRICAL_SURFACE('',#31906,0.15) ;
#26981=CYLINDRICAL_SURFACE('',#31909,0.15) ;
#26982=CYLINDRICAL_SURFACE('',#31912,0.15) ;
#26983=CYLINDRICAL_SURFACE('',#31915,0.15) ;
#26984=CYLINDRICAL_SURFACE('',#31918,0.15) ;
#26985=CYLINDRICAL_SURFACE('',#31921,0.15) ;
#26986=CYLINDRICAL_SURFACE('',#31924,0.15) ;
#26987=CYLINDRICAL_SURFACE('',#31927,0.15) ;
#26988=CYLINDRICAL_SURFACE('',#31930,0.15) ;
#26989=CYLINDRICAL_SURFACE('',#31933,0.15) ;
#26990=CYLINDRICAL_SURFACE('',#31936,0.15) ;
#26991=CYLINDRICAL_SURFACE('',#31939,0.15) ;
#26992=CYLINDRICAL_SURFACE('',#31942,0.15) ;
#26993=CYLINDRICAL_SURFACE('',#31945,0.15) ;
#26994=CYLINDRICAL_SURFACE('',#31948,0.15) ;
#26995=CYLINDRICAL_SURFACE('',#31951,0.15) ;
#26996=CYLINDRICAL_SURFACE('',#31954,0.15) ;
#26997=CYLINDRICAL_SURFACE('',#31957,0.15) ;
#26998=CYLINDRICAL_SURFACE('',#31960,0.15) ;
#26999=CYLINDRICAL_SURFACE('',#31963,0.15) ;
#27000=CYLINDRICAL_SURFACE('',#31966,0.15) ;
#27001=CYLINDRICAL_SURFACE('',#31969,0.15) ;
#27002=CYLINDRICAL_SURFACE('',#31972,0.15) ;
#27003=CYLINDRICAL_SURFACE('',#31975,0.15) ;
#27004=CYLINDRICAL_SURFACE('',#31978,0.15) ;
#27005=CYLINDRICAL_SURFACE('',#31981,0.15) ;
#27006=CYLINDRICAL_SURFACE('',#31984,0.15) ;
#27007=CYLINDRICAL_SURFACE('',#31987,0.15) ;
#27008=CYLINDRICAL_SURFACE('',#31990,0.15) ;
#27009=CYLINDRICAL_SURFACE('',#31993,0.15) ;
#27010=CYLINDRICAL_SURFACE('',#31996,0.15) ;
#27011=CYLINDRICAL_SURFACE('',#31999,0.15) ;
#27012=CYLINDRICAL_SURFACE('',#32002,0.15) ;
#27013=CYLINDRICAL_SURFACE('',#32005,0.15) ;
#27014=CYLINDRICAL_SURFACE('',#32008,0.15) ;
#27015=CYLINDRICAL_SURFACE('',#32011,0.15) ;
#27016=CYLINDRICAL_SURFACE('',#32014,0.15) ;
#27017=CYLINDRICAL_SURFACE('',#32017,0.15) ;
#27018=CYLINDRICAL_SURFACE('',#32020,0.15) ;
#27019=CYLINDRICAL_SURFACE('',#32023,0.15) ;
#27020=CYLINDRICAL_SURFACE('',#32026,0.15) ;
#27021=CYLINDRICAL_SURFACE('',#32029,0.15) ;
#27022=CYLINDRICAL_SURFACE('',#32032,0.15) ;
#27023=CYLINDRICAL_SURFACE('',#32035,0.15) ;
#27024=CYLINDRICAL_SURFACE('',#32038,0.15) ;
#27025=CYLINDRICAL_SURFACE('',#32041,0.15) ;
#27026=CYLINDRICAL_SURFACE('',#32044,0.15) ;
#27027=CYLINDRICAL_SURFACE('',#32047,0.15) ;
#27028=CYLINDRICAL_SURFACE('',#32050,0.15) ;
#27029=CYLINDRICAL_SURFACE('',#32053,0.15) ;
#27030=CYLINDRICAL_SURFACE('',#32056,0.55) ;
#27031=CYLINDRICAL_SURFACE('',#32059,0.25) ;
#27032=CYLINDRICAL_SURFACE('',#32064,0.15) ;
#28210=ADVANCED_FACE('',(#3475,#1379),#26895,.T.) ;
#28211=ADVANCED_FACE('',(#3476),#26896,.F.) ;
#28212=ADVANCED_FACE('',(#3477,#1380),#2244,.T.) ;
#28213=ADVANCED_FACE('',(#3478,#1381),#2245,.T.) ;
#28214=ADVANCED_FACE('',(#3479),#26897,.T.) ;
#28215=ADVANCED_FACE('',(#3480),#2246,.T.) ;
#28216=ADVANCED_FACE('',(#3481),#26898,.F.) ;
#28217=ADVANCED_FACE('',(#3482),#26899,.T.) ;
#28218=ADVANCED_FACE('',(#3483,#1382),#2247,.T.) ;
#28219=ADVANCED_FACE('',(#3484,#1383),#2248,.T.) ;
#28220=ADVANCED_FACE('',(#3485),#26900,.F.) ;
#28221=ADVANCED_FACE('',(#3486),#26901,.T.) ;
#28222=ADVANCED_FACE('',(#3487,#1384),#2249,.T.) ;
#28223=ADVANCED_FACE('',(#3488,#1385),#2250,.T.) ;
#28224=ADVANCED_FACE('',(#3489),#2251,.T.) ;
#28225=ADVANCED_FACE('',(#3490),#748,.T.) ;
#28226=ADVANCED_FACE('',(#3491),#749,.T.) ;
#28227=ADVANCED_FACE('',(#3492),#750,.T.) ;
#28228=ADVANCED_FACE('',(#3493),#751,.T.) ;
#28229=ADVANCED_FACE('',(#3494),#752,.T.) ;
#28230=ADVANCED_FACE('',(#3495),#753,.T.) ;
#28231=ADVANCED_FACE('',(#3496),#754,.T.) ;
#28232=ADVANCED_FACE('',(#3497),#755,.T.) ;
#28233=ADVANCED_FACE('',(#3498),#756,.T.) ;
#28234=ADVANCED_FACE('',(#3499),#757,.T.) ;
#28235=ADVANCED_FACE('',(#3500),#758,.T.) ;
#28236=ADVANCED_FACE('',(#3501),#759,.T.) ;
#28237=ADVANCED_FACE('',(#3502),#760,.T.) ;
#28238=ADVANCED_FACE('',(#3503),#761,.T.) ;
#28239=ADVANCED_FACE('',(#3504),#762,.T.) ;
#28240=ADVANCED_FACE('',(#3505),#763,.T.) ;
#28241=ADVANCED_FACE('',(#3506),#764,.T.) ;
#28242=ADVANCED_FACE('',(#3507),#765,.T.) ;
#28243=ADVANCED_FACE('',(#3508),#766,.T.) ;
#28244=ADVANCED_FACE('',(#3509),#767,.T.) ;
#28245=ADVANCED_FACE('',(#3510),#768,.T.) ;
#28246=ADVANCED_FACE('',(#3511),#769,.T.) ;
#28247=ADVANCED_FACE('',(#3512),#770,.T.) ;
#28248=ADVANCED_FACE('',(#3513),#771,.T.) ;
#28249=ADVANCED_FACE('',(#3514),#772,.T.) ;
#28250=ADVANCED_FACE('',(#3515),#773,.T.) ;
#28251=ADVANCED_FACE('',(#3516),#774,.T.) ;
#28252=ADVANCED_FACE('',(#3517),#775,.T.) ;
#28253=ADVANCED_FACE('',(#3518),#776,.T.) ;
#28254=ADVANCED_FACE('',(#3519),#777,.T.) ;
#28255=ADVANCED_FACE('',(#3520),#778,.T.) ;
#28256=ADVANCED_FACE('',(#3521),#779,.T.) ;
#28257=ADVANCED_FACE('',(#3522),#780,.T.) ;
#28258=ADVANCED_FACE('',(#3523),#781,.T.) ;
#28259=ADVANCED_FACE('',(#3524),#782,.T.) ;
#28260=ADVANCED_FACE('',(#3525),#783,.T.) ;
#28261=ADVANCED_FACE('',(#3526),#784,.T.) ;
#28262=ADVANCED_FACE('',(#3527),#785,.T.) ;
#28263=ADVANCED_FACE('',(#3528),#786,.T.) ;
#28264=ADVANCED_FACE('',(#3529),#787,.T.) ;
#28265=ADVANCED_FACE('',(#3530),#788,.T.) ;
#28266=ADVANCED_FACE('',(#3531),#789,.T.) ;
#28267=ADVANCED_FACE('',(#3532),#790,.T.) ;
#28268=ADVANCED_FACE('',(#3533),#791,.T.) ;
#28269=ADVANCED_FACE('',(#3534),#792,.T.) ;
#28270=ADVANCED_FACE('',(#3535),#793,.T.) ;
#28271=ADVANCED_FACE('',(#3536),#794,.T.) ;
#28272=ADVANCED_FACE('',(#3537),#795,.T.) ;
#28273=ADVANCED_FACE('',(#3538),#796,.T.) ;
#28274=ADVANCED_FACE('',(#3539),#797,.T.) ;
#28275=ADVANCED_FACE('',(#3540),#798,.T.) ;
#28276=ADVANCED_FACE('',(#3541),#799,.T.) ;
#28277=ADVANCED_FACE('',(#3542),#800,.T.) ;
#28278=ADVANCED_FACE('',(#3543),#801,.T.) ;
#28279=ADVANCED_FACE('',(#3544),#802,.T.) ;
#28280=ADVANCED_FACE('',(#3545),#803,.T.) ;
#28281=ADVANCED_FACE('',(#3546),#804,.T.) ;
#28282=ADVANCED_FACE('',(#3547),#805,.T.) ;
#28283=ADVANCED_FACE('',(#3548),#806,.T.) ;
#28284=ADVANCED_FACE('',(#3549),#807,.T.) ;
#28285=ADVANCED_FACE('',(#3550),#808,.T.) ;
#28286=ADVANCED_FACE('',(#3551),#809,.T.) ;
#28287=ADVANCED_FACE('',(#3552),#810,.T.) ;
#28288=ADVANCED_FACE('',(#3553),#811,.T.) ;
#28289=ADVANCED_FACE('',(#3554),#812,.T.) ;
#28290=ADVANCED_FACE('',(#3555),#813,.T.) ;
#28291=ADVANCED_FACE('',(#3556),#814,.T.) ;
#28292=ADVANCED_FACE('',(#3557),#815,.T.) ;
#28293=ADVANCED_FACE('',(#3558),#816,.T.) ;
#28294=ADVANCED_FACE('',(#3559),#817,.T.) ;
#28295=ADVANCED_FACE('',(#3560),#818,.T.) ;
#28296=ADVANCED_FACE('',(#3561),#819,.T.) ;
#28297=ADVANCED_FACE('',(#3562),#820,.T.) ;
#28298=ADVANCED_FACE('',(#3563),#821,.T.) ;
#28299=ADVANCED_FACE('',(#3564),#822,.T.) ;
#28300=ADVANCED_FACE('',(#3565),#823,.T.) ;
#28301=ADVANCED_FACE('',(#3566),#824,.T.) ;
#28302=ADVANCED_FACE('',(#3567),#825,.T.) ;
#28303=ADVANCED_FACE('',(#3568),#826,.T.) ;
#28304=ADVANCED_FACE('',(#3569),#827,.T.) ;
#28305=ADVANCED_FACE('',(#3570),#828,.T.) ;
#28306=ADVANCED_FACE('',(#3571),#829,.T.) ;
#28307=ADVANCED_FACE('',(#3572),#830,.T.) ;
#28308=ADVANCED_FACE('',(#3573),#831,.T.) ;
#28309=ADVANCED_FACE('',(#3574),#832,.T.) ;
#28310=ADVANCED_FACE('',(#3575),#833,.T.) ;
#28311=ADVANCED_FACE('',(#3576),#834,.T.) ;
#28312=ADVANCED_FACE('',(#3577),#835,.T.) ;
#28313=ADVANCED_FACE('',(#3578),#836,.T.) ;
#28314=ADVANCED_FACE('',(#3579),#837,.T.) ;
#28315=ADVANCED_FACE('',(#3580),#838,.T.) ;
#28316=ADVANCED_FACE('',(#3581),#839,.T.) ;
#28317=ADVANCED_FACE('',(#3582),#840,.T.) ;
#28318=ADVANCED_FACE('',(#3583),#841,.T.) ;
#28319=ADVANCED_FACE('',(#3584),#842,.T.) ;
#28320=ADVANCED_FACE('',(#3585),#843,.T.) ;
#28321=ADVANCED_FACE('',(#3586),#844,.T.) ;
#28322=ADVANCED_FACE('',(#3587),#845,.T.) ;
#28323=ADVANCED_FACE('',(#3588),#846,.T.) ;
#28324=ADVANCED_FACE('',(#3589),#847,.T.) ;
#28325=ADVANCED_FACE('',(#3590),#848,.T.) ;
#28326=ADVANCED_FACE('',(#3591),#849,.T.) ;
#28327=ADVANCED_FACE('',(#3592),#850,.T.) ;
#28328=ADVANCED_FACE('',(#3593),#851,.T.) ;
#28329=ADVANCED_FACE('',(#3594),#852,.T.) ;
#28330=ADVANCED_FACE('',(#3595),#853,.T.) ;
#28331=ADVANCED_FACE('',(#3596),#854,.T.) ;
#28332=ADVANCED_FACE('',(#3597),#855,.T.) ;
#28333=ADVANCED_FACE('',(#3598),#856,.T.) ;
#28334=ADVANCED_FACE('',(#3599),#857,.T.) ;
#28335=ADVANCED_FACE('',(#3600),#858,.T.) ;
#28336=ADVANCED_FACE('',(#3601),#859,.T.) ;
#28337=ADVANCED_FACE('',(#3602),#860,.T.) ;
#28338=ADVANCED_FACE('',(#3603),#861,.T.) ;
#28339=ADVANCED_FACE('',(#3604),#862,.T.) ;
#28340=ADVANCED_FACE('',(#3605),#863,.T.) ;
#28341=ADVANCED_FACE('',(#3606),#864,.T.) ;
#28342=ADVANCED_FACE('',(#3607),#865,.T.) ;
#28343=ADVANCED_FACE('',(#3608),#866,.T.) ;
#28344=ADVANCED_FACE('',(#3609),#867,.T.) ;
#28345=ADVANCED_FACE('',(#3610),#868,.T.) ;
#28346=ADVANCED_FACE('',(#3611),#869,.T.) ;
#28347=ADVANCED_FACE('',(#3612),#870,.T.) ;
#28348=ADVANCED_FACE('',(#3613),#871,.T.) ;
#28349=ADVANCED_FACE('',(#3614),#872,.T.) ;
#28350=ADVANCED_FACE('',(#3615),#873,.T.) ;
#28351=ADVANCED_FACE('',(#3616),#874,.T.) ;
#28352=ADVANCED_FACE('',(#3617),#26902,.T.) ;
#28353=ADVANCED_FACE('',(#3618),#26903,.T.) ;
#28354=ADVANCED_FACE('',(#3619),#26904,.T.) ;
#28355=ADVANCED_FACE('',(#3620),#26905,.T.) ;
#28356=ADVANCED_FACE('',(#3621),#26906,.T.) ;
#28357=ADVANCED_FACE('',(#3622),#26907,.T.) ;
#28358=ADVANCED_FACE('',(#3623),#26908,.T.) ;
#28359=ADVANCED_FACE('',(#3624),#26909,.T.) ;
#28360=ADVANCED_FACE('',(#3625),#26910,.T.) ;
#28361=ADVANCED_FACE('',(#3626),#26911,.T.) ;
#28362=ADVANCED_FACE('',(#3627),#26912,.T.) ;
#28363=ADVANCED_FACE('',(#3628),#26913,.T.) ;
#28364=ADVANCED_FACE('',(#3629),#26914,.T.) ;
#28365=ADVANCED_FACE('',(#3630),#26915,.T.) ;
#28366=ADVANCED_FACE('',(#3631),#26916,.T.) ;
#28367=ADVANCED_FACE('',(#3632),#26917,.T.) ;
#28368=ADVANCED_FACE('',(#3633),#26918,.T.) ;
#28369=ADVANCED_FACE('',(#3634),#26919,.T.) ;
#28370=ADVANCED_FACE('',(#3635),#26920,.T.) ;
#28371=ADVANCED_FACE('',(#3636),#26921,.T.) ;
#28372=ADVANCED_FACE('',(#3637),#26922,.T.) ;
#28373=ADVANCED_FACE('',(#3638),#26923,.T.) ;
#28374=ADVANCED_FACE('',(#3639),#26924,.T.) ;
#28375=ADVANCED_FACE('',(#3640),#26925,.T.) ;
#28376=ADVANCED_FACE('',(#3641),#26926,.T.) ;
#28377=ADVANCED_FACE('',(#3642),#26927,.T.) ;
#28378=ADVANCED_FACE('',(#3643),#26928,.T.) ;
#28379=ADVANCED_FACE('',(#3644),#26929,.T.) ;
#28380=ADVANCED_FACE('',(#3645),#26930,.T.) ;
#28381=ADVANCED_FACE('',(#3646),#26931,.T.) ;
#28382=ADVANCED_FACE('',(#3647),#26932,.T.) ;
#28383=ADVANCED_FACE('',(#3648),#26933,.T.) ;
#28384=ADVANCED_FACE('',(#3649),#26934,.T.) ;
#28385=ADVANCED_FACE('',(#3650),#26935,.T.) ;
#28386=ADVANCED_FACE('',(#3651),#26936,.T.) ;
#28387=ADVANCED_FACE('',(#3652),#26937,.T.) ;
#28388=ADVANCED_FACE('',(#3653),#26938,.T.) ;
#28389=ADVANCED_FACE('',(#3654),#26939,.T.) ;
#28390=ADVANCED_FACE('',(#3655),#26940,.T.) ;
#28391=ADVANCED_FACE('',(#3656),#26941,.T.) ;
#28392=ADVANCED_FACE('',(#3657),#26942,.T.) ;
#28393=ADVANCED_FACE('',(#3658),#26943,.T.) ;
#28394=ADVANCED_FACE('',(#3659),#26944,.T.) ;
#28395=ADVANCED_FACE('',(#3660),#26945,.T.) ;
#28396=ADVANCED_FACE('',(#3661),#26946,.T.) ;
#28397=ADVANCED_FACE('',(#3662),#26947,.T.) ;
#28398=ADVANCED_FACE('',(#3663),#26948,.T.) ;
#28399=ADVANCED_FACE('',(#3664),#26949,.T.) ;
#28400=ADVANCED_FACE('',(#3665),#26950,.T.) ;
#28401=ADVANCED_FACE('',(#3666),#26951,.T.) ;
#28402=ADVANCED_FACE('',(#3667),#26952,.T.) ;
#28403=ADVANCED_FACE('',(#3668),#26953,.T.) ;
#28404=ADVANCED_FACE('',(#3669),#26954,.T.) ;
#28405=ADVANCED_FACE('',(#3670),#26955,.T.) ;
#28406=ADVANCED_FACE('',(#3671),#26956,.T.) ;
#28407=ADVANCED_FACE('',(#3672),#26957,.T.) ;
#28408=ADVANCED_FACE('',(#3673),#26958,.T.) ;
#28409=ADVANCED_FACE('',(#3674),#26959,.T.) ;
#28410=ADVANCED_FACE('',(#3675),#26960,.T.) ;
#28411=ADVANCED_FACE('',(#3676),#26961,.T.) ;
#28412=ADVANCED_FACE('',(#3677),#26962,.T.) ;
#28413=ADVANCED_FACE('',(#3678),#26963,.T.) ;
#28414=ADVANCED_FACE('',(#3679),#26964,.T.) ;
#28415=ADVANCED_FACE('',(#3680),#26965,.T.) ;
#28416=ADVANCED_FACE('',(#3681),#26966,.T.) ;
#28417=ADVANCED_FACE('',(#3682),#26967,.T.) ;
#28418=ADVANCED_FACE('',(#3683),#26968,.T.) ;
#28419=ADVANCED_FACE('',(#3684),#26969,.T.) ;
#28420=ADVANCED_FACE('',(#3685),#26970,.T.) ;
#28421=ADVANCED_FACE('',(#3686),#26971,.T.) ;
#28422=ADVANCED_FACE('',(#3687),#26972,.T.) ;
#28423=ADVANCED_FACE('',(#3688),#26973,.T.) ;
#28424=ADVANCED_FACE('',(#3689),#26974,.T.) ;
#28425=ADVANCED_FACE('',(#3690),#26975,.T.) ;
#28426=ADVANCED_FACE('',(#3691),#26976,.T.) ;
#28427=ADVANCED_FACE('',(#3692),#26977,.T.) ;
#28428=ADVANCED_FACE('',(#3693),#26978,.T.) ;
#28429=ADVANCED_FACE('',(#3694),#26979,.T.) ;
#28430=ADVANCED_FACE('',(#3695),#26980,.T.) ;
#28431=ADVANCED_FACE('',(#3696),#26981,.T.) ;
#28432=ADVANCED_FACE('',(#3697),#26982,.T.) ;
#28433=ADVANCED_FACE('',(#3698),#26983,.T.) ;
#28434=ADVANCED_FACE('',(#3699),#26984,.T.) ;
#28435=ADVANCED_FACE('',(#3700),#26985,.T.) ;
#28436=ADVANCED_FACE('',(#3701),#26986,.T.) ;
#28437=ADVANCED_FACE('',(#3702),#26987,.T.) ;
#28438=ADVANCED_FACE('',(#3703),#26988,.T.) ;
#28439=ADVANCED_FACE('',(#3704),#26989,.T.) ;
#28440=ADVANCED_FACE('',(#3705),#26990,.T.) ;
#28441=ADVANCED_FACE('',(#3706),#26991,.T.) ;
#28442=ADVANCED_FACE('',(#3707),#26992,.T.) ;
#28443=ADVANCED_FACE('',(#3708),#26993,.T.) ;
#28444=ADVANCED_FACE('',(#3709),#26994,.T.) ;
#28445=ADVANCED_FACE('',(#3710),#26995,.T.) ;
#28446=ADVANCED_FACE('',(#3711),#26996,.T.) ;
#28447=ADVANCED_FACE('',(#3712),#26997,.T.) ;
#28448=ADVANCED_FACE('',(#3713),#26998,.T.) ;
#28449=ADVANCED_FACE('',(#3714),#26999,.T.) ;
#28450=ADVANCED_FACE('',(#3715),#27000,.T.) ;
#28451=ADVANCED_FACE('',(#3716),#27001,.T.) ;
#28452=ADVANCED_FACE('',(#3717),#27002,.T.) ;
#28453=ADVANCED_FACE('',(#3718),#27003,.T.) ;
#28454=ADVANCED_FACE('',(#3719),#27004,.T.) ;
#28455=ADVANCED_FACE('',(#3720),#27005,.T.) ;
#28456=ADVANCED_FACE('',(#3721),#27006,.T.) ;
#28457=ADVANCED_FACE('',(#3722),#27007,.T.) ;
#28458=ADVANCED_FACE('',(#3723),#27008,.T.) ;
#28459=ADVANCED_FACE('',(#3724),#27009,.T.) ;
#28460=ADVANCED_FACE('',(#3725),#27010,.T.) ;
#28461=ADVANCED_FACE('',(#3726),#27011,.T.) ;
#28462=ADVANCED_FACE('',(#3727),#27012,.T.) ;
#28463=ADVANCED_FACE('',(#3728),#27013,.T.) ;
#28464=ADVANCED_FACE('',(#3729),#27014,.T.) ;
#28465=ADVANCED_FACE('',(#3730),#27015,.T.) ;
#28466=ADVANCED_FACE('',(#3731),#27016,.T.) ;
#28467=ADVANCED_FACE('',(#3732),#27017,.T.) ;
#28468=ADVANCED_FACE('',(#3733),#27018,.T.) ;
#28469=ADVANCED_FACE('',(#3734),#27019,.T.) ;
#28470=ADVANCED_FACE('',(#3735),#27020,.T.) ;
#28471=ADVANCED_FACE('',(#3736),#27021,.T.) ;
#28472=ADVANCED_FACE('',(#3737),#27022,.T.) ;
#28473=ADVANCED_FACE('',(#3738),#27023,.T.) ;
#28474=ADVANCED_FACE('',(#3739),#27024,.T.) ;
#28475=ADVANCED_FACE('',(#3740),#27025,.T.) ;
#28476=ADVANCED_FACE('',(#3741),#27026,.T.) ;
#28477=ADVANCED_FACE('',(#3742),#27027,.T.) ;
#28478=ADVANCED_FACE('',(#3743),#27028,.T.) ;
#28479=ADVANCED_FACE('',(#3744),#27029,.T.) ;
#28480=ADVANCED_FACE('',(#3745),#2252,.T.) ;
#28481=ADVANCED_FACE('',(#3746),#27030,.T.) ;
#28482=ADVANCED_FACE('',(#3747),#27031,.F.) ;
#28483=ADVANCED_FACE('',(#3748,#1386),#2253,.T.) ;
#28484=ADVANCED_FACE('',(#3749,#1387),#2254,.T.) ;
#28485=ADVANCED_FACE('',(#3750),#27032,.T.) ;
#28486=ADVANCED_FACE('',(#3751),#2255,.T.) ;
#28693=CLOSED_SHELL('',(#28210,#28211,#28212,#28213,#28214,#28215)) ;
#28694=CLOSED_SHELL('',(#28216,#28217,#28218,#28219)) ;
#28695=CLOSED_SHELL('',(#28220,#28221,#28222,#28223,#28224,#28225,#28226,
#28227,#28228,#28229,#28230,#28231,#28232,#28233,#28234,#28235,#28236,#28237,
#28238,#28239,#28240,#28241,#28242,#28243,#28244,#28245,#28246,#28247,#28248,
#28249,#28250,#28251,#28252,#28253,#28254,#28255,#28256,#28257,#28258,#28259,
#28260,#28261,#28262,#28263,#28264,#28265,#28266,#28267,#28268,#28269,#28270,
#28271,#28272,#28273,#28274,#28275,#28276,#28277,#28278,#28279,#28280,#28281,
#28282,#28283,#28284,#28285,#28286,#28287,#28288,#28289,#28290,#28291,#28292,
#28293,#28294,#28295,#28296,#28297,#28298,#28299,#28300,#28301,#28302,#28303,
#28304,#28305,#28306,#28307,#28308,#28309,#28310,#28311,#28312,#28313,#28314,
#28315,#28316,#28317,#28318,#28319,#28320,#28321,#28322,#28323,#28324,#28325,
#28326,#28327,#28328,#28329,#28330,#28331,#28332,#28333,#28334,#28335,#28336,
#28337,#28338,#28339,#28340,#28341,#28342,#28343,#28344,#28345,#28346,#28347,
#28348,#28349,#28350,#28351,#28352,#28353,#28354,#28355,#28356,#28357,#28358,
#28359,#28360,#28361,#28362,#28363,#28364,#28365,#28366,#28367,#28368,#28369,
#28370,#28371,#28372,#28373,#28374,#28375,#28376,#28377,#28378,#28379,#28380,
#28381,#28382,#28383,#28384,#28385,#28386,#28387,#28388,#28389,#28390,#28391,
#28392,#28393,#28394,#28395,#28396,#28397,#28398,#28399,#28400,#28401,#28402,
#28403,#28404,#28405,#28406,#28407,#28408,#28409,#28410,#28411,#28412,#28413,
#28414,#28415,#28416,#28417,#28418,#28419,#28420,#28421,#28422,#28423,#28424,
#28425,#28426,#28427,#28428,#28429,#28430,#28431,#28432,#28433,#28434,#28435,
#28436,#28437,#28438,#28439,#28440,#28441,#28442,#28443,#28444,#28445,#28446,
#28447,#28448,#28449,#28450,#28451,#28452,#28453,#28454,#28455,#28456,#28457,
#28458,#28459,#28460,#28461,#28462,#28463,#28464,#28465,#28466,#28467,#28468,
#28469,#28470,#28471,#28472,#28473,#28474,#28475,#28476,#28477,#28478,#28479,
#28480)) ;
#28696=CLOSED_SHELL('',(#28481,#28482,#28483,#28484,#28485,#28486)) ;
#31069=AXIS2_PLACEMENT_3D('',#47520,#38264,#38265) ;
#31070=AXIS2_PLACEMENT_3D('',#47521,#38266,#38267) ;
#31071=AXIS2_PLACEMENT_3D('',#47523,#38268,#38269) ;
#31072=AXIS2_PLACEMENT_3D('',#47526,#38271,#38272) ;
#31073=AXIS2_PLACEMENT_3D('',#47565,#38273,#38274) ;
#31074=AXIS2_PLACEMENT_3D('',#47567,#38275,#38276) ;
#31075=AXIS2_PLACEMENT_3D('',#47570,#38278,#38279) ;
#31076=AXIS2_PLACEMENT_3D('',#47571,#38280,#38281) ;
#31077=AXIS2_PLACEMENT_3D('',#47572,#38282,#38283) ;
#31078=AXIS2_PLACEMENT_3D('',#47573,#38284,#38285) ;
#31079=AXIS2_PLACEMENT_3D('',#47575,#38286,#38287) ;
#31080=AXIS2_PLACEMENT_3D('',#47577,#38289,#38290) ;
#31081=AXIS2_PLACEMENT_3D('',#47578,#38291,#38292) ;
#31082=AXIS2_PLACEMENT_3D('',#47580,#38293,#38294) ;
#31083=AXIS2_PLACEMENT_3D('',#47583,#38296,#38297) ;
#31084=AXIS2_PLACEMENT_3D('',#47584,#38298,#38299) ;
#31085=AXIS2_PLACEMENT_3D('',#47586,#38300,#38301) ;
#31086=AXIS2_PLACEMENT_3D('',#47589,#38303,#38304) ;
#31087=AXIS2_PLACEMENT_3D('',#47590,#38305,#38306) ;
#31088=AXIS2_PLACEMENT_3D('',#47591,#38307,#38308) ;
#31089=AXIS2_PLACEMENT_3D('',#47592,#38309,#38310) ;
#31090=AXIS2_PLACEMENT_3D('',#47595,#38311,#38312) ;
#31091=AXIS2_PLACEMENT_3D('',#47625,#38313,#38314) ;
#31092=AXIS2_PLACEMENT_3D('',#47628,#38316,#38317) ;
#31093=AXIS2_PLACEMENT_3D('',#47629,#38318,#38319) ;
#31094=AXIS2_PLACEMENT_3D('',#47631,#38320,#38321) ;
#31095=AXIS2_PLACEMENT_3D('',#47634,#38323,#38324) ;
#31096=AXIS2_PLACEMENT_3D('',#47635,#38325,#38326) ;
#31097=AXIS2_PLACEMENT_3D('',#47639,#38328,#38329) ;
#31098=AXIS2_PLACEMENT_3D('',#47641,#38330,#38331) ;
#31099=AXIS2_PLACEMENT_3D('',#47643,#38332,#38333) ;
#31100=AXIS2_PLACEMENT_3D('',#47645,#38334,#38335) ;
#31101=AXIS2_PLACEMENT_3D('',#47646,#38336,#38337) ;
#31102=AXIS2_PLACEMENT_3D('',#47647,#38338,#38339) ;
#31103=AXIS2_PLACEMENT_3D('',#47648,#38340,#38341) ;
#31104=AXIS2_PLACEMENT_3D('',#47649,#38342,#38343) ;
#31105=AXIS2_PLACEMENT_3D('',#47650,#38344,#38345) ;
#31106=AXIS2_PLACEMENT_3D('',#47652,#38346,#38347) ;
#31107=AXIS2_PLACEMENT_3D('',#47653,#38348,#38349) ;
#31108=AXIS2_PLACEMENT_3D('',#47654,#38350,#38351) ;
#31109=AXIS2_PLACEMENT_3D('',#47656,#38352,#38353) ;
#31110=AXIS2_PLACEMENT_3D('',#47658,#38354,#38355) ;
#31111=AXIS2_PLACEMENT_3D('',#47659,#38356,#38357) ;
#31112=AXIS2_PLACEMENT_3D('',#47660,#38358,#38359) ;
#31113=AXIS2_PLACEMENT_3D('',#47663,#38360,#38361) ;
#31114=AXIS2_PLACEMENT_3D('',#47665,#38362,#38363) ;
#31115=AXIS2_PLACEMENT_3D('',#47666,#38364,#38365) ;
#31116=AXIS2_PLACEMENT_3D('',#47667,#38366,#38367) ;
#31117=AXIS2_PLACEMENT_3D('',#47670,#38368,#38369) ;
#31118=AXIS2_PLACEMENT_3D('',#47672,#38370,#38371) ;
#31119=AXIS2_PLACEMENT_3D('',#47674,#38372,#38373) ;
#31120=AXIS2_PLACEMENT_3D('',#47676,#38374,#38375) ;
#31121=AXIS2_PLACEMENT_3D('',#47677,#38376,#38377) ;
#31122=AXIS2_PLACEMENT_3D('',#47678,#38378,#38379) ;
#31123=AXIS2_PLACEMENT_3D('',#47681,#38380,#38381) ;
#31124=AXIS2_PLACEMENT_3D('',#47683,#38382,#38383) ;
#31125=AXIS2_PLACEMENT_3D('',#47684,#38384,#38385) ;
#31126=AXIS2_PLACEMENT_3D('',#47685,#38386,#38387) ;
#31127=AXIS2_PLACEMENT_3D('',#47688,#38388,#38389) ;
#31128=AXIS2_PLACEMENT_3D('',#47690,#38390,#38391) ;
#31129=AXIS2_PLACEMENT_3D('',#47691,#38392,#38393) ;
#31130=AXIS2_PLACEMENT_3D('',#47692,#38394,#38395) ;
#31131=AXIS2_PLACEMENT_3D('',#47695,#38396,#38397) ;
#31132=AXIS2_PLACEMENT_3D('',#47697,#38398,#38399) ;
#31133=AXIS2_PLACEMENT_3D('',#47698,#38400,#38401) ;
#31134=AXIS2_PLACEMENT_3D('',#47699,#38402,#38403) ;
#31135=AXIS2_PLACEMENT_3D('',#47702,#38404,#38405) ;
#31136=AXIS2_PLACEMENT_3D('',#47704,#38406,#38407) ;
#31137=AXIS2_PLACEMENT_3D('',#47706,#38408,#38409) ;
#31138=AXIS2_PLACEMENT_3D('',#47708,#38410,#38411) ;
#31139=AXIS2_PLACEMENT_3D('',#47709,#38412,#38413) ;
#31140=AXIS2_PLACEMENT_3D('',#47710,#38414,#38415) ;
#31141=AXIS2_PLACEMENT_3D('',#47713,#38416,#38417) ;
#31142=AXIS2_PLACEMENT_3D('',#47715,#38418,#38419) ;
#31143=AXIS2_PLACEMENT_3D('',#47716,#38420,#38421) ;
#31144=AXIS2_PLACEMENT_3D('',#47717,#38422,#38423) ;
#31145=AXIS2_PLACEMENT_3D('',#47720,#38424,#38425) ;
#31146=AXIS2_PLACEMENT_3D('',#47722,#38426,#38427) ;
#31147=AXIS2_PLACEMENT_3D('',#47723,#38428,#38429) ;
#31148=AXIS2_PLACEMENT_3D('',#47724,#38430,#38431) ;
#31149=AXIS2_PLACEMENT_3D('',#47727,#38432,#38433) ;
#31150=AXIS2_PLACEMENT_3D('',#47729,#38434,#38435) ;
#31151=AXIS2_PLACEMENT_3D('',#47730,#38436,#38437) ;
#31152=AXIS2_PLACEMENT_3D('',#47731,#38438,#38439) ;
#31153=AXIS2_PLACEMENT_3D('',#47734,#38440,#38441) ;
#31154=AXIS2_PLACEMENT_3D('',#47736,#38442,#38443) ;
#31155=AXIS2_PLACEMENT_3D('',#47738,#38444,#38445) ;
#31156=AXIS2_PLACEMENT_3D('',#47740,#38446,#38447) ;
#31157=AXIS2_PLACEMENT_3D('',#47741,#38448,#38449) ;
#31158=AXIS2_PLACEMENT_3D('',#47742,#38450,#38451) ;
#31159=AXIS2_PLACEMENT_3D('',#47745,#38452,#38453) ;
#31160=AXIS2_PLACEMENT_3D('',#47747,#38454,#38455) ;
#31161=AXIS2_PLACEMENT_3D('',#47748,#38456,#38457) ;
#31162=AXIS2_PLACEMENT_3D('',#47749,#38458,#38459) ;
#31163=AXIS2_PLACEMENT_3D('',#47752,#38460,#38461) ;
#31164=AXIS2_PLACEMENT_3D('',#47754,#38462,#38463) ;
#31165=AXIS2_PLACEMENT_3D('',#47755,#38464,#38465) ;
#31166=AXIS2_PLACEMENT_3D('',#47756,#38466,#38467) ;
#31167=AXIS2_PLACEMENT_3D('',#47759,#38468,#38469) ;
#31168=AXIS2_PLACEMENT_3D('',#47761,#38470,#38471) ;
#31169=AXIS2_PLACEMENT_3D('',#47762,#38472,#38473) ;
#31170=AXIS2_PLACEMENT_3D('',#47763,#38474,#38475) ;
#31171=AXIS2_PLACEMENT_3D('',#47766,#38476,#38477) ;
#31172=AXIS2_PLACEMENT_3D('',#47768,#38478,#38479) ;
#31173=AXIS2_PLACEMENT_3D('',#47770,#38480,#38481) ;
#31174=AXIS2_PLACEMENT_3D('',#47772,#38482,#38483) ;
#31175=AXIS2_PLACEMENT_3D('',#47773,#38484,#38485) ;
#31176=AXIS2_PLACEMENT_3D('',#47774,#38486,#38487) ;
#31177=AXIS2_PLACEMENT_3D('',#47777,#38488,#38489) ;
#31178=AXIS2_PLACEMENT_3D('',#47779,#38490,#38491) ;
#31179=AXIS2_PLACEMENT_3D('',#47780,#38492,#38493) ;
#31180=AXIS2_PLACEMENT_3D('',#47781,#38494,#38495) ;
#31181=AXIS2_PLACEMENT_3D('',#47784,#38496,#38497) ;
#31182=AXIS2_PLACEMENT_3D('',#47786,#38498,#38499) ;
#31183=AXIS2_PLACEMENT_3D('',#47787,#38500,#38501) ;
#31184=AXIS2_PLACEMENT_3D('',#47788,#38502,#38503) ;
#31185=AXIS2_PLACEMENT_3D('',#47791,#38504,#38505) ;
#31186=AXIS2_PLACEMENT_3D('',#47793,#38506,#38507) ;
#31187=AXIS2_PLACEMENT_3D('',#47794,#38508,#38509) ;
#31188=AXIS2_PLACEMENT_3D('',#47795,#38510,#38511) ;
#31189=AXIS2_PLACEMENT_3D('',#47798,#38512,#38513) ;
#31190=AXIS2_PLACEMENT_3D('',#47800,#38514,#38515) ;
#31191=AXIS2_PLACEMENT_3D('',#47802,#38516,#38517) ;
#31192=AXIS2_PLACEMENT_3D('',#47804,#38518,#38519) ;
#31193=AXIS2_PLACEMENT_3D('',#47805,#38520,#38521) ;
#31194=AXIS2_PLACEMENT_3D('',#47806,#38522,#38523) ;
#31195=AXIS2_PLACEMENT_3D('',#47809,#38524,#38525) ;
#31196=AXIS2_PLACEMENT_3D('',#47811,#38526,#38527) ;
#31197=AXIS2_PLACEMENT_3D('',#47812,#38528,#38529) ;
#31198=AXIS2_PLACEMENT_3D('',#47813,#38530,#38531) ;
#31199=AXIS2_PLACEMENT_3D('',#47816,#38532,#38533) ;
#31200=AXIS2_PLACEMENT_3D('',#47818,#38534,#38535) ;
#31201=AXIS2_PLACEMENT_3D('',#47819,#38536,#38537) ;
#31202=AXIS2_PLACEMENT_3D('',#47820,#38538,#38539) ;
#31203=AXIS2_PLACEMENT_3D('',#47823,#38540,#38541) ;
#31204=AXIS2_PLACEMENT_3D('',#47825,#38542,#38543) ;
#31205=AXIS2_PLACEMENT_3D('',#47826,#38544,#38545) ;
#31206=AXIS2_PLACEMENT_3D('',#47827,#38546,#38547) ;
#31207=AXIS2_PLACEMENT_3D('',#47830,#38548,#38549) ;
#31208=AXIS2_PLACEMENT_3D('',#47832,#38550,#38551) ;
#31209=AXIS2_PLACEMENT_3D('',#47834,#38552,#38553) ;
#31210=AXIS2_PLACEMENT_3D('',#47836,#38554,#38555) ;
#31211=AXIS2_PLACEMENT_3D('',#47837,#38556,#38557) ;
#31212=AXIS2_PLACEMENT_3D('',#47838,#38558,#38559) ;
#31213=AXIS2_PLACEMENT_3D('',#47841,#38560,#38561) ;
#31214=AXIS2_PLACEMENT_3D('',#47843,#38562,#38563) ;
#31215=AXIS2_PLACEMENT_3D('',#47844,#38564,#38565) ;
#31216=AXIS2_PLACEMENT_3D('',#47845,#38566,#38567) ;
#31217=AXIS2_PLACEMENT_3D('',#47848,#38568,#38569) ;
#31218=AXIS2_PLACEMENT_3D('',#47850,#38570,#38571) ;
#31219=AXIS2_PLACEMENT_3D('',#47851,#38572,#38573) ;
#31220=AXIS2_PLACEMENT_3D('',#47852,#38574,#38575) ;
#31221=AXIS2_PLACEMENT_3D('',#47855,#38576,#38577) ;
#31222=AXIS2_PLACEMENT_3D('',#47857,#38578,#38579) ;
#31223=AXIS2_PLACEMENT_3D('',#47858,#38580,#38581) ;
#31224=AXIS2_PLACEMENT_3D('',#47859,#38582,#38583) ;
#31225=AXIS2_PLACEMENT_3D('',#47862,#38584,#38585) ;
#31226=AXIS2_PLACEMENT_3D('',#47864,#38586,#38587) ;
#31227=AXIS2_PLACEMENT_3D('',#47866,#38588,#38589) ;
#31228=AXIS2_PLACEMENT_3D('',#47868,#38590,#38591) ;
#31229=AXIS2_PLACEMENT_3D('',#47869,#38592,#38593) ;
#31230=AXIS2_PLACEMENT_3D('',#47870,#38594,#38595) ;
#31231=AXIS2_PLACEMENT_3D('',#47873,#38596,#38597) ;
#31232=AXIS2_PLACEMENT_3D('',#47875,#38598,#38599) ;
#31233=AXIS2_PLACEMENT_3D('',#47876,#38600,#38601) ;
#31234=AXIS2_PLACEMENT_3D('',#47877,#38602,#38603) ;
#31235=AXIS2_PLACEMENT_3D('',#47880,#38604,#38605) ;
#31236=AXIS2_PLACEMENT_3D('',#47882,#38606,#38607) ;
#31237=AXIS2_PLACEMENT_3D('',#47883,#38608,#38609) ;
#31238=AXIS2_PLACEMENT_3D('',#47884,#38610,#38611) ;
#31239=AXIS2_PLACEMENT_3D('',#47887,#38612,#38613) ;
#31240=AXIS2_PLACEMENT_3D('',#47889,#38614,#38615) ;
#31241=AXIS2_PLACEMENT_3D('',#47890,#38616,#38617) ;
#31242=AXIS2_PLACEMENT_3D('',#47891,#38618,#38619) ;
#31243=AXIS2_PLACEMENT_3D('',#47894,#38620,#38621) ;
#31244=AXIS2_PLACEMENT_3D('',#47896,#38622,#38623) ;
#31245=AXIS2_PLACEMENT_3D('',#47898,#38624,#38625) ;
#31246=AXIS2_PLACEMENT_3D('',#47900,#38626,#38627) ;
#31247=AXIS2_PLACEMENT_3D('',#47901,#38628,#38629) ;
#31248=AXIS2_PLACEMENT_3D('',#47902,#38630,#38631) ;
#31249=AXIS2_PLACEMENT_3D('',#47905,#38632,#38633) ;
#31250=AXIS2_PLACEMENT_3D('',#47907,#38634,#38635) ;
#31251=AXIS2_PLACEMENT_3D('',#47908,#38636,#38637) ;
#31252=AXIS2_PLACEMENT_3D('',#47909,#38638,#38639) ;
#31253=AXIS2_PLACEMENT_3D('',#47912,#38640,#38641) ;
#31254=AXIS2_PLACEMENT_3D('',#47914,#38642,#38643) ;
#31255=AXIS2_PLACEMENT_3D('',#47915,#38644,#38645) ;
#31256=AXIS2_PLACEMENT_3D('',#47916,#38646,#38647) ;
#31257=AXIS2_PLACEMENT_3D('',#47919,#38648,#38649) ;
#31258=AXIS2_PLACEMENT_3D('',#47921,#38650,#38651) ;
#31259=AXIS2_PLACEMENT_3D('',#47922,#38652,#38653) ;
#31260=AXIS2_PLACEMENT_3D('',#47923,#38654,#38655) ;
#31261=AXIS2_PLACEMENT_3D('',#47926,#38656,#38657) ;
#31262=AXIS2_PLACEMENT_3D('',#47928,#38658,#38659) ;
#31263=AXIS2_PLACEMENT_3D('',#47930,#38660,#38661) ;
#31264=AXIS2_PLACEMENT_3D('',#47932,#38662,#38663) ;
#31265=AXIS2_PLACEMENT_3D('',#47933,#38664,#38665) ;
#31266=AXIS2_PLACEMENT_3D('',#47934,#38666,#38667) ;
#31267=AXIS2_PLACEMENT_3D('',#47937,#38668,#38669) ;
#31268=AXIS2_PLACEMENT_3D('',#47939,#38670,#38671) ;
#31269=AXIS2_PLACEMENT_3D('',#47940,#38672,#38673) ;
#31270=AXIS2_PLACEMENT_3D('',#47941,#38674,#38675) ;
#31271=AXIS2_PLACEMENT_3D('',#47944,#38676,#38677) ;
#31272=AXIS2_PLACEMENT_3D('',#47946,#38678,#38679) ;
#31273=AXIS2_PLACEMENT_3D('',#47947,#38680,#38681) ;
#31274=AXIS2_PLACEMENT_3D('',#47948,#38682,#38683) ;
#31275=AXIS2_PLACEMENT_3D('',#47951,#38684,#38685) ;
#31276=AXIS2_PLACEMENT_3D('',#47953,#38686,#38687) ;
#31277=AXIS2_PLACEMENT_3D('',#47954,#38688,#38689) ;
#31278=AXIS2_PLACEMENT_3D('',#47955,#38690,#38691) ;
#31279=AXIS2_PLACEMENT_3D('',#47958,#38692,#38693) ;
#31280=AXIS2_PLACEMENT_3D('',#47960,#38694,#38695) ;
#31281=AXIS2_PLACEMENT_3D('',#47962,#38696,#38697) ;
#31282=AXIS2_PLACEMENT_3D('',#47964,#38698,#38699) ;
#31283=AXIS2_PLACEMENT_3D('',#47965,#38700,#38701) ;
#31284=AXIS2_PLACEMENT_3D('',#47966,#38702,#38703) ;
#31285=AXIS2_PLACEMENT_3D('',#47969,#38704,#38705) ;
#31286=AXIS2_PLACEMENT_3D('',#47971,#38706,#38707) ;
#31287=AXIS2_PLACEMENT_3D('',#47972,#38708,#38709) ;
#31288=AXIS2_PLACEMENT_3D('',#47973,#38710,#38711) ;
#31289=AXIS2_PLACEMENT_3D('',#47976,#38712,#38713) ;
#31290=AXIS2_PLACEMENT_3D('',#47978,#38714,#38715) ;
#31291=AXIS2_PLACEMENT_3D('',#47979,#38716,#38717) ;
#31292=AXIS2_PLACEMENT_3D('',#47980,#38718,#38719) ;
#31293=AXIS2_PLACEMENT_3D('',#47983,#38720,#38721) ;
#31294=AXIS2_PLACEMENT_3D('',#47985,#38722,#38723) ;
#31295=AXIS2_PLACEMENT_3D('',#47986,#38724,#38725) ;
#31296=AXIS2_PLACEMENT_3D('',#47987,#38726,#38727) ;
#31297=AXIS2_PLACEMENT_3D('',#47990,#38728,#38729) ;
#31298=AXIS2_PLACEMENT_3D('',#47992,#38730,#38731) ;
#31299=AXIS2_PLACEMENT_3D('',#47994,#38732,#38733) ;
#31300=AXIS2_PLACEMENT_3D('',#47996,#38734,#38735) ;
#31301=AXIS2_PLACEMENT_3D('',#47997,#38736,#38737) ;
#31302=AXIS2_PLACEMENT_3D('',#47998,#38738,#38739) ;
#31303=AXIS2_PLACEMENT_3D('',#48001,#38740,#38741) ;
#31304=AXIS2_PLACEMENT_3D('',#48003,#38742,#38743) ;
#31305=AXIS2_PLACEMENT_3D('',#48004,#38744,#38745) ;
#31306=AXIS2_PLACEMENT_3D('',#48005,#38746,#38747) ;
#31307=AXIS2_PLACEMENT_3D('',#48008,#38748,#38749) ;
#31308=AXIS2_PLACEMENT_3D('',#48010,#38750,#38751) ;
#31309=AXIS2_PLACEMENT_3D('',#48011,#38752,#38753) ;
#31310=AXIS2_PLACEMENT_3D('',#48012,#38754,#38755) ;
#31311=AXIS2_PLACEMENT_3D('',#48015,#38756,#38757) ;
#31312=AXIS2_PLACEMENT_3D('',#48017,#38758,#38759) ;
#31313=AXIS2_PLACEMENT_3D('',#48018,#38760,#38761) ;
#31314=AXIS2_PLACEMENT_3D('',#48019,#38762,#38763) ;
#31315=AXIS2_PLACEMENT_3D('',#48022,#38764,#38765) ;
#31316=AXIS2_PLACEMENT_3D('',#48024,#38766,#38767) ;
#31317=AXIS2_PLACEMENT_3D('',#48026,#38768,#38769) ;
#31318=AXIS2_PLACEMENT_3D('',#48028,#38770,#38771) ;
#31319=AXIS2_PLACEMENT_3D('',#48029,#38772,#38773) ;
#31320=AXIS2_PLACEMENT_3D('',#48030,#38774,#38775) ;
#31321=AXIS2_PLACEMENT_3D('',#48033,#38776,#38777) ;
#31322=AXIS2_PLACEMENT_3D('',#48035,#38778,#38779) ;
#31323=AXIS2_PLACEMENT_3D('',#48036,#38780,#38781) ;
#31324=AXIS2_PLACEMENT_3D('',#48037,#38782,#38783) ;
#31325=AXIS2_PLACEMENT_3D('',#48040,#38784,#38785) ;
#31326=AXIS2_PLACEMENT_3D('',#48042,#38786,#38787) ;
#31327=AXIS2_PLACEMENT_3D('',#48043,#38788,#38789) ;
#31328=AXIS2_PLACEMENT_3D('',#48044,#38790,#38791) ;
#31329=AXIS2_PLACEMENT_3D('',#48047,#38792,#38793) ;
#31330=AXIS2_PLACEMENT_3D('',#48049,#38794,#38795) ;
#31331=AXIS2_PLACEMENT_3D('',#48050,#38796,#38797) ;
#31332=AXIS2_PLACEMENT_3D('',#48051,#38798,#38799) ;
#31333=AXIS2_PLACEMENT_3D('',#48054,#38800,#38801) ;
#31334=AXIS2_PLACEMENT_3D('',#48056,#38802,#38803) ;
#31335=AXIS2_PLACEMENT_3D('',#48058,#38804,#38805) ;
#31336=AXIS2_PLACEMENT_3D('',#48060,#38806,#38807) ;
#31337=AXIS2_PLACEMENT_3D('',#48061,#38808,#38809) ;
#31338=AXIS2_PLACEMENT_3D('',#48062,#38810,#38811) ;
#31339=AXIS2_PLACEMENT_3D('',#48065,#38812,#38813) ;
#31340=AXIS2_PLACEMENT_3D('',#48067,#38814,#38815) ;
#31341=AXIS2_PLACEMENT_3D('',#48068,#38816,#38817) ;
#31342=AXIS2_PLACEMENT_3D('',#48069,#38818,#38819) ;
#31343=AXIS2_PLACEMENT_3D('',#48072,#38820,#38821) ;
#31344=AXIS2_PLACEMENT_3D('',#48074,#38822,#38823) ;
#31345=AXIS2_PLACEMENT_3D('',#48075,#38824,#38825) ;
#31346=AXIS2_PLACEMENT_3D('',#48076,#38826,#38827) ;
#31347=AXIS2_PLACEMENT_3D('',#48079,#38828,#38829) ;
#31348=AXIS2_PLACEMENT_3D('',#48081,#38830,#38831) ;
#31349=AXIS2_PLACEMENT_3D('',#48082,#38832,#38833) ;
#31350=AXIS2_PLACEMENT_3D('',#48083,#38834,#38835) ;
#31351=AXIS2_PLACEMENT_3D('',#48086,#38836,#38837) ;
#31352=AXIS2_PLACEMENT_3D('',#48088,#38838,#38839) ;
#31353=AXIS2_PLACEMENT_3D('',#48090,#38840,#38841) ;
#31354=AXIS2_PLACEMENT_3D('',#48092,#38842,#38843) ;
#31355=AXIS2_PLACEMENT_3D('',#48093,#38844,#38845) ;
#31356=AXIS2_PLACEMENT_3D('',#48094,#38846,#38847) ;
#31357=AXIS2_PLACEMENT_3D('',#48097,#38848,#38849) ;
#31358=AXIS2_PLACEMENT_3D('',#48099,#38850,#38851) ;
#31359=AXIS2_PLACEMENT_3D('',#48100,#38852,#38853) ;
#31360=AXIS2_PLACEMENT_3D('',#48101,#38854,#38855) ;
#31361=AXIS2_PLACEMENT_3D('',#48104,#38856,#38857) ;
#31362=AXIS2_PLACEMENT_3D('',#48106,#38858,#38859) ;
#31363=AXIS2_PLACEMENT_3D('',#48107,#38860,#38861) ;
#31364=AXIS2_PLACEMENT_3D('',#48108,#38862,#38863) ;
#31365=AXIS2_PLACEMENT_3D('',#48111,#38864,#38865) ;
#31366=AXIS2_PLACEMENT_3D('',#48113,#38866,#38867) ;
#31367=AXIS2_PLACEMENT_3D('',#48114,#38868,#38869) ;
#31368=AXIS2_PLACEMENT_3D('',#48115,#38870,#38871) ;
#31369=AXIS2_PLACEMENT_3D('',#48118,#38872,#38873) ;
#31370=AXIS2_PLACEMENT_3D('',#48120,#38874,#38875) ;
#31371=AXIS2_PLACEMENT_3D('',#48122,#38876,#38877) ;
#31372=AXIS2_PLACEMENT_3D('',#48124,#38878,#38879) ;
#31373=AXIS2_PLACEMENT_3D('',#48125,#38880,#38881) ;
#31374=AXIS2_PLACEMENT_3D('',#48126,#38882,#38883) ;
#31375=AXIS2_PLACEMENT_3D('',#48129,#38884,#38885) ;
#31376=AXIS2_PLACEMENT_3D('',#48131,#38886,#38887) ;
#31377=AXIS2_PLACEMENT_3D('',#48132,#38888,#38889) ;
#31378=AXIS2_PLACEMENT_3D('',#48133,#38890,#38891) ;
#31379=AXIS2_PLACEMENT_3D('',#48136,#38892,#38893) ;
#31380=AXIS2_PLACEMENT_3D('',#48138,#38894,#38895) ;
#31381=AXIS2_PLACEMENT_3D('',#48139,#38896,#38897) ;
#31382=AXIS2_PLACEMENT_3D('',#48140,#38898,#38899) ;
#31383=AXIS2_PLACEMENT_3D('',#48143,#38900,#38901) ;
#31384=AXIS2_PLACEMENT_3D('',#48145,#38902,#38903) ;
#31385=AXIS2_PLACEMENT_3D('',#48146,#38904,#38905) ;
#31386=AXIS2_PLACEMENT_3D('',#48147,#38906,#38907) ;
#31387=AXIS2_PLACEMENT_3D('',#48150,#38908,#38909) ;
#31388=AXIS2_PLACEMENT_3D('',#48152,#38910,#38911) ;
#31389=AXIS2_PLACEMENT_3D('',#48154,#38912,#38913) ;
#31390=AXIS2_PLACEMENT_3D('',#48156,#38914,#38915) ;
#31391=AXIS2_PLACEMENT_3D('',#48157,#38916,#38917) ;
#31392=AXIS2_PLACEMENT_3D('',#48158,#38918,#38919) ;
#31393=AXIS2_PLACEMENT_3D('',#48161,#38920,#38921) ;
#31394=AXIS2_PLACEMENT_3D('',#48163,#38922,#38923) ;
#31395=AXIS2_PLACEMENT_3D('',#48164,#38924,#38925) ;
#31396=AXIS2_PLACEMENT_3D('',#48165,#38926,#38927) ;
#31397=AXIS2_PLACEMENT_3D('',#48168,#38928,#38929) ;
#31398=AXIS2_PLACEMENT_3D('',#48170,#38930,#38931) ;
#31399=AXIS2_PLACEMENT_3D('',#48171,#38932,#38933) ;
#31400=AXIS2_PLACEMENT_3D('',#48172,#38934,#38935) ;
#31401=AXIS2_PLACEMENT_3D('',#48175,#38936,#38937) ;
#31402=AXIS2_PLACEMENT_3D('',#48177,#38938,#38939) ;
#31403=AXIS2_PLACEMENT_3D('',#48178,#38940,#38941) ;
#31404=AXIS2_PLACEMENT_3D('',#48179,#38942,#38943) ;
#31405=AXIS2_PLACEMENT_3D('',#48182,#38944,#38945) ;
#31406=AXIS2_PLACEMENT_3D('',#48184,#38946,#38947) ;
#31407=AXIS2_PLACEMENT_3D('',#48186,#38948,#38949) ;
#31408=AXIS2_PLACEMENT_3D('',#48188,#38950,#38951) ;
#31409=AXIS2_PLACEMENT_3D('',#48189,#38952,#38953) ;
#31410=AXIS2_PLACEMENT_3D('',#48190,#38954,#38955) ;
#31411=AXIS2_PLACEMENT_3D('',#48193,#38956,#38957) ;
#31412=AXIS2_PLACEMENT_3D('',#48195,#38958,#38959) ;
#31413=AXIS2_PLACEMENT_3D('',#48196,#38960,#38961) ;
#31414=AXIS2_PLACEMENT_3D('',#48197,#38962,#38963) ;
#31415=AXIS2_PLACEMENT_3D('',#48200,#38964,#38965) ;
#31416=AXIS2_PLACEMENT_3D('',#48202,#38966,#38967) ;
#31417=AXIS2_PLACEMENT_3D('',#48203,#38968,#38969) ;
#31418=AXIS2_PLACEMENT_3D('',#48204,#38970,#38971) ;
#31419=AXIS2_PLACEMENT_3D('',#48207,#38972,#38973) ;
#31420=AXIS2_PLACEMENT_3D('',#48209,#38974,#38975) ;
#31421=AXIS2_PLACEMENT_3D('',#48210,#38976,#38977) ;
#31422=AXIS2_PLACEMENT_3D('',#48211,#38978,#38979) ;
#31423=AXIS2_PLACEMENT_3D('',#48214,#38980,#38981) ;
#31424=AXIS2_PLACEMENT_3D('',#48216,#38982,#38983) ;
#31425=AXIS2_PLACEMENT_3D('',#48218,#38984,#38985) ;
#31426=AXIS2_PLACEMENT_3D('',#48220,#38986,#38987) ;
#31427=AXIS2_PLACEMENT_3D('',#48221,#38988,#38989) ;
#31428=AXIS2_PLACEMENT_3D('',#48222,#38990,#38991) ;
#31429=AXIS2_PLACEMENT_3D('',#48225,#38992,#38993) ;
#31430=AXIS2_PLACEMENT_3D('',#48227,#38994,#38995) ;
#31431=AXIS2_PLACEMENT_3D('',#48228,#38996,#38997) ;
#31432=AXIS2_PLACEMENT_3D('',#48229,#38998,#38999) ;
#31433=AXIS2_PLACEMENT_3D('',#48232,#39000,#39001) ;
#31434=AXIS2_PLACEMENT_3D('',#48234,#39002,#39003) ;
#31435=AXIS2_PLACEMENT_3D('',#48235,#39004,#39005) ;
#31436=AXIS2_PLACEMENT_3D('',#48236,#39006,#39007) ;
#31437=AXIS2_PLACEMENT_3D('',#48239,#39008,#39009) ;
#31438=AXIS2_PLACEMENT_3D('',#48241,#39010,#39011) ;
#31439=AXIS2_PLACEMENT_3D('',#48242,#39012,#39013) ;
#31440=AXIS2_PLACEMENT_3D('',#48243,#39014,#39015) ;
#31441=AXIS2_PLACEMENT_3D('',#48246,#39016,#39017) ;
#31442=AXIS2_PLACEMENT_3D('',#48248,#39018,#39019) ;
#31443=AXIS2_PLACEMENT_3D('',#48250,#39020,#39021) ;
#31444=AXIS2_PLACEMENT_3D('',#48252,#39022,#39023) ;
#31445=AXIS2_PLACEMENT_3D('',#48253,#39024,#39025) ;
#31446=AXIS2_PLACEMENT_3D('',#48254,#39026,#39027) ;
#31447=AXIS2_PLACEMENT_3D('',#48257,#39028,#39029) ;
#31448=AXIS2_PLACEMENT_3D('',#48259,#39030,#39031) ;
#31449=AXIS2_PLACEMENT_3D('',#48260,#39032,#39033) ;
#31450=AXIS2_PLACEMENT_3D('',#48261,#39034,#39035) ;
#31451=AXIS2_PLACEMENT_3D('',#48264,#39036,#39037) ;
#31452=AXIS2_PLACEMENT_3D('',#48266,#39038,#39039) ;
#31453=AXIS2_PLACEMENT_3D('',#48267,#39040,#39041) ;
#31454=AXIS2_PLACEMENT_3D('',#48268,#39042,#39043) ;
#31455=AXIS2_PLACEMENT_3D('',#48271,#39044,#39045) ;
#31456=AXIS2_PLACEMENT_3D('',#48273,#39046,#39047) ;
#31457=AXIS2_PLACEMENT_3D('',#48274,#39048,#39049) ;
#31458=AXIS2_PLACEMENT_3D('',#48275,#39050,#39051) ;
#31459=AXIS2_PLACEMENT_3D('',#48278,#39052,#39053) ;
#31460=AXIS2_PLACEMENT_3D('',#48280,#39054,#39055) ;
#31461=AXIS2_PLACEMENT_3D('',#48282,#39056,#39057) ;
#31462=AXIS2_PLACEMENT_3D('',#48284,#39058,#39059) ;
#31463=AXIS2_PLACEMENT_3D('',#48285,#39060,#39061) ;
#31464=AXIS2_PLACEMENT_3D('',#48286,#39062,#39063) ;
#31465=AXIS2_PLACEMENT_3D('',#48289,#39064,#39065) ;
#31466=AXIS2_PLACEMENT_3D('',#48291,#39066,#39067) ;
#31467=AXIS2_PLACEMENT_3D('',#48292,#39068,#39069) ;
#31468=AXIS2_PLACEMENT_3D('',#48293,#39070,#39071) ;
#31469=AXIS2_PLACEMENT_3D('',#48296,#39072,#39073) ;
#31470=AXIS2_PLACEMENT_3D('',#48298,#39074,#39075) ;
#31471=AXIS2_PLACEMENT_3D('',#48299,#39076,#39077) ;
#31472=AXIS2_PLACEMENT_3D('',#48300,#39078,#39079) ;
#31473=AXIS2_PLACEMENT_3D('',#48303,#39080,#39081) ;
#31474=AXIS2_PLACEMENT_3D('',#48305,#39082,#39083) ;
#31475=AXIS2_PLACEMENT_3D('',#48306,#39084,#39085) ;
#31476=AXIS2_PLACEMENT_3D('',#48307,#39086,#39087) ;
#31477=AXIS2_PLACEMENT_3D('',#48310,#39088,#39089) ;
#31478=AXIS2_PLACEMENT_3D('',#48312,#39090,#39091) ;
#31479=AXIS2_PLACEMENT_3D('',#48314,#39092,#39093) ;
#31480=AXIS2_PLACEMENT_3D('',#48316,#39094,#39095) ;
#31481=AXIS2_PLACEMENT_3D('',#48317,#39096,#39097) ;
#31482=AXIS2_PLACEMENT_3D('',#48318,#39098,#39099) ;
#31483=AXIS2_PLACEMENT_3D('',#48321,#39100,#39101) ;
#31484=AXIS2_PLACEMENT_3D('',#48323,#39102,#39103) ;
#31485=AXIS2_PLACEMENT_3D('',#48324,#39104,#39105) ;
#31486=AXIS2_PLACEMENT_3D('',#48325,#39106,#39107) ;
#31487=AXIS2_PLACEMENT_3D('',#48328,#39108,#39109) ;
#31488=AXIS2_PLACEMENT_3D('',#48330,#39110,#39111) ;
#31489=AXIS2_PLACEMENT_3D('',#48331,#39112,#39113) ;
#31490=AXIS2_PLACEMENT_3D('',#48332,#39114,#39115) ;
#31491=AXIS2_PLACEMENT_3D('',#48335,#39116,#39117) ;
#31492=AXIS2_PLACEMENT_3D('',#48337,#39118,#39119) ;
#31493=AXIS2_PLACEMENT_3D('',#48338,#39120,#39121) ;
#31494=AXIS2_PLACEMENT_3D('',#48339,#39122,#39123) ;
#31495=AXIS2_PLACEMENT_3D('',#48342,#39124,#39125) ;
#31496=AXIS2_PLACEMENT_3D('',#48344,#39126,#39127) ;
#31497=AXIS2_PLACEMENT_3D('',#48346,#39128,#39129) ;
#31498=AXIS2_PLACEMENT_3D('',#48348,#39130,#39131) ;
#31499=AXIS2_PLACEMENT_3D('',#48349,#39132,#39133) ;
#31500=AXIS2_PLACEMENT_3D('',#48350,#39134,#39135) ;
#31501=AXIS2_PLACEMENT_3D('',#48353,#39136,#39137) ;
#31502=AXIS2_PLACEMENT_3D('',#48355,#39138,#39139) ;
#31503=AXIS2_PLACEMENT_3D('',#48356,#39140,#39141) ;
#31504=AXIS2_PLACEMENT_3D('',#48357,#39142,#39143) ;
#31505=AXIS2_PLACEMENT_3D('',#48360,#39144,#39145) ;
#31506=AXIS2_PLACEMENT_3D('',#48362,#39146,#39147) ;
#31507=AXIS2_PLACEMENT_3D('',#48363,#39148,#39149) ;
#31508=AXIS2_PLACEMENT_3D('',#48364,#39150,#39151) ;
#31509=AXIS2_PLACEMENT_3D('',#48367,#39152,#39153) ;
#31510=AXIS2_PLACEMENT_3D('',#48369,#39154,#39155) ;
#31511=AXIS2_PLACEMENT_3D('',#48370,#39156,#39157) ;
#31512=AXIS2_PLACEMENT_3D('',#48371,#39158,#39159) ;
#31513=AXIS2_PLACEMENT_3D('',#48374,#39160,#39161) ;
#31514=AXIS2_PLACEMENT_3D('',#48376,#39162,#39163) ;
#31515=AXIS2_PLACEMENT_3D('',#48378,#39164,#39165) ;
#31516=AXIS2_PLACEMENT_3D('',#48380,#39166,#39167) ;
#31517=AXIS2_PLACEMENT_3D('',#48381,#39168,#39169) ;
#31518=AXIS2_PLACEMENT_3D('',#48382,#39170,#39171) ;
#31519=AXIS2_PLACEMENT_3D('',#48385,#39172,#39173) ;
#31520=AXIS2_PLACEMENT_3D('',#48387,#39174,#39175) ;
#31521=AXIS2_PLACEMENT_3D('',#48388,#39176,#39177) ;
#31522=AXIS2_PLACEMENT_3D('',#48389,#39178,#39179) ;
#31523=AXIS2_PLACEMENT_3D('',#48392,#39180,#39181) ;
#31524=AXIS2_PLACEMENT_3D('',#48394,#39182,#39183) ;
#31525=AXIS2_PLACEMENT_3D('',#48395,#39184,#39185) ;
#31526=AXIS2_PLACEMENT_3D('',#48396,#39186,#39187) ;
#31527=AXIS2_PLACEMENT_3D('',#48399,#39188,#39189) ;
#31528=AXIS2_PLACEMENT_3D('',#48401,#39190,#39191) ;
#31529=AXIS2_PLACEMENT_3D('',#48402,#39192,#39193) ;
#31530=AXIS2_PLACEMENT_3D('',#48403,#39194,#39195) ;
#31531=AXIS2_PLACEMENT_3D('',#48406,#39196,#39197) ;
#31532=AXIS2_PLACEMENT_3D('',#48408,#39198,#39199) ;
#31533=AXIS2_PLACEMENT_3D('',#48410,#39200,#39201) ;
#31534=AXIS2_PLACEMENT_3D('',#48412,#39202,#39203) ;
#31535=AXIS2_PLACEMENT_3D('',#48413,#39204,#39205) ;
#31536=AXIS2_PLACEMENT_3D('',#48414,#39206,#39207) ;
#31537=AXIS2_PLACEMENT_3D('',#48417,#39208,#39209) ;
#31538=AXIS2_PLACEMENT_3D('',#48419,#39210,#39211) ;
#31539=AXIS2_PLACEMENT_3D('',#48420,#39212,#39213) ;
#31540=AXIS2_PLACEMENT_3D('',#48421,#39214,#39215) ;
#31541=AXIS2_PLACEMENT_3D('',#48424,#39216,#39217) ;
#31542=AXIS2_PLACEMENT_3D('',#48426,#39218,#39219) ;
#31543=AXIS2_PLACEMENT_3D('',#48427,#39220,#39221) ;
#31544=AXIS2_PLACEMENT_3D('',#48428,#39222,#39223) ;
#31545=AXIS2_PLACEMENT_3D('',#48431,#39224,#39225) ;
#31546=AXIS2_PLACEMENT_3D('',#48433,#39226,#39227) ;
#31547=AXIS2_PLACEMENT_3D('',#48434,#39228,#39229) ;
#31548=AXIS2_PLACEMENT_3D('',#48435,#39230,#39231) ;
#31549=AXIS2_PLACEMENT_3D('',#48438,#39232,#39233) ;
#31550=AXIS2_PLACEMENT_3D('',#48440,#39234,#39235) ;
#31551=AXIS2_PLACEMENT_3D('',#48442,#39236,#39237) ;
#31552=AXIS2_PLACEMENT_3D('',#48444,#39238,#39239) ;
#31553=AXIS2_PLACEMENT_3D('',#48445,#39240,#39241) ;
#31554=AXIS2_PLACEMENT_3D('',#48446,#39242,#39243) ;
#31555=AXIS2_PLACEMENT_3D('',#48449,#39244,#39245) ;
#31556=AXIS2_PLACEMENT_3D('',#48451,#39246,#39247) ;
#31557=AXIS2_PLACEMENT_3D('',#48452,#39248,#39249) ;
#31558=AXIS2_PLACEMENT_3D('',#48453,#39250,#39251) ;
#31559=AXIS2_PLACEMENT_3D('',#48456,#39252,#39253) ;
#31560=AXIS2_PLACEMENT_3D('',#48458,#39254,#39255) ;
#31561=AXIS2_PLACEMENT_3D('',#48459,#39256,#39257) ;
#31562=AXIS2_PLACEMENT_3D('',#48460,#39258,#39259) ;
#31563=AXIS2_PLACEMENT_3D('',#48463,#39260,#39261) ;
#31564=AXIS2_PLACEMENT_3D('',#48465,#39262,#39263) ;
#31565=AXIS2_PLACEMENT_3D('',#48466,#39264,#39265) ;
#31566=AXIS2_PLACEMENT_3D('',#48467,#39266,#39267) ;
#31567=AXIS2_PLACEMENT_3D('',#48470,#39268,#39269) ;
#31568=AXIS2_PLACEMENT_3D('',#48472,#39270,#39271) ;
#31569=AXIS2_PLACEMENT_3D('',#48474,#39272,#39273) ;
#31570=AXIS2_PLACEMENT_3D('',#48476,#39274,#39275) ;
#31571=AXIS2_PLACEMENT_3D('',#48477,#39276,#39277) ;
#31572=AXIS2_PLACEMENT_3D('',#48478,#39278,#39279) ;
#31573=AXIS2_PLACEMENT_3D('',#48481,#39280,#39281) ;
#31574=AXIS2_PLACEMENT_3D('',#48483,#39282,#39283) ;
#31575=AXIS2_PLACEMENT_3D('',#48484,#39284,#39285) ;
#31576=AXIS2_PLACEMENT_3D('',#48485,#39286,#39287) ;
#31577=AXIS2_PLACEMENT_3D('',#48488,#39288,#39289) ;
#31578=AXIS2_PLACEMENT_3D('',#48490,#39290,#39291) ;
#31579=AXIS2_PLACEMENT_3D('',#48491,#39292,#39293) ;
#31580=AXIS2_PLACEMENT_3D('',#48492,#39294,#39295) ;
#31581=AXIS2_PLACEMENT_3D('',#48495,#39296,#39297) ;
#31582=AXIS2_PLACEMENT_3D('',#48497,#39298,#39299) ;
#31583=AXIS2_PLACEMENT_3D('',#48498,#39300,#39301) ;
#31584=AXIS2_PLACEMENT_3D('',#48499,#39302,#39303) ;
#31585=AXIS2_PLACEMENT_3D('',#48502,#39304,#39305) ;
#31586=AXIS2_PLACEMENT_3D('',#48504,#39306,#39307) ;
#31587=AXIS2_PLACEMENT_3D('',#48506,#39308,#39309) ;
#31588=AXIS2_PLACEMENT_3D('',#48508,#39310,#39311) ;
#31589=AXIS2_PLACEMENT_3D('',#48509,#39312,#39313) ;
#31590=AXIS2_PLACEMENT_3D('',#48510,#39314,#39315) ;
#31591=AXIS2_PLACEMENT_3D('',#48513,#39316,#39317) ;
#31592=AXIS2_PLACEMENT_3D('',#48515,#39318,#39319) ;
#31593=AXIS2_PLACEMENT_3D('',#48516,#39320,#39321) ;
#31594=AXIS2_PLACEMENT_3D('',#48517,#39322,#39323) ;
#31595=AXIS2_PLACEMENT_3D('',#48520,#39324,#39325) ;
#31596=AXIS2_PLACEMENT_3D('',#48522,#39326,#39327) ;
#31597=AXIS2_PLACEMENT_3D('',#48523,#39328,#39329) ;
#31598=AXIS2_PLACEMENT_3D('',#48524,#39330,#39331) ;
#31599=AXIS2_PLACEMENT_3D('',#48527,#39332,#39333) ;
#31600=AXIS2_PLACEMENT_3D('',#48529,#39334,#39335) ;
#31601=AXIS2_PLACEMENT_3D('',#48530,#39336,#39337) ;
#31602=AXIS2_PLACEMENT_3D('',#48531,#39338,#39339) ;
#31603=AXIS2_PLACEMENT_3D('',#48534,#39340,#39341) ;
#31604=AXIS2_PLACEMENT_3D('',#48536,#39342,#39343) ;
#31605=AXIS2_PLACEMENT_3D('',#48538,#39344,#39345) ;
#31606=AXIS2_PLACEMENT_3D('',#48540,#39346,#39347) ;
#31607=AXIS2_PLACEMENT_3D('',#48541,#39348,#39349) ;
#31608=AXIS2_PLACEMENT_3D('',#48542,#39350,#39351) ;
#31609=AXIS2_PLACEMENT_3D('',#48545,#39352,#39353) ;
#31610=AXIS2_PLACEMENT_3D('',#48547,#39354,#39355) ;
#31611=AXIS2_PLACEMENT_3D('',#48548,#39356,#39357) ;
#31612=AXIS2_PLACEMENT_3D('',#48549,#39358,#39359) ;
#31613=AXIS2_PLACEMENT_3D('',#48552,#39360,#39361) ;
#31614=AXIS2_PLACEMENT_3D('',#48554,#39362,#39363) ;
#31615=AXIS2_PLACEMENT_3D('',#48555,#39364,#39365) ;
#31616=AXIS2_PLACEMENT_3D('',#48556,#39366,#39367) ;
#31617=AXIS2_PLACEMENT_3D('',#48559,#39368,#39369) ;
#31618=AXIS2_PLACEMENT_3D('',#48561,#39370,#39371) ;
#31619=AXIS2_PLACEMENT_3D('',#48562,#39372,#39373) ;
#31620=AXIS2_PLACEMENT_3D('',#48563,#39374,#39375) ;
#31621=AXIS2_PLACEMENT_3D('',#48566,#39376,#39377) ;
#31622=AXIS2_PLACEMENT_3D('',#48568,#39378,#39379) ;
#31623=AXIS2_PLACEMENT_3D('',#48570,#39380,#39381) ;
#31624=AXIS2_PLACEMENT_3D('',#48572,#39382,#39383) ;
#31625=AXIS2_PLACEMENT_3D('',#48573,#39384,#39385) ;
#31626=AXIS2_PLACEMENT_3D('',#48574,#39386,#39387) ;
#31627=AXIS2_PLACEMENT_3D('',#48577,#39388,#39389) ;
#31628=AXIS2_PLACEMENT_3D('',#48579,#39390,#39391) ;
#31629=AXIS2_PLACEMENT_3D('',#48580,#39392,#39393) ;
#31630=AXIS2_PLACEMENT_3D('',#48581,#39394,#39395) ;
#31631=AXIS2_PLACEMENT_3D('',#48584,#39396,#39397) ;
#31632=AXIS2_PLACEMENT_3D('',#48586,#39398,#39399) ;
#31633=AXIS2_PLACEMENT_3D('',#48587,#39400,#39401) ;
#31634=AXIS2_PLACEMENT_3D('',#48588,#39402,#39403) ;
#31635=AXIS2_PLACEMENT_3D('',#48591,#39404,#39405) ;
#31636=AXIS2_PLACEMENT_3D('',#48593,#39406,#39407) ;
#31637=AXIS2_PLACEMENT_3D('',#48594,#39408,#39409) ;
#31638=AXIS2_PLACEMENT_3D('',#48595,#39410,#39411) ;
#31639=AXIS2_PLACEMENT_3D('',#48598,#39412,#39413) ;
#31640=AXIS2_PLACEMENT_3D('',#48600,#39414,#39415) ;
#31641=AXIS2_PLACEMENT_3D('',#48602,#39416,#39417) ;
#31642=AXIS2_PLACEMENT_3D('',#48604,#39418,#39419) ;
#31643=AXIS2_PLACEMENT_3D('',#48605,#39420,#39421) ;
#31644=AXIS2_PLACEMENT_3D('',#48606,#39422,#39423) ;
#31645=AXIS2_PLACEMENT_3D('',#48609,#39424,#39425) ;
#31646=AXIS2_PLACEMENT_3D('',#48611,#39426,#39427) ;
#31647=AXIS2_PLACEMENT_3D('',#48612,#39428,#39429) ;
#31648=AXIS2_PLACEMENT_3D('',#48613,#39430,#39431) ;
#31649=AXIS2_PLACEMENT_3D('',#48616,#39432,#39433) ;
#31650=AXIS2_PLACEMENT_3D('',#48618,#39434,#39435) ;
#31651=AXIS2_PLACEMENT_3D('',#48619,#39436,#39437) ;
#31652=AXIS2_PLACEMENT_3D('',#48620,#39438,#39439) ;
#31653=AXIS2_PLACEMENT_3D('',#48623,#39440,#39441) ;
#31654=AXIS2_PLACEMENT_3D('',#48625,#39442,#39443) ;
#31655=AXIS2_PLACEMENT_3D('',#48626,#39444,#39445) ;
#31656=AXIS2_PLACEMENT_3D('',#48627,#39446,#39447) ;
#31657=AXIS2_PLACEMENT_3D('',#48630,#39448,#39449) ;
#31658=AXIS2_PLACEMENT_3D('',#48632,#39450,#39451) ;
#31659=AXIS2_PLACEMENT_3D('',#48634,#39452,#39453) ;
#31660=AXIS2_PLACEMENT_3D('',#48636,#39454,#39455) ;
#31661=AXIS2_PLACEMENT_3D('',#48637,#39456,#39457) ;
#31662=AXIS2_PLACEMENT_3D('',#48638,#39458,#39459) ;
#31663=AXIS2_PLACEMENT_3D('',#48641,#39460,#39461) ;
#31664=AXIS2_PLACEMENT_3D('',#48643,#39462,#39463) ;
#31665=AXIS2_PLACEMENT_3D('',#48644,#39464,#39465) ;
#31666=AXIS2_PLACEMENT_3D('',#48645,#39466,#39467) ;
#31667=AXIS2_PLACEMENT_3D('',#48648,#39468,#39469) ;
#31668=AXIS2_PLACEMENT_3D('',#48650,#39470,#39471) ;
#31669=AXIS2_PLACEMENT_3D('',#48651,#39472,#39473) ;
#31670=AXIS2_PLACEMENT_3D('',#48652,#39474,#39475) ;
#31671=AXIS2_PLACEMENT_3D('',#48655,#39476,#39477) ;
#31672=AXIS2_PLACEMENT_3D('',#48657,#39478,#39479) ;
#31673=AXIS2_PLACEMENT_3D('',#48658,#39480,#39481) ;
#31674=AXIS2_PLACEMENT_3D('',#48659,#39482,#39483) ;
#31675=AXIS2_PLACEMENT_3D('',#48660,#39484,#39485) ;
#31676=AXIS2_PLACEMENT_3D('',#48661,#39486,#39487) ;
#31677=AXIS2_PLACEMENT_3D('',#48662,#39488,#39489) ;
#31678=AXIS2_PLACEMENT_3D('',#48663,#39490,#39491) ;
#31679=AXIS2_PLACEMENT_3D('',#48666,#39493,#39494) ;
#31680=AXIS2_PLACEMENT_3D('',#48667,#39495,#39496) ;
#31681=AXIS2_PLACEMENT_3D('',#48668,#39497,#39498) ;
#31682=AXIS2_PLACEMENT_3D('',#48671,#39500,#39501) ;
#31683=AXIS2_PLACEMENT_3D('',#48672,#39502,#39503) ;
#31684=AXIS2_PLACEMENT_3D('',#48673,#39504,#39505) ;
#31685=AXIS2_PLACEMENT_3D('',#48676,#39507,#39508) ;
#31686=AXIS2_PLACEMENT_3D('',#48677,#39509,#39510) ;
#31687=AXIS2_PLACEMENT_3D('',#48678,#39511,#39512) ;
#31688=AXIS2_PLACEMENT_3D('',#48681,#39514,#39515) ;
#31689=AXIS2_PLACEMENT_3D('',#48682,#39516,#39517) ;
#31690=AXIS2_PLACEMENT_3D('',#48683,#39518,#39519) ;
#31691=AXIS2_PLACEMENT_3D('',#48686,#39521,#39522) ;
#31692=AXIS2_PLACEMENT_3D('',#48687,#39523,#39524) ;
#31693=AXIS2_PLACEMENT_3D('',#48688,#39525,#39526) ;
#31694=AXIS2_PLACEMENT_3D('',#48691,#39528,#39529) ;
#31695=AXIS2_PLACEMENT_3D('',#48692,#39530,#39531) ;
#31696=AXIS2_PLACEMENT_3D('',#48693,#39532,#39533) ;
#31697=AXIS2_PLACEMENT_3D('',#48696,#39535,#39536) ;
#31698=AXIS2_PLACEMENT_3D('',#48697,#39537,#39538) ;
#31699=AXIS2_PLACEMENT_3D('',#48698,#39539,#39540) ;
#31700=AXIS2_PLACEMENT_3D('',#48701,#39542,#39543) ;
#31701=AXIS2_PLACEMENT_3D('',#48702,#39544,#39545) ;
#31702=AXIS2_PLACEMENT_3D('',#48703,#39546,#39547) ;
#31703=AXIS2_PLACEMENT_3D('',#48706,#39549,#39550) ;
#31704=AXIS2_PLACEMENT_3D('',#48707,#39551,#39552) ;
#31705=AXIS2_PLACEMENT_3D('',#48708,#39553,#39554) ;
#31706=AXIS2_PLACEMENT_3D('',#48711,#39556,#39557) ;
#31707=AXIS2_PLACEMENT_3D('',#48712,#39558,#39559) ;
#31708=AXIS2_PLACEMENT_3D('',#48713,#39560,#39561) ;
#31709=AXIS2_PLACEMENT_3D('',#48716,#39563,#39564) ;
#31710=AXIS2_PLACEMENT_3D('',#48717,#39565,#39566) ;
#31711=AXIS2_PLACEMENT_3D('',#48718,#39567,#39568) ;
#31712=AXIS2_PLACEMENT_3D('',#48721,#39570,#39571) ;
#31713=AXIS2_PLACEMENT_3D('',#48722,#39572,#39573) ;
#31714=AXIS2_PLACEMENT_3D('',#48723,#39574,#39575) ;
#31715=AXIS2_PLACEMENT_3D('',#48726,#39577,#39578) ;
#31716=AXIS2_PLACEMENT_3D('',#48727,#39579,#39580) ;
#31717=AXIS2_PLACEMENT_3D('',#48728,#39581,#39582) ;
#31718=AXIS2_PLACEMENT_3D('',#48731,#39584,#39585) ;
#31719=AXIS2_PLACEMENT_3D('',#48732,#39586,#39587) ;
#31720=AXIS2_PLACEMENT_3D('',#48733,#39588,#39589) ;
#31721=AXIS2_PLACEMENT_3D('',#48736,#39591,#39592) ;
#31722=AXIS2_PLACEMENT_3D('',#48737,#39593,#39594) ;
#31723=AXIS2_PLACEMENT_3D('',#48738,#39595,#39596) ;
#31724=AXIS2_PLACEMENT_3D('',#48741,#39598,#39599) ;
#31725=AXIS2_PLACEMENT_3D('',#48742,#39600,#39601) ;
#31726=AXIS2_PLACEMENT_3D('',#48743,#39602,#39603) ;
#31727=AXIS2_PLACEMENT_3D('',#48746,#39605,#39606) ;
#31728=AXIS2_PLACEMENT_3D('',#48747,#39607,#39608) ;
#31729=AXIS2_PLACEMENT_3D('',#48748,#39609,#39610) ;
#31730=AXIS2_PLACEMENT_3D('',#48751,#39612,#39613) ;
#31731=AXIS2_PLACEMENT_3D('',#48752,#39614,#39615) ;
#31732=AXIS2_PLACEMENT_3D('',#48753,#39616,#39617) ;
#31733=AXIS2_PLACEMENT_3D('',#48756,#39619,#39620) ;
#31734=AXIS2_PLACEMENT_3D('',#48757,#39621,#39622) ;
#31735=AXIS2_PLACEMENT_3D('',#48758,#39623,#39624) ;
#31736=AXIS2_PLACEMENT_3D('',#48761,#39626,#39627) ;
#31737=AXIS2_PLACEMENT_3D('',#48762,#39628,#39629) ;
#31738=AXIS2_PLACEMENT_3D('',#48763,#39630,#39631) ;
#31739=AXIS2_PLACEMENT_3D('',#48766,#39633,#39634) ;
#31740=AXIS2_PLACEMENT_3D('',#48767,#39635,#39636) ;
#31741=AXIS2_PLACEMENT_3D('',#48768,#39637,#39638) ;
#31742=AXIS2_PLACEMENT_3D('',#48771,#39640,#39641) ;
#31743=AXIS2_PLACEMENT_3D('',#48772,#39642,#39643) ;
#31744=AXIS2_PLACEMENT_3D('',#48773,#39644,#39645) ;
#31745=AXIS2_PLACEMENT_3D('',#48776,#39647,#39648) ;
#31746=AXIS2_PLACEMENT_3D('',#48777,#39649,#39650) ;
#31747=AXIS2_PLACEMENT_3D('',#48778,#39651,#39652) ;
#31748=AXIS2_PLACEMENT_3D('',#48781,#39654,#39655) ;
#31749=AXIS2_PLACEMENT_3D('',#48782,#39656,#39657) ;
#31750=AXIS2_PLACEMENT_3D('',#48783,#39658,#39659) ;
#31751=AXIS2_PLACEMENT_3D('',#48786,#39661,#39662) ;
#31752=AXIS2_PLACEMENT_3D('',#48787,#39663,#39664) ;
#31753=AXIS2_PLACEMENT_3D('',#48788,#39665,#39666) ;
#31754=AXIS2_PLACEMENT_3D('',#48791,#39668,#39669) ;
#31755=AXIS2_PLACEMENT_3D('',#48792,#39670,#39671) ;
#31756=AXIS2_PLACEMENT_3D('',#48793,#39672,#39673) ;
#31757=AXIS2_PLACEMENT_3D('',#48796,#39675,#39676) ;
#31758=AXIS2_PLACEMENT_3D('',#48797,#39677,#39678) ;
#31759=AXIS2_PLACEMENT_3D('',#48798,#39679,#39680) ;
#31760=AXIS2_PLACEMENT_3D('',#48801,#39682,#39683) ;
#31761=AXIS2_PLACEMENT_3D('',#48802,#39684,#39685) ;
#31762=AXIS2_PLACEMENT_3D('',#48803,#39686,#39687) ;
#31763=AXIS2_PLACEMENT_3D('',#48806,#39689,#39690) ;
#31764=AXIS2_PLACEMENT_3D('',#48807,#39691,#39692) ;
#31765=AXIS2_PLACEMENT_3D('',#48808,#39693,#39694) ;
#31766=AXIS2_PLACEMENT_3D('',#48811,#39696,#39697) ;
#31767=AXIS2_PLACEMENT_3D('',#48812,#39698,#39699) ;
#31768=AXIS2_PLACEMENT_3D('',#48813,#39700,#39701) ;
#31769=AXIS2_PLACEMENT_3D('',#48816,#39703,#39704) ;
#31770=AXIS2_PLACEMENT_3D('',#48817,#39705,#39706) ;
#31771=AXIS2_PLACEMENT_3D('',#48818,#39707,#39708) ;
#31772=AXIS2_PLACEMENT_3D('',#48821,#39710,#39711) ;
#31773=AXIS2_PLACEMENT_3D('',#48822,#39712,#39713) ;
#31774=AXIS2_PLACEMENT_3D('',#48823,#39714,#39715) ;
#31775=AXIS2_PLACEMENT_3D('',#48826,#39717,#39718) ;
#31776=AXIS2_PLACEMENT_3D('',#48827,#39719,#39720) ;
#31777=AXIS2_PLACEMENT_3D('',#48828,#39721,#39722) ;
#31778=AXIS2_PLACEMENT_3D('',#48831,#39724,#39725) ;
#31779=AXIS2_PLACEMENT_3D('',#48832,#39726,#39727) ;
#31780=AXIS2_PLACEMENT_3D('',#48833,#39728,#39729) ;
#31781=AXIS2_PLACEMENT_3D('',#48836,#39731,#39732) ;
#31782=AXIS2_PLACEMENT_3D('',#48837,#39733,#39734) ;
#31783=AXIS2_PLACEMENT_3D('',#48838,#39735,#39736) ;
#31784=AXIS2_PLACEMENT_3D('',#48841,#39738,#39739) ;
#31785=AXIS2_PLACEMENT_3D('',#48842,#39740,#39741) ;
#31786=AXIS2_PLACEMENT_3D('',#48843,#39742,#39743) ;
#31787=AXIS2_PLACEMENT_3D('',#48846,#39745,#39746) ;
#31788=AXIS2_PLACEMENT_3D('',#48847,#39747,#39748) ;
#31789=AXIS2_PLACEMENT_3D('',#48848,#39749,#39750) ;
#31790=AXIS2_PLACEMENT_3D('',#48851,#39752,#39753) ;
#31791=AXIS2_PLACEMENT_3D('',#48852,#39754,#39755) ;
#31792=AXIS2_PLACEMENT_3D('',#48853,#39756,#39757) ;
#31793=AXIS2_PLACEMENT_3D('',#48856,#39759,#39760) ;
#31794=AXIS2_PLACEMENT_3D('',#48857,#39761,#39762) ;
#31795=AXIS2_PLACEMENT_3D('',#48858,#39763,#39764) ;
#31796=AXIS2_PLACEMENT_3D('',#48861,#39766,#39767) ;
#31797=AXIS2_PLACEMENT_3D('',#48862,#39768,#39769) ;
#31798=AXIS2_PLACEMENT_3D('',#48863,#39770,#39771) ;
#31799=AXIS2_PLACEMENT_3D('',#48866,#39773,#39774) ;
#31800=AXIS2_PLACEMENT_3D('',#48867,#39775,#39776) ;
#31801=AXIS2_PLACEMENT_3D('',#48868,#39777,#39778) ;
#31802=AXIS2_PLACEMENT_3D('',#48871,#39780,#39781) ;
#31803=AXIS2_PLACEMENT_3D('',#48872,#39782,#39783) ;
#31804=AXIS2_PLACEMENT_3D('',#48873,#39784,#39785) ;
#31805=AXIS2_PLACEMENT_3D('',#48876,#39787,#39788) ;
#31806=AXIS2_PLACEMENT_3D('',#48877,#39789,#39790) ;
#31807=AXIS2_PLACEMENT_3D('',#48878,#39791,#39792) ;
#31808=AXIS2_PLACEMENT_3D('',#48881,#39794,#39795) ;
#31809=AXIS2_PLACEMENT_3D('',#48882,#39796,#39797) ;
#31810=AXIS2_PLACEMENT_3D('',#48883,#39798,#39799) ;
#31811=AXIS2_PLACEMENT_3D('',#48886,#39801,#39802) ;
#31812=AXIS2_PLACEMENT_3D('',#48887,#39803,#39804) ;
#31813=AXIS2_PLACEMENT_3D('',#48888,#39805,#39806) ;
#31814=AXIS2_PLACEMENT_3D('',#48891,#39808,#39809) ;
#31815=AXIS2_PLACEMENT_3D('',#48892,#39810,#39811) ;
#31816=AXIS2_PLACEMENT_3D('',#48893,#39812,#39813) ;
#31817=AXIS2_PLACEMENT_3D('',#48896,#39815,#39816) ;
#31818=AXIS2_PLACEMENT_3D('',#48897,#39817,#39818) ;
#31819=AXIS2_PLACEMENT_3D('',#48898,#39819,#39820) ;
#31820=AXIS2_PLACEMENT_3D('',#48901,#39822,#39823) ;
#31821=AXIS2_PLACEMENT_3D('',#48902,#39824,#39825) ;
#31822=AXIS2_PLACEMENT_3D('',#48903,#39826,#39827) ;
#31823=AXIS2_PLACEMENT_3D('',#48906,#39829,#39830) ;
#31824=AXIS2_PLACEMENT_3D('',#48907,#39831,#39832) ;
#31825=AXIS2_PLACEMENT_3D('',#48908,#39833,#39834) ;
#31826=AXIS2_PLACEMENT_3D('',#48911,#39836,#39837) ;
#31827=AXIS2_PLACEMENT_3D('',#48912,#39838,#39839) ;
#31828=AXIS2_PLACEMENT_3D('',#48913,#39840,#39841) ;
#31829=AXIS2_PLACEMENT_3D('',#48916,#39843,#39844) ;
#31830=AXIS2_PLACEMENT_3D('',#48917,#39845,#39846) ;
#31831=AXIS2_PLACEMENT_3D('',#48918,#39847,#39848) ;
#31832=AXIS2_PLACEMENT_3D('',#48921,#39850,#39851) ;
#31833=AXIS2_PLACEMENT_3D('',#48922,#39852,#39853) ;
#31834=AXIS2_PLACEMENT_3D('',#48923,#39854,#39855) ;
#31835=AXIS2_PLACEMENT_3D('',#48926,#39857,#39858) ;
#31836=AXIS2_PLACEMENT_3D('',#48927,#39859,#39860) ;
#31837=AXIS2_PLACEMENT_3D('',#48928,#39861,#39862) ;
#31838=AXIS2_PLACEMENT_3D('',#48931,#39864,#39865) ;
#31839=AXIS2_PLACEMENT_3D('',#48932,#39866,#39867) ;
#31840=AXIS2_PLACEMENT_3D('',#48933,#39868,#39869) ;
#31841=AXIS2_PLACEMENT_3D('',#48936,#39871,#39872) ;
#31842=AXIS2_PLACEMENT_3D('',#48937,#39873,#39874) ;
#31843=AXIS2_PLACEMENT_3D('',#48938,#39875,#39876) ;
#31844=AXIS2_PLACEMENT_3D('',#48941,#39878,#39879) ;
#31845=AXIS2_PLACEMENT_3D('',#48942,#39880,#39881) ;
#31846=AXIS2_PLACEMENT_3D('',#48943,#39882,#39883) ;
#31847=AXIS2_PLACEMENT_3D('',#48946,#39885,#39886) ;
#31848=AXIS2_PLACEMENT_3D('',#48947,#39887,#39888) ;
#31849=AXIS2_PLACEMENT_3D('',#48948,#39889,#39890) ;
#31850=AXIS2_PLACEMENT_3D('',#48951,#39892,#39893) ;
#31851=AXIS2_PLACEMENT_3D('',#48952,#39894,#39895) ;
#31852=AXIS2_PLACEMENT_3D('',#48953,#39896,#39897) ;
#31853=AXIS2_PLACEMENT_3D('',#48956,#39899,#39900) ;
#31854=AXIS2_PLACEMENT_3D('',#48957,#39901,#39902) ;
#31855=AXIS2_PLACEMENT_3D('',#48958,#39903,#39904) ;
#31856=AXIS2_PLACEMENT_3D('',#48961,#39906,#39907) ;
#31857=AXIS2_PLACEMENT_3D('',#48962,#39908,#39909) ;
#31858=AXIS2_PLACEMENT_3D('',#48963,#39910,#39911) ;
#31859=AXIS2_PLACEMENT_3D('',#48966,#39913,#39914) ;
#31860=AXIS2_PLACEMENT_3D('',#48967,#39915,#39916) ;
#31861=AXIS2_PLACEMENT_3D('',#48968,#39917,#39918) ;
#31862=AXIS2_PLACEMENT_3D('',#48971,#39920,#39921) ;
#31863=AXIS2_PLACEMENT_3D('',#48972,#39922,#39923) ;
#31864=AXIS2_PLACEMENT_3D('',#48973,#39924,#39925) ;
#31865=AXIS2_PLACEMENT_3D('',#48976,#39927,#39928) ;
#31866=AXIS2_PLACEMENT_3D('',#48977,#39929,#39930) ;
#31867=AXIS2_PLACEMENT_3D('',#48978,#39931,#39932) ;
#31868=AXIS2_PLACEMENT_3D('',#48981,#39934,#39935) ;
#31869=AXIS2_PLACEMENT_3D('',#48982,#39936,#39937) ;
#31870=AXIS2_PLACEMENT_3D('',#48983,#39938,#39939) ;
#31871=AXIS2_PLACEMENT_3D('',#48986,#39941,#39942) ;
#31872=AXIS2_PLACEMENT_3D('',#48987,#39943,#39944) ;
#31873=AXIS2_PLACEMENT_3D('',#48988,#39945,#39946) ;
#31874=AXIS2_PLACEMENT_3D('',#48991,#39948,#39949) ;
#31875=AXIS2_PLACEMENT_3D('',#48992,#39950,#39951) ;
#31876=AXIS2_PLACEMENT_3D('',#48993,#39952,#39953) ;
#31877=AXIS2_PLACEMENT_3D('',#48996,#39955,#39956) ;
#31878=AXIS2_PLACEMENT_3D('',#48997,#39957,#39958) ;
#31879=AXIS2_PLACEMENT_3D('',#48998,#39959,#39960) ;
#31880=AXIS2_PLACEMENT_3D('',#49001,#39962,#39963) ;
#31881=AXIS2_PLACEMENT_3D('',#49002,#39964,#39965) ;
#31882=AXIS2_PLACEMENT_3D('',#49003,#39966,#39967) ;
#31883=AXIS2_PLACEMENT_3D('',#49006,#39969,#39970) ;
#31884=AXIS2_PLACEMENT_3D('',#49007,#39971,#39972) ;
#31885=AXIS2_PLACEMENT_3D('',#49008,#39973,#39974) ;
#31886=AXIS2_PLACEMENT_3D('',#49011,#39976,#39977) ;
#31887=AXIS2_PLACEMENT_3D('',#49012,#39978,#39979) ;
#31888=AXIS2_PLACEMENT_3D('',#49013,#39980,#39981) ;
#31889=AXIS2_PLACEMENT_3D('',#49016,#39983,#39984) ;
#31890=AXIS2_PLACEMENT_3D('',#49017,#39985,#39986) ;
#31891=AXIS2_PLACEMENT_3D('',#49018,#39987,#39988) ;
#31892=AXIS2_PLACEMENT_3D('',#49021,#39990,#39991) ;
#31893=AXIS2_PLACEMENT_3D('',#49022,#39992,#39993) ;
#31894=AXIS2_PLACEMENT_3D('',#49023,#39994,#39995) ;
#31895=AXIS2_PLACEMENT_3D('',#49026,#39997,#39998) ;
#31896=AXIS2_PLACEMENT_3D('',#49027,#39999,#40000) ;
#31897=AXIS2_PLACEMENT_3D('',#49028,#40001,#40002) ;
#31898=AXIS2_PLACEMENT_3D('',#49031,#40004,#40005) ;
#31899=AXIS2_PLACEMENT_3D('',#49032,#40006,#40007) ;
#31900=AXIS2_PLACEMENT_3D('',#49033,#40008,#40009) ;
#31901=AXIS2_PLACEMENT_3D('',#49036,#40011,#40012) ;
#31902=AXIS2_PLACEMENT_3D('',#49037,#40013,#40014) ;
#31903=AXIS2_PLACEMENT_3D('',#49038,#40015,#40016) ;
#31904=AXIS2_PLACEMENT_3D('',#49041,#40018,#40019) ;
#31905=AXIS2_PLACEMENT_3D('',#49042,#40020,#40021) ;
#31906=AXIS2_PLACEMENT_3D('',#49043,#40022,#40023) ;
#31907=AXIS2_PLACEMENT_3D('',#49046,#40025,#40026) ;
#31908=AXIS2_PLACEMENT_3D('',#49047,#40027,#40028) ;
#31909=AXIS2_PLACEMENT_3D('',#49048,#40029,#40030) ;
#31910=AXIS2_PLACEMENT_3D('',#49051,#40032,#40033) ;
#31911=AXIS2_PLACEMENT_3D('',#49052,#40034,#40035) ;
#31912=AXIS2_PLACEMENT_3D('',#49053,#40036,#40037) ;
#31913=AXIS2_PLACEMENT_3D('',#49056,#40039,#40040) ;
#31914=AXIS2_PLACEMENT_3D('',#49057,#40041,#40042) ;
#31915=AXIS2_PLACEMENT_3D('',#49058,#40043,#40044) ;
#31916=AXIS2_PLACEMENT_3D('',#49061,#40046,#40047) ;
#31917=AXIS2_PLACEMENT_3D('',#49062,#40048,#40049) ;
#31918=AXIS2_PLACEMENT_3D('',#49063,#40050,#40051) ;
#31919=AXIS2_PLACEMENT_3D('',#49066,#40053,#40054) ;
#31920=AXIS2_PLACEMENT_3D('',#49067,#40055,#40056) ;
#31921=AXIS2_PLACEMENT_3D('',#49068,#40057,#40058) ;
#31922=AXIS2_PLACEMENT_3D('',#49071,#40060,#40061) ;
#31923=AXIS2_PLACEMENT_3D('',#49072,#40062,#40063) ;
#31924=AXIS2_PLACEMENT_3D('',#49073,#40064,#40065) ;
#31925=AXIS2_PLACEMENT_3D('',#49076,#40067,#40068) ;
#31926=AXIS2_PLACEMENT_3D('',#49077,#40069,#40070) ;
#31927=AXIS2_PLACEMENT_3D('',#49078,#40071,#40072) ;
#31928=AXIS2_PLACEMENT_3D('',#49081,#40074,#40075) ;
#31929=AXIS2_PLACEMENT_3D('',#49082,#40076,#40077) ;
#31930=AXIS2_PLACEMENT_3D('',#49083,#40078,#40079) ;
#31931=AXIS2_PLACEMENT_3D('',#49086,#40081,#40082) ;
#31932=AXIS2_PLACEMENT_3D('',#49087,#40083,#40084) ;
#31933=AXIS2_PLACEMENT_3D('',#49088,#40085,#40086) ;
#31934=AXIS2_PLACEMENT_3D('',#49091,#40088,#40089) ;
#31935=AXIS2_PLACEMENT_3D('',#49092,#40090,#40091) ;
#31936=AXIS2_PLACEMENT_3D('',#49093,#40092,#40093) ;
#31937=AXIS2_PLACEMENT_3D('',#49096,#40095,#40096) ;
#31938=AXIS2_PLACEMENT_3D('',#49097,#40097,#40098) ;
#31939=AXIS2_PLACEMENT_3D('',#49098,#40099,#40100) ;
#31940=AXIS2_PLACEMENT_3D('',#49101,#40102,#40103) ;
#31941=AXIS2_PLACEMENT_3D('',#49102,#40104,#40105) ;
#31942=AXIS2_PLACEMENT_3D('',#49103,#40106,#40107) ;
#31943=AXIS2_PLACEMENT_3D('',#49106,#40109,#40110) ;
#31944=AXIS2_PLACEMENT_3D('',#49107,#40111,#40112) ;
#31945=AXIS2_PLACEMENT_3D('',#49108,#40113,#40114) ;
#31946=AXIS2_PLACEMENT_3D('',#49111,#40116,#40117) ;
#31947=AXIS2_PLACEMENT_3D('',#49112,#40118,#40119) ;
#31948=AXIS2_PLACEMENT_3D('',#49113,#40120,#40121) ;
#31949=AXIS2_PLACEMENT_3D('',#49116,#40123,#40124) ;
#31950=AXIS2_PLACEMENT_3D('',#49117,#40125,#40126) ;
#31951=AXIS2_PLACEMENT_3D('',#49118,#40127,#40128) ;
#31952=AXIS2_PLACEMENT_3D('',#49121,#40130,#40131) ;
#31953=AXIS2_PLACEMENT_3D('',#49122,#40132,#40133) ;
#31954=AXIS2_PLACEMENT_3D('',#49123,#40134,#40135) ;
#31955=AXIS2_PLACEMENT_3D('',#49126,#40137,#40138) ;
#31956=AXIS2_PLACEMENT_3D('',#49127,#40139,#40140) ;
#31957=AXIS2_PLACEMENT_3D('',#49128,#40141,#40142) ;
#31958=AXIS2_PLACEMENT_3D('',#49131,#40144,#40145) ;
#31959=AXIS2_PLACEMENT_3D('',#49132,#40146,#40147) ;
#31960=AXIS2_PLACEMENT_3D('',#49133,#40148,#40149) ;
#31961=AXIS2_PLACEMENT_3D('',#49136,#40151,#40152) ;
#31962=AXIS2_PLACEMENT_3D('',#49137,#40153,#40154) ;
#31963=AXIS2_PLACEMENT_3D('',#49138,#40155,#40156) ;
#31964=AXIS2_PLACEMENT_3D('',#49141,#40158,#40159) ;
#31965=AXIS2_PLACEMENT_3D('',#49142,#40160,#40161) ;
#31966=AXIS2_PLACEMENT_3D('',#49143,#40162,#40163) ;
#31967=AXIS2_PLACEMENT_3D('',#49146,#40165,#40166) ;
#31968=AXIS2_PLACEMENT_3D('',#49147,#40167,#40168) ;
#31969=AXIS2_PLACEMENT_3D('',#49148,#40169,#40170) ;
#31970=AXIS2_PLACEMENT_3D('',#49151,#40172,#40173) ;
#31971=AXIS2_PLACEMENT_3D('',#49152,#40174,#40175) ;
#31972=AXIS2_PLACEMENT_3D('',#49153,#40176,#40177) ;
#31973=AXIS2_PLACEMENT_3D('',#49156,#40179,#40180) ;
#31974=AXIS2_PLACEMENT_3D('',#49157,#40181,#40182) ;
#31975=AXIS2_PLACEMENT_3D('',#49158,#40183,#40184) ;
#31976=AXIS2_PLACEMENT_3D('',#49161,#40186,#40187) ;
#31977=AXIS2_PLACEMENT_3D('',#49162,#40188,#40189) ;
#31978=AXIS2_PLACEMENT_3D('',#49163,#40190,#40191) ;
#31979=AXIS2_PLACEMENT_3D('',#49166,#40193,#40194) ;
#31980=AXIS2_PLACEMENT_3D('',#49167,#40195,#40196) ;
#31981=AXIS2_PLACEMENT_3D('',#49168,#40197,#40198) ;
#31982=AXIS2_PLACEMENT_3D('',#49171,#40200,#40201) ;
#31983=AXIS2_PLACEMENT_3D('',#49172,#40202,#40203) ;
#31984=AXIS2_PLACEMENT_3D('',#49173,#40204,#40205) ;
#31985=AXIS2_PLACEMENT_3D('',#49176,#40207,#40208) ;
#31986=AXIS2_PLACEMENT_3D('',#49177,#40209,#40210) ;
#31987=AXIS2_PLACEMENT_3D('',#49178,#40211,#40212) ;
#31988=AXIS2_PLACEMENT_3D('',#49181,#40214,#40215) ;
#31989=AXIS2_PLACEMENT_3D('',#49182,#40216,#40217) ;
#31990=AXIS2_PLACEMENT_3D('',#49183,#40218,#40219) ;
#31991=AXIS2_PLACEMENT_3D('',#49186,#40221,#40222) ;
#31992=AXIS2_PLACEMENT_3D('',#49187,#40223,#40224) ;
#31993=AXIS2_PLACEMENT_3D('',#49188,#40225,#40226) ;
#31994=AXIS2_PLACEMENT_3D('',#49191,#40228,#40229) ;
#31995=AXIS2_PLACEMENT_3D('',#49192,#40230,#40231) ;
#31996=AXIS2_PLACEMENT_3D('',#49193,#40232,#40233) ;
#31997=AXIS2_PLACEMENT_3D('',#49196,#40235,#40236) ;
#31998=AXIS2_PLACEMENT_3D('',#49197,#40237,#40238) ;
#31999=AXIS2_PLACEMENT_3D('',#49198,#40239,#40240) ;
#32000=AXIS2_PLACEMENT_3D('',#49201,#40242,#40243) ;
#32001=AXIS2_PLACEMENT_3D('',#49202,#40244,#40245) ;
#32002=AXIS2_PLACEMENT_3D('',#49203,#40246,#40247) ;
#32003=AXIS2_PLACEMENT_3D('',#49206,#40249,#40250) ;
#32004=AXIS2_PLACEMENT_3D('',#49207,#40251,#40252) ;
#32005=AXIS2_PLACEMENT_3D('',#49208,#40253,#40254) ;
#32006=AXIS2_PLACEMENT_3D('',#49211,#40256,#40257) ;
#32007=AXIS2_PLACEMENT_3D('',#49212,#40258,#40259) ;
#32008=AXIS2_PLACEMENT_3D('',#49213,#40260,#40261) ;
#32009=AXIS2_PLACEMENT_3D('',#49216,#40263,#40264) ;
#32010=AXIS2_PLACEMENT_3D('',#49217,#40265,#40266) ;
#32011=AXIS2_PLACEMENT_3D('',#49218,#40267,#40268) ;
#32012=AXIS2_PLACEMENT_3D('',#49221,#40270,#40271) ;
#32013=AXIS2_PLACEMENT_3D('',#49222,#40272,#40273) ;
#32014=AXIS2_PLACEMENT_3D('',#49223,#40274,#40275) ;
#32015=AXIS2_PLACEMENT_3D('',#49226,#40277,#40278) ;
#32016=AXIS2_PLACEMENT_3D('',#49227,#40279,#40280) ;
#32017=AXIS2_PLACEMENT_3D('',#49228,#40281,#40282) ;
#32018=AXIS2_PLACEMENT_3D('',#49231,#40284,#40285) ;
#32019=AXIS2_PLACEMENT_3D('',#49232,#40286,#40287) ;
#32020=AXIS2_PLACEMENT_3D('',#49233,#40288,#40289) ;
#32021=AXIS2_PLACEMENT_3D('',#49236,#40291,#40292) ;
#32022=AXIS2_PLACEMENT_3D('',#49237,#40293,#40294) ;
#32023=AXIS2_PLACEMENT_3D('',#49238,#40295,#40296) ;
#32024=AXIS2_PLACEMENT_3D('',#49241,#40298,#40299) ;
#32025=AXIS2_PLACEMENT_3D('',#49242,#40300,#40301) ;
#32026=AXIS2_PLACEMENT_3D('',#49243,#40302,#40303) ;
#32027=AXIS2_PLACEMENT_3D('',#49246,#40305,#40306) ;
#32028=AXIS2_PLACEMENT_3D('',#49247,#40307,#40308) ;
#32029=AXIS2_PLACEMENT_3D('',#49248,#40309,#40310) ;
#32030=AXIS2_PLACEMENT_3D('',#49251,#40312,#40313) ;
#32031=AXIS2_PLACEMENT_3D('',#49252,#40314,#40315) ;
#32032=AXIS2_PLACEMENT_3D('',#49253,#40316,#40317) ;
#32033=AXIS2_PLACEMENT_3D('',#49256,#40319,#40320) ;
#32034=AXIS2_PLACEMENT_3D('',#49257,#40321,#40322) ;
#32035=AXIS2_PLACEMENT_3D('',#49258,#40323,#40324) ;
#32036=AXIS2_PLACEMENT_3D('',#49261,#40326,#40327) ;
#32037=AXIS2_PLACEMENT_3D('',#49262,#40328,#40329) ;
#32038=AXIS2_PLACEMENT_3D('',#49263,#40330,#40331) ;
#32039=AXIS2_PLACEMENT_3D('',#49266,#40333,#40334) ;
#32040=AXIS2_PLACEMENT_3D('',#49267,#40335,#40336) ;
#32041=AXIS2_PLACEMENT_3D('',#49268,#40337,#40338) ;
#32042=AXIS2_PLACEMENT_3D('',#49271,#40340,#40341) ;
#32043=AXIS2_PLACEMENT_3D('',#49272,#40342,#40343) ;
#32044=AXIS2_PLACEMENT_3D('',#49273,#40344,#40345) ;
#32045=AXIS2_PLACEMENT_3D('',#49276,#40347,#40348) ;
#32046=AXIS2_PLACEMENT_3D('',#49277,#40349,#40350) ;
#32047=AXIS2_PLACEMENT_3D('',#49278,#40351,#40352) ;
#32048=AXIS2_PLACEMENT_3D('',#49281,#40354,#40355) ;
#32049=AXIS2_PLACEMENT_3D('',#49282,#40356,#40357) ;
#32050=AXIS2_PLACEMENT_3D('',#49283,#40358,#40359) ;
#32051=AXIS2_PLACEMENT_3D('',#49286,#40361,#40362) ;
#32052=AXIS2_PLACEMENT_3D('',#49287,#40363,#40364) ;
#32053=AXIS2_PLACEMENT_3D('',#49288,#40365,#40366) ;
#32054=AXIS2_PLACEMENT_3D('',#49291,#40368,#40369) ;
#32055=AXIS2_PLACEMENT_3D('',#49292,#40370,#40371) ;
#32056=AXIS2_PLACEMENT_3D('',#49293,#40372,#40373) ;
#32057=AXIS2_PLACEMENT_3D('',#49295,#40374,#40375) ;
#32058=AXIS2_PLACEMENT_3D('',#49319,#40378,#40379) ;
#32059=AXIS2_PLACEMENT_3D('',#49341,#40380,#40381) ;
#32060=AXIS2_PLACEMENT_3D('',#49343,#40382,#40383) ;
#32061=AXIS2_PLACEMENT_3D('',#49346,#40385,#40386) ;
#32062=AXIS2_PLACEMENT_3D('',#49347,#40387,#40388) ;
#32063=AXIS2_PLACEMENT_3D('',#49348,#40389,#40390) ;
#32064=AXIS2_PLACEMENT_3D('',#49349,#40391,#40392) ;
#32065=AXIS2_PLACEMENT_3D('',#49352,#40394,#40395) ;
#32066=AXIS2_PLACEMENT_3D('',#49353,#40396,#40397) ;
#38264=DIRECTION('axis',(0.,0.,1.)) ;
#38265=DIRECTION('refdir',(1.,0.,0.)) ;
#38266=DIRECTION('center_axis',(0.,0.,1.)) ;
#38267=DIRECTION('ref_axis',(1.,0.,0.)) ;
#38268=DIRECTION('center_axis',(0.,0.,1.)) ;
#38269=DIRECTION('ref_axis',(1.,0.,0.)) ;
#38270=DIRECTION('',(0.,0.,-1.)) ;
#38271=DIRECTION('center_axis',(0.,0.,-1.)) ;
#38272=DIRECTION('ref_axis',(1.,0.,0.)) ;
#38273=DIRECTION('center_axis',(0.,0.,1.)) ;
#38274=DIRECTION('ref_axis',(1.,0.,0.)) ;
#38275=DIRECTION('center_axis',(0.,0.,1.)) ;
#38276=DIRECTION('ref_axis',(1.,0.,0.)) ;
#38277=DIRECTION('',(0.,0.,1.)) ;
#38278=DIRECTION('center_axis',(0.,0.,-1.)) ;
#38279=DIRECTION('ref_axis',(1.,0.,0.)) ;
#38280=DIRECTION('center_axis',(0.,0.,-1.)) ;
#38281=DIRECTION('ref_axis',(-1.,0.,0.)) ;
#38282=DIRECTION('center_axis',(0.,0.,1.)) ;
#38283=DIRECTION('ref_axis',(1.,0.,0.)) ;
#38284=DIRECTION('center_axis',(0.94299033358289,0.,0.332820117735135)) ;
#38285=DIRECTION('ref_axis',(0.332820117735135,0.,-0.94299033358289)) ;
#38286=DIRECTION('center_axis',(0.94299033358289,0.,0.332820117735135)) ;
#38287=DIRECTION('ref_axis',(0.332820117735135,0.,-0.94299033358289)) ;
#38288=DIRECTION('',(-0.94299033358289,0.,-0.332820117735135)) ;
#38289=DIRECTION('center_axis',(0.94299033358289,0.,0.332820117735135)) ;
#38290=DIRECTION('ref_axis',(0.332820117735135,0.,-0.94299033358289)) ;
#38291=DIRECTION('center_axis',(1.,0.,0.)) ;
#38292=DIRECTION('ref_axis',(0.,0.,-1.)) ;
#38293=DIRECTION('center_axis',(1.,0.,0.)) ;
#38294=DIRECTION('ref_axis',(0.,0.,-1.)) ;
#38295=DIRECTION('',(1.,0.,0.)) ;
#38296=DIRECTION('center_axis',(-1.,0.,0.)) ;
#38297=DIRECTION('ref_axis',(0.,0.,-1.)) ;
#38298=DIRECTION('center_axis',(1.,0.,0.)) ;
#38299=DIRECTION('ref_axis',(0.,0.,-1.)) ;
#38300=DIRECTION('center_axis',(1.,0.,0.)) ;
#38301=DIRECTION('ref_axis',(0.,0.,-1.)) ;
#38302=DIRECTION('',(-1.,0.,0.)) ;
#38303=DIRECTION('center_axis',(-1.,0.,0.)) ;
#38304=DIRECTION('ref_axis',(0.,0.,-1.)) ;
#38305=DIRECTION('center_axis',(-1.,0.,0.)) ;
#38306=DIRECTION('ref_axis',(0.,0.,1.)) ;
#38307=DIRECTION('center_axis',(1.,0.,0.)) ;
#38308=DIRECTION('ref_axis',(0.,0.,-1.)) ;
#38309=DIRECTION('center_axis',(1.,0.,0.)) ;
#38310=DIRECTION('ref_axis',(0.,0.,-1.)) ;
#38311=DIRECTION('center_axis',(0.091482478332531,-0.920005415661246,0.381078720623595)) ;
#38312=DIRECTION('ref_axis',(0.995806686138499,0.0845187893148324,-0.0350088288095587)) ;
#38313=DIRECTION('center_axis',(1.,0.,0.)) ;
#38314=DIRECTION('ref_axis',(0.,0.,-1.)) ;
#38315=DIRECTION('',(1.,0.,0.)) ;
#38316=DIRECTION('center_axis',(-1.,0.,0.)) ;
#38317=DIRECTION('ref_axis',(0.,0.,-1.)) ;
#38318=DIRECTION('center_axis',(1.,0.,0.)) ;
#38319=DIRECTION('ref_axis',(0.,0.,-1.)) ;
#38320=DIRECTION('center_axis',(1.,0.,0.)) ;
#38321=DIRECTION('ref_axis',(0.,0.,-1.)) ;
#38322=DIRECTION('',(-1.,0.,0.)) ;
#38323=DIRECTION('center_axis',(-1.,0.,0.)) ;
#38324=DIRECTION('ref_axis',(0.,0.,-1.)) ;
#38325=DIRECTION('center_axis',(-1.,0.,0.)) ;
#38326=DIRECTION('ref_axis',(0.,0.,1.)) ;
#38327=DIRECTION('',(0.,0.382683432365099,0.923879532511283)) ;
#38328=DIRECTION('center_axis',(-1.,0.,0.)) ;
#38329=DIRECTION('ref_axis',(0.,-0.382683432365094,-0.923879532511285)) ;
#38330=DIRECTION('center_axis',(-1.,0.,0.)) ;
#38331=DIRECTION('ref_axis',(0.,0.,-1.)) ;
#38332=DIRECTION('center_axis',(-1.,0.,0.)) ;
#38333=DIRECTION('ref_axis',(0.,0.38268343236509,-0.923879532511287)) ;
#38334=DIRECTION('center_axis',(-1.,0.,0.)) ;
#38335=DIRECTION('ref_axis',(0.,0.,-1.)) ;
#38336=DIRECTION('center_axis',(-1.,0.,0.)) ;
#38337=DIRECTION('ref_axis',(0.,0.923879532511283,-0.382683432365099)) ;
#38338=DIRECTION('center_axis',(1.,0.,0.)) ;
#38339=DIRECTION('ref_axis',(0.,0.,-1.)) ;
#38340=DIRECTION('center_axis',(0.091482478332531,-0.920005415661246,0.381078720623595)) ;
#38341=DIRECTION('ref_axis',(0.995806686138499,0.0845187893148324,-0.0350088288095587)) ;
#38342=DIRECTION('center_axis',(0.091482478332531,-0.920005415661246,0.381078720623595)) ;
#38343=DIRECTION('ref_axis',(0.995806686138498,0.0845187893148324,-0.0350088288095587)) ;
#38344=DIRECTION('center_axis',(0.,0.,1.)) ;
#38345=DIRECTION('ref_axis',(-0.421632036455268,0.906767018497356,0.)) ;
#38346=DIRECTION('center_axis',(0.0914824783325255,-0.381078720623586,0.92000541566125)) ;
#38347=DIRECTION('ref_axis',(0.995806686138499,0.0350088288095558,-0.0845187893148275)) ;
#38348=DIRECTION('center_axis',(-0.091482478332531,0.920005415661246,-0.381078720623595)) ;
#38349=DIRECTION('ref_axis',(0.995806686138498,0.0845187893148324,-0.0350088288095587)) ;
#38350=DIRECTION('center_axis',(0.,0.,1.)) ;
#38351=DIRECTION('ref_axis',(1.,0.,0.)) ;
#38352=DIRECTION('center_axis',(0.0914824783325241,0.381078720623591,0.920005415661248)) ;
#38353=DIRECTION('ref_axis',(0.995806686138499,-0.0350088288095557,-0.0845187893148261)) ;
#38354=DIRECTION('center_axis',(0.0914824783325241,0.381078720623591,0.920005415661248)) ;
#38355=DIRECTION('ref_axis',(0.995806686138499,-0.0350088288095557,-0.0845187893148261)) ;
#38356=DIRECTION('center_axis',(-0.0914824783325255,0.381078720623586,-0.92000541566125)) ;
#38357=DIRECTION('ref_axis',(0.995806686138499,0.0350088288095558,-0.0845187893148275)) ;
#38358=DIRECTION('center_axis',(0.,0.,1.)) ;
#38359=DIRECTION('ref_axis',(1.,0.,0.)) ;
#38360=DIRECTION('center_axis',(-0.0914824783325241,-0.381078720623591,
-0.920005415661248)) ;
#38361=DIRECTION('ref_axis',(0.995806686138499,-0.0350088288095557,-0.0845187893148261)) ;
#38362=DIRECTION('center_axis',(0.0914824783325315,0.920005415661255,0.381078720623574)) ;
#38363=DIRECTION('ref_axis',(0.995806686138498,-0.0845187893148336,-0.035008828809557)) ;
#38364=DIRECTION('center_axis',(0.0914824783325315,0.920005415661255,0.381078720623574)) ;
#38365=DIRECTION('ref_axis',(0.995806686138498,-0.0845187893148336,-0.035008828809557)) ;
#38366=DIRECTION('center_axis',(0.,0.,1.)) ;
#38367=DIRECTION('ref_axis',(1.,0.,0.)) ;
#38368=DIRECTION('center_axis',(-0.0914824783325315,-0.920005415661255,
-0.381078720623574)) ;
#38369=DIRECTION('ref_axis',(0.995806686138498,-0.0845187893148336,-0.035008828809557)) ;
#38370=DIRECTION('center_axis',(0.0914824783325258,0.92000541566125,-0.381078720623586)) ;
#38371=DIRECTION('ref_axis',(0.995806686138499,-0.0845187893148279,0.0350088288095559)) ;
#38372=DIRECTION('center_axis',(1.22464679914737E-16,-1.,0.)) ;
#38373=DIRECTION('ref_axis',(-1.,-1.22464679914737E-16,0.)) ;
#38374=DIRECTION('center_axis',(0.0914824783325258,0.92000541566125,-0.381078720623586)) ;
#38375=DIRECTION('ref_axis',(0.995806686138499,-0.0845187893148279,0.0350088288095559)) ;
#38376=DIRECTION('center_axis',(0.0914824783325258,0.92000541566125,-0.381078720623586)) ;
#38377=DIRECTION('ref_axis',(0.995806686138499,-0.0845187893148279,0.0350088288095559)) ;
#38378=DIRECTION('center_axis',(0.,0.,1.)) ;
#38379=DIRECTION('ref_axis',(-0.0701393346692214,-0.997537204184465,0.)) ;
#38380=DIRECTION('center_axis',(-0.0914824783325258,-0.92000541566125,0.381078720623586)) ;
#38381=DIRECTION('ref_axis',(0.995806686138499,-0.0845187893148279,0.0350088288095559)) ;
#38382=DIRECTION('center_axis',(0.0914824783325313,0.381078720623583,-0.920005415661251)) ;
#38383=DIRECTION('ref_axis',(0.995806686138498,-0.0350088288095578,0.084518789314833)) ;
#38384=DIRECTION('center_axis',(0.0914824783325313,0.381078720623583,-0.920005415661251)) ;
#38385=DIRECTION('ref_axis',(0.995806686138498,-0.0350088288095578,0.084518789314833)) ;
#38386=DIRECTION('center_axis',(0.,0.,1.)) ;
#38387=DIRECTION('ref_axis',(1.,0.,0.)) ;
#38388=DIRECTION('center_axis',(-0.0914824783325313,-0.381078720623583,
0.920005415661251)) ;
#38389=DIRECTION('ref_axis',(0.995806686138498,-0.0350088288095578,0.084518789314833)) ;
#38390=DIRECTION('center_axis',(0.0914824783325254,-0.381078720623587,-0.92000541566125)) ;
#38391=DIRECTION('ref_axis',(0.995806686138499,0.0350088288095558,0.0845187893148275)) ;
#38392=DIRECTION('center_axis',(0.0914824783325254,-0.381078720623587,-0.92000541566125)) ;
#38393=DIRECTION('ref_axis',(0.995806686138499,0.0350088288095558,0.0845187893148275)) ;
#38394=DIRECTION('center_axis',(0.,0.,1.)) ;
#38395=DIRECTION('ref_axis',(1.,0.,0.)) ;
#38396=DIRECTION('center_axis',(-0.0914824783325254,0.381078720623587,0.92000541566125)) ;
#38397=DIRECTION('ref_axis',(0.995806686138499,0.0350088288095558,0.0845187893148275)) ;
#38398=DIRECTION('center_axis',(0.0914824783325237,-0.920005415661249,-0.381078720623589)) ;
#38399=DIRECTION('ref_axis',(0.995806686138499,0.0845187893148259,0.0350088288095553)) ;
#38400=DIRECTION('center_axis',(0.0914824783325237,-0.920005415661249,-0.381078720623589)) ;
#38401=DIRECTION('ref_axis',(0.995806686138499,0.0845187893148259,0.0350088288095553)) ;
#38402=DIRECTION('center_axis',(0.,0.,1.)) ;
#38403=DIRECTION('ref_axis',(1.,0.,0.)) ;
#38404=DIRECTION('center_axis',(-0.0914824783325237,0.920005415661249,0.381078720623589)) ;
#38405=DIRECTION('ref_axis',(0.995806686138499,0.0845187893148259,0.0350088288095553)) ;
#38406=DIRECTION('center_axis',(0.0914824783325308,-0.920005415661242,0.381078720623606)) ;
#38407=DIRECTION('ref_axis',(0.995806686138498,0.0845187893148318,-0.0350088288095597)) ;
#38408=DIRECTION('center_axis',(1.22464679914732E-16,-1.,0.)) ;
#38409=DIRECTION('ref_axis',(-1.,-1.22464679914732E-16,0.)) ;
#38410=DIRECTION('center_axis',(0.0914824783325308,-0.920005415661242,0.381078720623606)) ;
#38411=DIRECTION('ref_axis',(0.995806686138498,0.0845187893148318,-0.0350088288095597)) ;
#38412=DIRECTION('center_axis',(0.0914824783325308,-0.920005415661242,0.381078720623606)) ;
#38413=DIRECTION('ref_axis',(0.995806686138498,0.0845187893148318,-0.0350088288095597)) ;
#38414=DIRECTION('center_axis',(0.,0.,1.)) ;
#38415=DIRECTION('ref_axis',(-0.0701393346692214,0.997537204184465,0.)) ;
#38416=DIRECTION('center_axis',(-0.0914824783325308,0.920005415661242,-0.381078720623606)) ;
#38417=DIRECTION('ref_axis',(0.995806686138498,0.0845187893148318,-0.0350088288095597)) ;
#38418=DIRECTION('center_axis',(0.0914824783325257,-0.381078720623581,0.920005415661252)) ;
#38419=DIRECTION('ref_axis',(0.995806686138499,0.0350088288095554,-0.0845187893148279)) ;
#38420=DIRECTION('center_axis',(0.0914824783325257,-0.381078720623581,0.920005415661252)) ;
#38421=DIRECTION('ref_axis',(0.995806686138499,0.0350088288095554,-0.0845187893148279)) ;
#38422=DIRECTION('center_axis',(0.,0.,1.)) ;
#38423=DIRECTION('ref_axis',(1.,0.,0.)) ;
#38424=DIRECTION('center_axis',(-0.0914824783325257,0.381078720623581,-0.920005415661252)) ;
#38425=DIRECTION('ref_axis',(0.995806686138499,0.0350088288095554,-0.0845187893148279)) ;
#38426=DIRECTION('center_axis',(0.091482478332532,0.381078720623593,0.920005415661247)) ;
#38427=DIRECTION('ref_axis',(0.995806686138498,-0.0350088288095589,-0.0845187893148333)) ;
#38428=DIRECTION('center_axis',(0.091482478332532,0.381078720623593,0.920005415661247)) ;
#38429=DIRECTION('ref_axis',(0.995806686138498,-0.0350088288095589,-0.0845187893148333)) ;
#38430=DIRECTION('center_axis',(0.,0.,1.)) ;
#38431=DIRECTION('ref_axis',(1.,0.,0.)) ;
#38432=DIRECTION('center_axis',(-0.091482478332532,-0.381078720623593,-0.920005415661247)) ;
#38433=DIRECTION('ref_axis',(0.995806686138498,-0.0350088288095589,-0.0845187893148333)) ;
#38434=DIRECTION('center_axis',(0.0914824783325256,0.920005415661251,0.381078720623585)) ;
#38435=DIRECTION('ref_axis',(0.995806686138499,-0.0845187893148277,-0.0350088288095557)) ;
#38436=DIRECTION('center_axis',(0.0914824783325256,0.920005415661251,0.381078720623585)) ;
#38437=DIRECTION('ref_axis',(0.995806686138499,-0.0845187893148277,-0.0350088288095557)) ;
#38438=DIRECTION('center_axis',(0.,0.,1.)) ;
#38439=DIRECTION('ref_axis',(1.,0.,0.)) ;
#38440=DIRECTION('center_axis',(-0.0914824783325256,-0.920005415661251,
-0.381078720623585)) ;
#38441=DIRECTION('ref_axis',(0.995806686138499,-0.0845187893148277,-0.0350088288095557)) ;
#38442=DIRECTION('center_axis',(0.0914824783325256,0.920005415661251,-0.381078720623585)) ;
#38443=DIRECTION('ref_axis',(0.995806686138499,-0.0845187893148277,0.0350088288095557)) ;
#38444=DIRECTION('center_axis',(1.22464679914737E-16,-1.,0.)) ;
#38445=DIRECTION('ref_axis',(-1.,-1.22464679914737E-16,0.)) ;
#38446=DIRECTION('center_axis',(0.0914824783325256,0.920005415661251,-0.381078720623585)) ;
#38447=DIRECTION('ref_axis',(0.995806686138499,-0.0845187893148277,0.0350088288095557)) ;
#38448=DIRECTION('center_axis',(0.0914824783325256,0.920005415661251,-0.381078720623585)) ;
#38449=DIRECTION('ref_axis',(0.995806686138499,-0.0845187893148277,0.0350088288095557)) ;
#38450=DIRECTION('center_axis',(0.,0.,1.)) ;
#38451=DIRECTION('ref_axis',(-0.0701393346692214,-0.997537204184465,0.)) ;
#38452=DIRECTION('center_axis',(-0.0914824783325256,-0.920005415661251,
0.381078720623585)) ;
#38453=DIRECTION('ref_axis',(0.995806686138499,-0.0845187893148277,0.0350088288095557)) ;
#38454=DIRECTION('center_axis',(0.0914824783325301,0.381078720623585,-0.92000541566125)) ;
#38455=DIRECTION('ref_axis',(0.995806686138499,-0.0350088288095575,0.0845187893148319)) ;
#38456=DIRECTION('center_axis',(0.0914824783325301,0.381078720623585,-0.92000541566125)) ;
#38457=DIRECTION('ref_axis',(0.995806686138499,-0.0350088288095575,0.0845187893148319)) ;
#38458=DIRECTION('center_axis',(0.,0.,1.)) ;
#38459=DIRECTION('ref_axis',(1.,0.,0.)) ;
#38460=DIRECTION('center_axis',(-0.0914824783325301,-0.381078720623585,
0.92000541566125)) ;
#38461=DIRECTION('ref_axis',(0.995806686138499,-0.0350088288095575,0.0845187893148319)) ;
#38462=DIRECTION('center_axis',(0.0914824783325252,-0.381078720623592,-0.920005415661248)) ;
#38463=DIRECTION('ref_axis',(0.995806686138499,0.0350088288095562,0.0845187893148271)) ;
#38464=DIRECTION('center_axis',(0.0914824783325252,-0.381078720623592,-0.920005415661248)) ;
#38465=DIRECTION('ref_axis',(0.995806686138499,0.0350088288095562,0.0845187893148271)) ;
#38466=DIRECTION('center_axis',(0.,0.,1.)) ;
#38467=DIRECTION('ref_axis',(1.,0.,0.)) ;
#38468=DIRECTION('center_axis',(-0.0914824783325252,0.381078720623592,0.920005415661248)) ;
#38469=DIRECTION('ref_axis',(0.995806686138499,0.0350088288095562,0.0845187893148271)) ;
#38470=DIRECTION('center_axis',(0.0914824783325312,-0.920005415661251,-0.381078720623584)) ;
#38471=DIRECTION('ref_axis',(0.995806686138498,0.0845187893148329,0.0350088288095578)) ;
#38472=DIRECTION('center_axis',(0.0914824783325312,-0.920005415661251,-0.381078720623584)) ;
#38473=DIRECTION('ref_axis',(0.995806686138498,0.0845187893148329,0.0350088288095578)) ;
#38474=DIRECTION('center_axis',(0.,0.,1.)) ;
#38475=DIRECTION('ref_axis',(1.,0.,0.)) ;
#38476=DIRECTION('center_axis',(-0.0914824783325312,0.920005415661251,0.381078720623584)) ;
#38477=DIRECTION('ref_axis',(0.995806686138498,0.0845187893148329,0.0350088288095578)) ;
#38478=DIRECTION('center_axis',(0.0914824783325253,-0.920005415661246,0.381078720623595)) ;
#38479=DIRECTION('ref_axis',(0.995806686138499,0.0845187893148271,-0.0350088288095565)) ;
#38480=DIRECTION('center_axis',(1.22464679914737E-16,-1.,0.)) ;
#38481=DIRECTION('ref_axis',(-1.,-1.22464679914737E-16,0.)) ;
#38482=DIRECTION('center_axis',(0.0914824783325253,-0.920005415661246,0.381078720623595)) ;
#38483=DIRECTION('ref_axis',(0.995806686138499,0.0845187893148271,-0.0350088288095565)) ;
#38484=DIRECTION('center_axis',(0.0914824783325253,-0.920005415661246,0.381078720623595)) ;
#38485=DIRECTION('ref_axis',(0.995806686138499,0.0845187893148271,-0.0350088288095565)) ;
#38486=DIRECTION('center_axis',(0.,0.,1.)) ;
#38487=DIRECTION('ref_axis',(-0.0701393346692214,0.997537204184465,0.)) ;
#38488=DIRECTION('center_axis',(-0.0914824783325253,0.920005415661246,-0.381078720623595)) ;
#38489=DIRECTION('ref_axis',(0.995806686138499,0.0845187893148271,-0.0350088288095565)) ;
#38490=DIRECTION('center_axis',(0.0914824783325254,-0.381078720623587,0.92000541566125)) ;
#38491=DIRECTION('ref_axis',(0.995806686138499,0.0350088288095558,-0.0845187893148275)) ;
#38492=DIRECTION('center_axis',(0.0914824783325254,-0.381078720623587,0.92000541566125)) ;
#38493=DIRECTION('ref_axis',(0.995806686138499,0.0350088288095558,-0.0845187893148275)) ;
#38494=DIRECTION('center_axis',(0.,0.,1.)) ;
#38495=DIRECTION('ref_axis',(1.,0.,0.)) ;
#38496=DIRECTION('center_axis',(-0.0914824783325254,0.381078720623587,-0.92000541566125)) ;
#38497=DIRECTION('ref_axis',(0.995806686138499,0.0350088288095558,-0.0845187893148275)) ;
#38498=DIRECTION('center_axis',(0.0914824783325299,0.38107872062359,0.920005415661248)) ;
#38499=DIRECTION('ref_axis',(0.995806686138498,-0.0350088288095579,-0.0845187893148314)) ;
#38500=DIRECTION('center_axis',(0.0914824783325299,0.38107872062359,0.920005415661248)) ;
#38501=DIRECTION('ref_axis',(0.995806686138498,-0.0350088288095579,-0.0845187893148314)) ;
#38502=DIRECTION('center_axis',(0.,0.,1.)) ;
#38503=DIRECTION('ref_axis',(1.,0.,0.)) ;
#38504=DIRECTION('center_axis',(-0.0914824783325299,-0.38107872062359,-0.920005415661248)) ;
#38505=DIRECTION('ref_axis',(0.995806686138498,-0.0350088288095579,-0.0845187893148314)) ;
#38506=DIRECTION('center_axis',(0.0914824783325257,0.920005415661255,0.381078720623574)) ;
#38507=DIRECTION('ref_axis',(0.995806686138499,-0.0845187893148283,-0.0350088288095548)) ;
#38508=DIRECTION('center_axis',(0.0914824783325257,0.920005415661255,0.381078720623574)) ;
#38509=DIRECTION('ref_axis',(0.995806686138499,-0.0845187893148283,-0.0350088288095548)) ;
#38510=DIRECTION('center_axis',(0.,0.,1.)) ;
#38511=DIRECTION('ref_axis',(1.,0.,0.)) ;
#38512=DIRECTION('center_axis',(-0.0914824783325257,-0.920005415661255,
-0.381078720623574)) ;
#38513=DIRECTION('ref_axis',(0.995806686138499,-0.0845187893148283,-0.0350088288095548)) ;
#38514=DIRECTION('center_axis',(0.0914824783325315,0.92000541566125,-0.381078720623586)) ;
#38515=DIRECTION('ref_axis',(0.995806686138498,-0.0845187893148332,0.0350088288095581)) ;
#38516=DIRECTION('center_axis',(1.22464679914737E-16,-1.,0.)) ;
#38517=DIRECTION('ref_axis',(-1.,-1.22464679914737E-16,0.)) ;
#38518=DIRECTION('center_axis',(0.0914824783325315,0.92000541566125,-0.381078720623586)) ;
#38519=DIRECTION('ref_axis',(0.995806686138498,-0.0845187893148332,0.0350088288095581)) ;
#38520=DIRECTION('center_axis',(0.0914824783325315,0.92000541566125,-0.381078720623586)) ;
#38521=DIRECTION('ref_axis',(0.995806686138498,-0.0845187893148332,0.0350088288095581)) ;
#38522=DIRECTION('center_axis',(0.,0.,1.)) ;
#38523=DIRECTION('ref_axis',(-0.0701393346692214,-0.997537204184465,0.)) ;
#38524=DIRECTION('center_axis',(-0.0914824783325315,-0.92000541566125,0.381078720623586)) ;
#38525=DIRECTION('ref_axis',(0.995806686138498,-0.0845187893148332,0.0350088288095581)) ;
#38526=DIRECTION('center_axis',(0.0914824783325256,0.381078720623584,-0.920005415661251)) ;
#38527=DIRECTION('ref_axis',(0.995806686138499,-0.0350088288095556,0.0845187893148277)) ;
#38528=DIRECTION('center_axis',(0.0914824783325256,0.381078720623584,-0.920005415661251)) ;
#38529=DIRECTION('ref_axis',(0.995806686138499,-0.0350088288095556,0.0845187893148277)) ;
#38530=DIRECTION('center_axis',(0.,0.,1.)) ;
#38531=DIRECTION('ref_axis',(1.,0.,0.)) ;
#38532=DIRECTION('center_axis',(-0.0914824783325256,-0.381078720623584,
0.920005415661251)) ;
#38533=DIRECTION('ref_axis',(0.995806686138499,-0.0350088288095556,0.0845187893148277)) ;
#38534=DIRECTION('center_axis',(0.0914824783325255,-0.381078720623586,-0.92000541566125)) ;
#38535=DIRECTION('ref_axis',(0.995806686138499,0.0350088288095558,0.0845187893148275)) ;
#38536=DIRECTION('center_axis',(0.0914824783325255,-0.381078720623586,-0.92000541566125)) ;
#38537=DIRECTION('ref_axis',(0.995806686138499,0.0350088288095558,0.0845187893148275)) ;
#38538=DIRECTION('center_axis',(0.,0.,1.)) ;
#38539=DIRECTION('ref_axis',(1.,0.,0.)) ;
#38540=DIRECTION('center_axis',(-0.0914824783325255,0.381078720623586,0.92000541566125)) ;
#38541=DIRECTION('ref_axis',(0.995806686138499,0.0350088288095558,0.0845187893148275)) ;
#38542=DIRECTION('center_axis',(0.091482478332531,-0.920005415661246,-0.381078720623595)) ;
#38543=DIRECTION('ref_axis',(0.995806686138498,0.0845187893148324,0.0350088288095587)) ;
#38544=DIRECTION('center_axis',(0.091482478332531,-0.920005415661246,-0.381078720623595)) ;
#38545=DIRECTION('ref_axis',(0.995806686138498,0.0845187893148324,0.0350088288095587)) ;
#38546=DIRECTION('center_axis',(0.,0.,1.)) ;
#38547=DIRECTION('ref_axis',(1.,0.,0.)) ;
#38548=DIRECTION('center_axis',(-0.091482478332531,0.920005415661246,0.381078720623595)) ;
#38549=DIRECTION('ref_axis',(0.995806686138498,0.0845187893148324,0.0350088288095587)) ;
#38550=DIRECTION('center_axis',(0.0914824783325236,-0.920005415661245,0.3810787206236)) ;
#38551=DIRECTION('ref_axis',(0.995806686138499,0.0845187893148253,-0.0350088288095563)) ;
#38552=DIRECTION('center_axis',(1.22464679914737E-16,-1.,0.)) ;
#38553=DIRECTION('ref_axis',(-1.,-1.22464679914737E-16,0.)) ;
#38554=DIRECTION('center_axis',(0.0914824783325236,-0.920005415661245,0.3810787206236)) ;
#38555=DIRECTION('ref_axis',(0.995806686138499,0.0845187893148253,-0.0350088288095563)) ;
#38556=DIRECTION('center_axis',(0.0914824783325236,-0.920005415661245,0.3810787206236)) ;
#38557=DIRECTION('ref_axis',(0.995806686138499,0.0845187893148253,-0.0350088288095563)) ;
#38558=DIRECTION('center_axis',(0.,0.,1.)) ;
#38559=DIRECTION('ref_axis',(-0.0701393346692214,0.997537204184465,0.)) ;
#38560=DIRECTION('center_axis',(-0.0914824783325236,0.920005415661245,-0.3810787206236)) ;
#38561=DIRECTION('ref_axis',(0.995806686138499,0.0845187893148253,-0.0350088288095563)) ;
#38562=DIRECTION('center_axis',(0.0914824783325314,-0.381078720623581,0.920005415661252)) ;
#38563=DIRECTION('ref_axis',(0.995806686138498,0.0350088288095576,-0.0845187893148332)) ;
#38564=DIRECTION('center_axis',(0.0914824783325314,-0.381078720623581,0.920005415661252)) ;
#38565=DIRECTION('ref_axis',(0.995806686138498,0.0350088288095576,-0.0845187893148332)) ;
#38566=DIRECTION('center_axis',(0.,0.,1.)) ;
#38567=DIRECTION('ref_axis',(1.,0.,0.)) ;
#38568=DIRECTION('center_axis',(-0.0914824783325314,0.381078720623581,-0.920005415661252)) ;
#38569=DIRECTION('ref_axis',(0.995806686138498,0.0350088288095576,-0.0845187893148332)) ;
#38570=DIRECTION('center_axis',(0.0914824783325263,0.381078720623593,0.920005415661247)) ;
#38571=DIRECTION('ref_axis',(0.995806686138499,-0.0350088288095567,-0.0845187893148281)) ;
#38572=DIRECTION('center_axis',(0.0914824783325263,0.381078720623593,0.920005415661247)) ;
#38573=DIRECTION('ref_axis',(0.995806686138499,-0.0350088288095567,-0.0845187893148281)) ;
#38574=DIRECTION('center_axis',(0.,0.,1.)) ;
#38575=DIRECTION('ref_axis',(1.,0.,0.)) ;
#38576=DIRECTION('center_axis',(-0.0914824783325263,-0.381078720623593,
-0.920005415661247)) ;
#38577=DIRECTION('ref_axis',(0.995806686138499,-0.0350088288095567,-0.0845187893148281)) ;
#38578=DIRECTION('center_axis',(0.0914824783325256,0.920005415661251,0.381078720623585)) ;
#38579=DIRECTION('ref_axis',(0.995806686138499,-0.0845187893148277,-0.0350088288095557)) ;
#38580=DIRECTION('center_axis',(0.0914824783325256,0.920005415661251,0.381078720623585)) ;
#38581=DIRECTION('ref_axis',(0.995806686138499,-0.0845187893148277,-0.0350088288095557)) ;
#38582=DIRECTION('center_axis',(0.,0.,1.)) ;
#38583=DIRECTION('ref_axis',(1.,0.,0.)) ;
#38584=DIRECTION('center_axis',(-0.0914824783325256,-0.920005415661251,
-0.381078720623585)) ;
#38585=DIRECTION('ref_axis',(0.995806686138499,-0.0845187893148277,-0.0350088288095557)) ;
#38586=DIRECTION('center_axis',(0.0914824783325317,0.920005415661254,-0.381078720623575)) ;
#38587=DIRECTION('ref_axis',(0.995806686138498,-0.0845187893148337,0.0350088288095571)) ;
#38588=DIRECTION('center_axis',(1.22464679914736E-16,-1.,0.)) ;
#38589=DIRECTION('ref_axis',(-1.,-1.22464679914736E-16,0.)) ;
#38590=DIRECTION('center_axis',(0.0914824783325317,0.920005415661254,-0.381078720623575)) ;
#38591=DIRECTION('ref_axis',(0.995806686138498,-0.0845187893148337,0.0350088288095571)) ;
#38592=DIRECTION('center_axis',(0.0914824783325317,0.920005415661254,-0.381078720623575)) ;
#38593=DIRECTION('ref_axis',(0.995806686138498,-0.0845187893148337,0.0350088288095571)) ;
#38594=DIRECTION('center_axis',(0.,0.,1.)) ;
#38595=DIRECTION('ref_axis',(-0.0701393346692214,-0.997537204184465,0.)) ;
#38596=DIRECTION('center_axis',(-0.0914824783325317,-0.920005415661254,
0.381078720623575)) ;
#38597=DIRECTION('ref_axis',(0.995806686138498,-0.0845187893148337,0.0350088288095571)) ;
#38598=DIRECTION('center_axis',(0.0914824783325234,0.381078720623582,-0.920005415661252)) ;
#38599=DIRECTION('ref_axis',(0.995806686138499,-0.0350088288095545,0.0845187893148258)) ;
#38600=DIRECTION('center_axis',(0.0914824783325234,0.381078720623582,-0.920005415661252)) ;
#38601=DIRECTION('ref_axis',(0.995806686138499,-0.0350088288095545,0.0845187893148258)) ;
#38602=DIRECTION('center_axis',(0.,0.,1.)) ;
#38603=DIRECTION('ref_axis',(1.,0.,0.)) ;
#38604=DIRECTION('center_axis',(-0.0914824783325234,-0.381078720623582,
0.920005415661252)) ;
#38605=DIRECTION('ref_axis',(0.995806686138499,-0.0350088288095545,0.0845187893148258)) ;
#38606=DIRECTION('center_axis',(0.091482478332531,-0.381078720623592,-0.920005415661248)) ;
#38607=DIRECTION('ref_axis',(0.995806686138498,0.0350088288095584,0.0845187893148324)) ;
#38608=DIRECTION('center_axis',(0.091482478332531,-0.381078720623592,-0.920005415661248)) ;
#38609=DIRECTION('ref_axis',(0.995806686138498,0.0350088288095584,0.0845187893148324)) ;
#38610=DIRECTION('center_axis',(0.,0.,1.)) ;
#38611=DIRECTION('ref_axis',(1.,0.,0.)) ;
#38612=DIRECTION('center_axis',(-0.091482478332531,0.381078720623592,0.920005415661248)) ;
#38613=DIRECTION('ref_axis',(0.995806686138498,0.0350088288095584,0.0845187893148324)) ;
#38614=DIRECTION('center_axis',(0.0914824783325255,-0.920005415661251,-0.381078720623585)) ;
#38615=DIRECTION('ref_axis',(0.995806686138499,0.0845187893148276,0.0350088288095556)) ;
#38616=DIRECTION('center_axis',(0.0914824783325255,-0.920005415661251,-0.381078720623585)) ;
#38617=DIRECTION('ref_axis',(0.995806686138499,0.0845187893148276,0.0350088288095556)) ;
#38618=DIRECTION('center_axis',(0.,0.,1.)) ;
#38619=DIRECTION('ref_axis',(1.,0.,0.)) ;
#38620=DIRECTION('center_axis',(-0.0914824783325255,0.920005415661251,0.381078720623585)) ;
#38621=DIRECTION('ref_axis',(0.995806686138499,0.0845187893148276,0.0350088288095556)) ;
#38622=DIRECTION('center_axis',(0.0914824783325253,-0.920005415661247,0.381078720623595)) ;
#38623=DIRECTION('ref_axis',(0.995806686138499,0.084518789314827,-0.0350088288095565)) ;
#38624=DIRECTION('center_axis',(1.22464679914737E-16,-1.,0.)) ;
#38625=DIRECTION('ref_axis',(-1.,-1.22464679914737E-16,0.)) ;
#38626=DIRECTION('center_axis',(0.0914824783325253,-0.920005415661247,0.381078720623595)) ;
#38627=DIRECTION('ref_axis',(0.995806686138499,0.084518789314827,-0.0350088288095565)) ;
#38628=DIRECTION('center_axis',(0.0914824783325253,-0.920005415661247,0.381078720623595)) ;
#38629=DIRECTION('ref_axis',(0.995806686138499,0.084518789314827,-0.0350088288095565)) ;
#38630=DIRECTION('center_axis',(0.,0.,1.)) ;
#38631=DIRECTION('ref_axis',(-0.0701393346691978,0.997537204184467,0.)) ;
#38632=DIRECTION('center_axis',(-0.0914824783325253,0.920005415661247,-0.381078720623595)) ;
#38633=DIRECTION('ref_axis',(0.995806686138499,0.084518789314827,-0.0350088288095565)) ;
#38634=DIRECTION('center_axis',(0.0914824783325311,-0.381078720623587,0.920005415661249)) ;
#38635=DIRECTION('ref_axis',(0.995806686138498,0.035008828809558,-0.0845187893148328)) ;
#38636=DIRECTION('center_axis',(0.0914824783325311,-0.381078720623587,0.920005415661249)) ;
#38637=DIRECTION('ref_axis',(0.995806686138498,0.035008828809558,-0.0845187893148328)) ;
#38638=DIRECTION('center_axis',(0.,0.,1.)) ;
#38639=DIRECTION('ref_axis',(1.,0.,0.)) ;
#38640=DIRECTION('center_axis',(-0.0914824783325311,0.381078720623587,-0.920005415661249)) ;
#38641=DIRECTION('ref_axis',(0.995806686138498,0.035008828809558,-0.0845187893148328)) ;
#38642=DIRECTION('center_axis',(0.0914824783325242,0.38107872062359,0.920005415661249)) ;
#38643=DIRECTION('ref_axis',(0.995806686138499,-0.0350088288095556,-0.0845187893148262)) ;
#38644=DIRECTION('center_axis',(0.0914824783325242,0.38107872062359,0.920005415661249)) ;
#38645=DIRECTION('ref_axis',(0.995806686138499,-0.0350088288095556,-0.0845187893148262)) ;
#38646=DIRECTION('center_axis',(0.,0.,1.)) ;
#38647=DIRECTION('ref_axis',(1.,0.,0.)) ;
#38648=DIRECTION('center_axis',(-0.0914824783325242,-0.38107872062359,-0.920005415661249)) ;
#38649=DIRECTION('ref_axis',(0.995806686138499,-0.0350088288095556,-0.0845187893148262)) ;
#38650=DIRECTION('center_axis',(0.0914824783325315,0.920005415661255,0.381078720623574)) ;
#38651=DIRECTION('ref_axis',(0.995806686138498,-0.0845187893148336,-0.035008828809557)) ;
#38652=DIRECTION('center_axis',(0.0914824783325315,0.920005415661255,0.381078720623574)) ;
#38653=DIRECTION('ref_axis',(0.995806686138498,-0.0845187893148336,-0.035008828809557)) ;
#38654=DIRECTION('center_axis',(0.,0.,1.)) ;
#38655=DIRECTION('ref_axis',(1.,0.,0.)) ;
#38656=DIRECTION('center_axis',(-0.0914824783325315,-0.920005415661255,
-0.381078720623574)) ;
#38657=DIRECTION('ref_axis',(0.995806686138498,-0.0845187893148336,-0.035008828809557)) ;
#38658=DIRECTION('center_axis',(0.0914824783325258,0.92000541566125,-0.381078720623586)) ;
#38659=DIRECTION('ref_axis',(0.995806686138499,-0.0845187893148279,0.0350088288095559)) ;
#38660=DIRECTION('center_axis',(1.22464679914737E-16,-1.,0.)) ;
#38661=DIRECTION('ref_axis',(-1.,-1.22464679914737E-16,0.)) ;
#38662=DIRECTION('center_axis',(0.0914824783325258,0.92000541566125,-0.381078720623586)) ;
#38663=DIRECTION('ref_axis',(0.995806686138499,-0.0845187893148279,0.0350088288095559)) ;
#38664=DIRECTION('center_axis',(0.0914824783325258,0.92000541566125,-0.381078720623586)) ;
#38665=DIRECTION('ref_axis',(0.995806686138499,-0.0845187893148279,0.0350088288095559)) ;
#38666=DIRECTION('center_axis',(0.,0.,1.)) ;
#38667=DIRECTION('ref_axis',(-0.0701393346692214,-0.997537204184465,0.)) ;
#38668=DIRECTION('center_axis',(-0.0914824783325258,-0.92000541566125,0.381078720623586)) ;
#38669=DIRECTION('ref_axis',(0.995806686138499,-0.0845187893148279,0.0350088288095559)) ;
#38670=DIRECTION('center_axis',(0.0914824783325255,0.381078720623584,-0.920005415661251)) ;
#38671=DIRECTION('ref_axis',(0.995806686138499,-0.0350088288095556,0.0845187893148277)) ;
#38672=DIRECTION('center_axis',(0.0914824783325255,0.381078720623584,-0.920005415661251)) ;
#38673=DIRECTION('ref_axis',(0.995806686138499,-0.0350088288095556,0.0845187893148277)) ;
#38674=DIRECTION('center_axis',(0.,0.,1.)) ;
#38675=DIRECTION('ref_axis',(1.,0.,0.)) ;
#38676=DIRECTION('center_axis',(-0.0914824783325255,-0.381078720623584,
0.920005415661251)) ;
#38677=DIRECTION('ref_axis',(0.995806686138499,-0.0350088288095556,0.0845187893148277)) ;
#38678=DIRECTION('center_axis',(0.0914824783325312,-0.381078720623586,-0.92000541566125)) ;
#38679=DIRECTION('ref_axis',(0.995806686138498,0.0350088288095579,0.0845187893148329)) ;
#38680=DIRECTION('center_axis',(0.0914824783325312,-0.381078720623586,-0.92000541566125)) ;
#38681=DIRECTION('ref_axis',(0.995806686138498,0.0350088288095579,0.0845187893148329)) ;
#38682=DIRECTION('center_axis',(0.,0.,1.)) ;
#38683=DIRECTION('ref_axis',(1.,0.,0.)) ;
#38684=DIRECTION('center_axis',(-0.0914824783325312,0.381078720623586,0.92000541566125)) ;
#38685=DIRECTION('ref_axis',(0.995806686138498,0.0350088288095579,0.0845187893148329)) ;
#38686=DIRECTION('center_axis',(0.0914824783325238,-0.920005415661249,-0.381078720623589)) ;
#38687=DIRECTION('ref_axis',(0.995806686138499,0.0845187893148259,0.0350088288095554)) ;
#38688=DIRECTION('center_axis',(0.0914824783325238,-0.920005415661249,-0.381078720623589)) ;
#38689=DIRECTION('ref_axis',(0.995806686138499,0.0845187893148259,0.0350088288095554)) ;
#38690=DIRECTION('center_axis',(0.,0.,1.)) ;
#38691=DIRECTION('ref_axis',(1.,0.,0.)) ;
#38692=DIRECTION('center_axis',(-0.0914824783325238,0.920005415661249,0.381078720623589)) ;
#38693=DIRECTION('ref_axis',(0.995806686138499,0.0845187893148259,0.0350088288095554)) ;
#38694=DIRECTION('center_axis',(0.0914824783325308,-0.920005415661242,0.381078720623606)) ;
#38695=DIRECTION('ref_axis',(0.995806686138498,0.0845187893148317,-0.0350088288095596)) ;
#38696=DIRECTION('center_axis',(1.22464679914732E-16,-1.,0.)) ;
#38697=DIRECTION('ref_axis',(-1.,-1.22464679914732E-16,0.)) ;
#38698=DIRECTION('center_axis',(0.0914824783325308,-0.920005415661242,0.381078720623606)) ;
#38699=DIRECTION('ref_axis',(0.995806686138498,0.0845187893148317,-0.0350088288095596)) ;
#38700=DIRECTION('center_axis',(0.0914824783325308,-0.920005415661242,0.381078720623606)) ;
#38701=DIRECTION('ref_axis',(0.995806686138498,0.0845187893148317,-0.0350088288095596)) ;
#38702=DIRECTION('center_axis',(0.,0.,1.)) ;
#38703=DIRECTION('ref_axis',(-0.0701393346692214,0.997537204184465,0.)) ;
#38704=DIRECTION('center_axis',(-0.0914824783325308,0.920005415661242,-0.381078720623606)) ;
#38705=DIRECTION('ref_axis',(0.995806686138498,0.0845187893148317,-0.0350088288095596)) ;
#38706=DIRECTION('center_axis',(0.0914824783325257,-0.381078720623582,0.920005415661252)) ;
#38707=DIRECTION('ref_axis',(0.995806686138499,0.0350088288095554,-0.0845187893148279)) ;
#38708=DIRECTION('center_axis',(0.0914824783325257,-0.381078720623582,0.920005415661252)) ;
#38709=DIRECTION('ref_axis',(0.995806686138499,0.0350088288095554,-0.0845187893148279)) ;
#38710=DIRECTION('center_axis',(0.,0.,1.)) ;
#38711=DIRECTION('ref_axis',(1.,0.,0.)) ;
#38712=DIRECTION('center_axis',(-0.0914824783325257,0.381078720623582,-0.920005415661252)) ;
#38713=DIRECTION('ref_axis',(0.995806686138499,0.0350088288095554,-0.0845187893148279)) ;
#38714=DIRECTION('center_axis',(0.0914824783325263,0.381078720623592,0.920005415661247)) ;
#38715=DIRECTION('ref_axis',(0.995806686138499,-0.0350088288095567,-0.0845187893148281)) ;
#38716=DIRECTION('center_axis',(0.0914824783325263,0.381078720623592,0.920005415661247)) ;
#38717=DIRECTION('ref_axis',(0.995806686138499,-0.0350088288095567,-0.0845187893148281)) ;
#38718=DIRECTION('center_axis',(0.,0.,1.)) ;
#38719=DIRECTION('ref_axis',(1.,0.,0.)) ;
#38720=DIRECTION('center_axis',(-0.0914824783325263,-0.381078720623592,
-0.920005415661247)) ;
#38721=DIRECTION('ref_axis',(0.995806686138499,-0.0350088288095567,-0.0845187893148281)) ;
#38722=DIRECTION('center_axis',(0.0914824783325313,0.92000541566125,0.381078720623585)) ;
#38723=DIRECTION('ref_axis',(0.995806686138498,-0.084518789314833,-0.0350088288095579)) ;
#38724=DIRECTION('center_axis',(0.0914824783325313,0.92000541566125,0.381078720623585)) ;
#38725=DIRECTION('ref_axis',(0.995806686138498,-0.084518789314833,-0.0350088288095579)) ;
#38726=DIRECTION('center_axis',(0.,0.,1.)) ;
#38727=DIRECTION('ref_axis',(1.,0.,0.)) ;
#38728=DIRECTION('center_axis',(-0.0914824783325313,-0.92000541566125,-0.381078720623585)) ;
#38729=DIRECTION('ref_axis',(0.995806686138498,-0.084518789314833,-0.0350088288095579)) ;
#38730=DIRECTION('center_axis',(0.091482478332526,0.920005415661255,-0.381078720623575)) ;
#38731=DIRECTION('ref_axis',(0.995806686138499,-0.0845187893148284,0.0350088288095549)) ;
#38732=DIRECTION('center_axis',(1.22464679914737E-16,-1.,0.)) ;
#38733=DIRECTION('ref_axis',(-1.,-1.22464679914737E-16,0.)) ;
#38734=DIRECTION('center_axis',(0.091482478332526,0.920005415661255,-0.381078720623575)) ;
#38735=DIRECTION('ref_axis',(0.995806686138499,-0.0845187893148284,0.0350088288095549)) ;
#38736=DIRECTION('center_axis',(0.091482478332526,0.920005415661255,-0.381078720623575)) ;
#38737=DIRECTION('ref_axis',(0.995806686138499,-0.0845187893148284,0.0350088288095549)) ;
#38738=DIRECTION('center_axis',(0.,0.,1.)) ;
#38739=DIRECTION('ref_axis',(-0.0701393346692214,-0.997537204184465,0.)) ;
#38740=DIRECTION('center_axis',(-0.091482478332526,-0.920005415661255,0.381078720623575)) ;
#38741=DIRECTION('ref_axis',(0.995806686138499,-0.0845187893148284,0.0350088288095549)) ;
#38742=DIRECTION('center_axis',(0.0914824783325291,0.381078720623582,-0.920005415661252)) ;
#38743=DIRECTION('ref_axis',(0.995806686138499,-0.0350088288095568,0.0845187893148311)) ;
#38744=DIRECTION('center_axis',(0.0914824783325291,0.381078720623582,-0.920005415661252)) ;
#38745=DIRECTION('ref_axis',(0.995806686138499,-0.0350088288095568,0.0845187893148311)) ;
#38746=DIRECTION('center_axis',(0.,0.,1.)) ;
#38747=DIRECTION('ref_axis',(1.,0.,0.)) ;
#38748=DIRECTION('center_axis',(-0.0914824783325291,-0.381078720623582,
0.920005415661252)) ;
#38749=DIRECTION('ref_axis',(0.995806686138499,-0.0350088288095568,0.0845187893148311)) ;
#38750=DIRECTION('center_axis',(0.0914824783325252,-0.381078720623591,-0.920005415661248)) ;
#38751=DIRECTION('ref_axis',(0.995806686138499,0.0350088288095562,0.0845187893148272)) ;
#38752=DIRECTION('center_axis',(0.0914824783325252,-0.381078720623591,-0.920005415661248)) ;
#38753=DIRECTION('ref_axis',(0.995806686138499,0.0350088288095562,0.0845187893148272)) ;
#38754=DIRECTION('center_axis',(0.,0.,1.)) ;
#38755=DIRECTION('ref_axis',(1.,0.,0.)) ;
#38756=DIRECTION('center_axis',(-0.0914824783325252,0.381078720623591,0.920005415661248)) ;
#38757=DIRECTION('ref_axis',(0.995806686138499,0.0350088288095562,0.0845187893148272)) ;
#38758=DIRECTION('center_axis',(0.0914824783325255,-0.920005415661251,-0.381078720623585)) ;
#38759=DIRECTION('ref_axis',(0.995806686138499,0.0845187893148276,0.0350088288095556)) ;
#38760=DIRECTION('center_axis',(0.0914824783325255,-0.920005415661251,-0.381078720623585)) ;
#38761=DIRECTION('ref_axis',(0.995806686138499,0.0845187893148276,0.0350088288095556)) ;
#38762=DIRECTION('center_axis',(0.,0.,1.)) ;
#38763=DIRECTION('ref_axis',(1.,0.,0.)) ;
#38764=DIRECTION('center_axis',(-0.0914824783325255,0.920005415661251,0.381078720623585)) ;
#38765=DIRECTION('ref_axis',(0.995806686138499,0.0845187893148276,0.0350088288095556)) ;
#38766=DIRECTION('center_axis',(0.091482478332531,-0.920005415661246,0.381078720623595)) ;
#38767=DIRECTION('ref_axis',(0.995806686138498,0.0845187893148323,-0.0350088288095587)) ;
#38768=DIRECTION('center_axis',(1.22464679914737E-16,-1.,0.)) ;
#38769=DIRECTION('ref_axis',(-1.,-1.22464679914737E-16,0.)) ;
#38770=DIRECTION('center_axis',(0.091482478332531,-0.920005415661246,0.381078720623595)) ;
#38771=DIRECTION('ref_axis',(0.995806686138498,0.0845187893148323,-0.0350088288095587)) ;
#38772=DIRECTION('center_axis',(0.091482478332531,-0.920005415661246,0.381078720623595)) ;
#38773=DIRECTION('ref_axis',(0.995806686138498,0.0845187893148323,-0.0350088288095587)) ;
#38774=DIRECTION('center_axis',(0.,0.,1.)) ;
#38775=DIRECTION('ref_axis',(-0.0701393346692214,0.997537204184465,0.)) ;
#38776=DIRECTION('center_axis',(-0.091482478332531,0.920005415661246,-0.381078720623595)) ;
#38777=DIRECTION('ref_axis',(0.995806686138498,0.0845187893148323,-0.0350088288095587)) ;
#38778=DIRECTION('center_axis',(0.0914824783325244,-0.381078720623583,0.920005415661252)) ;
#38779=DIRECTION('ref_axis',(0.995806686138499,0.0350088288095551,-0.0845187893148267)) ;
#38780=DIRECTION('center_axis',(0.0914824783325244,-0.381078720623583,0.920005415661252)) ;
#38781=DIRECTION('ref_axis',(0.995806686138499,0.0350088288095551,-0.0845187893148267)) ;
#38782=DIRECTION('center_axis',(0.,0.,1.)) ;
#38783=DIRECTION('ref_axis',(1.,0.,0.)) ;
#38784=DIRECTION('center_axis',(-0.0914824783325244,0.381078720623583,-0.920005415661252)) ;
#38785=DIRECTION('ref_axis',(0.995806686138499,0.0350088288095551,-0.0845187893148267)) ;
#38786=DIRECTION('center_axis',(0.0914824783325321,0.381078720623592,0.920005415661247)) ;
#38787=DIRECTION('ref_axis',(0.995806686138498,-0.0350088288095589,-0.0845187893148334)) ;
#38788=DIRECTION('center_axis',(0.0914824783325321,0.381078720623592,0.920005415661247)) ;
#38789=DIRECTION('ref_axis',(0.995806686138498,-0.0350088288095589,-0.0845187893148334)) ;
#38790=DIRECTION('center_axis',(0.,0.,1.)) ;
#38791=DIRECTION('ref_axis',(1.,0.,0.)) ;
#38792=DIRECTION('center_axis',(-0.0914824783325321,-0.381078720623592,
-0.920005415661247)) ;
#38793=DIRECTION('ref_axis',(0.995806686138498,-0.0350088288095589,-0.0845187893148334)) ;
#38794=DIRECTION('center_axis',(0.0914824783325248,0.920005415661252,0.381078720623582)) ;
#38795=DIRECTION('ref_axis',(0.995806686138499,-0.0845187893148271,-0.0350088288095551)) ;
#38796=DIRECTION('center_axis',(0.0914824783325248,0.920005415661252,0.381078720623582)) ;
#38797=DIRECTION('ref_axis',(0.995806686138499,-0.0845187893148271,-0.0350088288095551)) ;
#38798=DIRECTION('center_axis',(0.,0.,1.)) ;
#38799=DIRECTION('ref_axis',(1.,0.,0.)) ;
#38800=DIRECTION('center_axis',(-0.0914824783325248,-0.920005415661252,
-0.381078720623582)) ;
#38801=DIRECTION('ref_axis',(0.995806686138499,-0.0845187893148271,-0.0350088288095551)) ;
#38802=DIRECTION('center_axis',(0.0914824783325258,0.92000541566125,-0.381078720623586)) ;
#38803=DIRECTION('ref_axis',(0.995806686138499,-0.0845187893148278,0.0350088288095558)) ;
#38804=DIRECTION('center_axis',(1.22464679914737E-16,-1.,0.)) ;
#38805=DIRECTION('ref_axis',(-1.,-1.22464679914737E-16,0.)) ;
#38806=DIRECTION('center_axis',(0.0914824783325258,0.92000541566125,-0.381078720623586)) ;
#38807=DIRECTION('ref_axis',(0.995806686138499,-0.0845187893148278,0.0350088288095558)) ;
#38808=DIRECTION('center_axis',(0.0914824783325258,0.92000541566125,-0.381078720623586)) ;
#38809=DIRECTION('ref_axis',(0.995806686138499,-0.0845187893148278,0.0350088288095558)) ;
#38810=DIRECTION('center_axis',(0.,0.,1.)) ;
#38811=DIRECTION('ref_axis',(-0.0701393346692214,-0.997537204184465,0.)) ;
#38812=DIRECTION('center_axis',(-0.0914824783325258,-0.92000541566125,0.381078720623586)) ;
#38813=DIRECTION('ref_axis',(0.995806686138499,-0.0845187893148278,0.0350088288095558)) ;
#38814=DIRECTION('center_axis',(0.0914824783325312,0.381078720623584,-0.92000541566125)) ;
#38815=DIRECTION('ref_axis',(0.995806686138498,-0.0350088288095578,0.084518789314833)) ;
#38816=DIRECTION('center_axis',(0.0914824783325312,0.381078720623584,-0.92000541566125)) ;
#38817=DIRECTION('ref_axis',(0.995806686138498,-0.0350088288095578,0.084518789314833)) ;
#38818=DIRECTION('center_axis',(0.,0.,1.)) ;
#38819=DIRECTION('ref_axis',(1.,0.,0.)) ;
#38820=DIRECTION('center_axis',(-0.0914824783325312,-0.381078720623584,
0.92000541566125)) ;
#38821=DIRECTION('ref_axis',(0.995806686138498,-0.0350088288095578,0.084518789314833)) ;
#38822=DIRECTION('center_axis',(0.0914824783325243,-0.381078720623587,-0.92000541566125)) ;
#38823=DIRECTION('ref_axis',(0.995806686138499,0.0350088288095554,0.0845187893148264)) ;
#38824=DIRECTION('center_axis',(0.0914824783325243,-0.381078720623587,-0.92000541566125)) ;
#38825=DIRECTION('ref_axis',(0.995806686138499,0.0350088288095554,0.0845187893148264)) ;
#38826=DIRECTION('center_axis',(0.,0.,1.)) ;
#38827=DIRECTION('ref_axis',(1.,0.,0.)) ;
#38828=DIRECTION('center_axis',(-0.0914824783325243,0.381078720623587,0.92000541566125)) ;
#38829=DIRECTION('ref_axis',(0.995806686138499,0.0350088288095554,0.0845187893148264)) ;
#38830=DIRECTION('center_axis',(0.0914824783325312,-0.92000541566125,-0.381078720623584)) ;
#38831=DIRECTION('ref_axis',(0.995806686138498,0.0845187893148329,0.0350088288095578)) ;
#38832=DIRECTION('center_axis',(0.0914824783325312,-0.92000541566125,-0.381078720623584)) ;
#38833=DIRECTION('ref_axis',(0.995806686138498,0.0845187893148329,0.0350088288095578)) ;
#38834=DIRECTION('center_axis',(0.,0.,1.)) ;
#38835=DIRECTION('ref_axis',(1.,0.,0.)) ;
#38836=DIRECTION('center_axis',(-0.0914824783325312,0.92000541566125,0.381078720623584)) ;
#38837=DIRECTION('ref_axis',(0.995806686138498,0.0845187893148329,0.0350088288095578)) ;
#38838=DIRECTION('center_axis',(0.0914824783325252,-0.920005415661246,0.381078720623595)) ;
#38839=DIRECTION('ref_axis',(0.995806686138499,0.084518789314827,-0.0350088288095565)) ;
#38840=DIRECTION('center_axis',(1.22464679914736E-16,-1.,0.)) ;
#38841=DIRECTION('ref_axis',(-1.,-1.22464679914736E-16,0.)) ;
#38842=DIRECTION('center_axis',(0.0914824783325252,-0.920005415661246,0.381078720623595)) ;
#38843=DIRECTION('ref_axis',(0.995806686138499,0.084518789314827,-0.0350088288095565)) ;
#38844=DIRECTION('center_axis',(0.0914824783325252,-0.920005415661246,0.381078720623595)) ;
#38845=DIRECTION('ref_axis',(0.995806686138499,0.084518789314827,-0.0350088288095565)) ;
#38846=DIRECTION('center_axis',(0.,0.,1.)) ;
#38847=DIRECTION('ref_axis',(-0.0701393346691978,0.997537204184467,0.)) ;
#38848=DIRECTION('center_axis',(-0.0914824783325252,0.920005415661246,-0.381078720623595)) ;
#38849=DIRECTION('ref_axis',(0.995806686138499,0.084518789314827,-0.0350088288095565)) ;
#38850=DIRECTION('center_axis',(0.0914824783325244,-0.381078720623584,0.920005415661252)) ;
#38851=DIRECTION('ref_axis',(0.995806686138499,0.0350088288095551,-0.0845187893148267)) ;
#38852=DIRECTION('center_axis',(0.0914824783325244,-0.381078720623584,0.920005415661252)) ;
#38853=DIRECTION('ref_axis',(0.995806686138499,0.0350088288095551,-0.0845187893148267)) ;
#38854=DIRECTION('center_axis',(0.,0.,1.)) ;
#38855=DIRECTION('ref_axis',(1.,0.,0.)) ;
#38856=DIRECTION('center_axis',(-0.0914824783325244,0.381078720623584,-0.920005415661252)) ;
#38857=DIRECTION('ref_axis',(0.995806686138499,0.0350088288095551,-0.0845187893148267)) ;
#38858=DIRECTION('center_axis',(0.0914824783325321,0.381078720623592,0.920005415661247)) ;
#38859=DIRECTION('ref_axis',(0.995806686138498,-0.0350088288095588,-0.0845187893148334)) ;
#38860=DIRECTION('center_axis',(0.0914824783325321,0.381078720623592,0.920005415661247)) ;
#38861=DIRECTION('ref_axis',(0.995806686138498,-0.0350088288095588,-0.0845187893148334)) ;
#38862=DIRECTION('center_axis',(0.,0.,1.)) ;
#38863=DIRECTION('ref_axis',(1.,0.,0.)) ;
#38864=DIRECTION('center_axis',(-0.0914824783325321,-0.381078720623592,
-0.920005415661247)) ;
#38865=DIRECTION('ref_axis',(0.995806686138498,-0.0350088288095588,-0.0845187893148334)) ;
#38866=DIRECTION('center_axis',(0.0914824783325256,0.920005415661251,0.381078720623585)) ;
#38867=DIRECTION('ref_axis',(0.995806686138499,-0.0845187893148278,-0.0350088288095557)) ;
#38868=DIRECTION('center_axis',(0.0914824783325256,0.920005415661251,0.381078720623585)) ;
#38869=DIRECTION('ref_axis',(0.995806686138499,-0.0845187893148278,-0.0350088288095557)) ;
#38870=DIRECTION('center_axis',(0.,0.,1.)) ;
#38871=DIRECTION('ref_axis',(1.,0.,0.)) ;
#38872=DIRECTION('center_axis',(-0.0914824783325256,-0.920005415661251,
-0.381078720623585)) ;
#38873=DIRECTION('ref_axis',(0.995806686138499,-0.0845187893148278,-0.0350088288095557)) ;
#38874=DIRECTION('center_axis',(0.0914824783325307,0.920005415661251,-0.381078720623582)) ;
#38875=DIRECTION('ref_axis',(0.995806686138498,-0.0845187893148325,0.0350088288095574)) ;
#38876=DIRECTION('center_axis',(1.22464679914736E-16,-1.,0.)) ;
#38877=DIRECTION('ref_axis',(-1.,-1.22464679914736E-16,0.)) ;
#38878=DIRECTION('center_axis',(0.0914824783325307,0.920005415661251,-0.381078720623582)) ;
#38879=DIRECTION('ref_axis',(0.995806686138498,-0.0845187893148325,0.0350088288095574)) ;
#38880=DIRECTION('center_axis',(0.0914824783325307,0.920005415661251,-0.381078720623582)) ;
#38881=DIRECTION('ref_axis',(0.995806686138498,-0.0845187893148325,0.0350088288095574)) ;
#38882=DIRECTION('center_axis',(0.,0.,1.)) ;
#38883=DIRECTION('ref_axis',(-0.0701393346692214,-0.997537204184465,0.)) ;
#38884=DIRECTION('center_axis',(-0.0914824783325307,-0.920005415661251,
0.381078720623582)) ;
#38885=DIRECTION('ref_axis',(0.995806686138498,-0.0845187893148325,0.0350088288095574)) ;
#38886=DIRECTION('center_axis',(0.0914824783325255,0.381078720623585,-0.920005415661251)) ;
#38887=DIRECTION('ref_axis',(0.995806686138499,-0.0350088288095557,0.0845187893148276)) ;
#38888=DIRECTION('center_axis',(0.0914824783325255,0.381078720623585,-0.920005415661251)) ;
#38889=DIRECTION('ref_axis',(0.995806686138499,-0.0350088288095557,0.0845187893148276)) ;
#38890=DIRECTION('center_axis',(0.,0.,1.)) ;
#38891=DIRECTION('ref_axis',(1.,0.,0.)) ;
#38892=DIRECTION('center_axis',(-0.0914824783325255,-0.381078720623585,
0.920005415661251)) ;
#38893=DIRECTION('ref_axis',(0.995806686138499,-0.0350088288095557,0.0845187893148276)) ;
#38894=DIRECTION('center_axis',(0.0914824783325243,-0.381078720623587,-0.92000541566125)) ;
#38895=DIRECTION('ref_axis',(0.995806686138499,0.0350088288095554,0.0845187893148264)) ;
#38896=DIRECTION('center_axis',(0.0914824783325243,-0.381078720623587,-0.92000541566125)) ;
#38897=DIRECTION('ref_axis',(0.995806686138499,0.0350088288095554,0.0845187893148264)) ;
#38898=DIRECTION('center_axis',(0.,0.,1.)) ;
#38899=DIRECTION('ref_axis',(1.,0.,0.)) ;
#38900=DIRECTION('center_axis',(-0.0914824783325243,0.381078720623587,0.92000541566125)) ;
#38901=DIRECTION('ref_axis',(0.995806686138499,0.0350088288095554,0.0845187893148264)) ;
#38902=DIRECTION('center_axis',(0.0914824783325312,-0.92000541566125,-0.381078720623584)) ;
#38903=DIRECTION('ref_axis',(0.995806686138498,0.0845187893148329,0.0350088288095578)) ;
#38904=DIRECTION('center_axis',(0.0914824783325312,-0.92000541566125,-0.381078720623584)) ;
#38905=DIRECTION('ref_axis',(0.995806686138498,0.0845187893148329,0.0350088288095578)) ;
#38906=DIRECTION('center_axis',(0.,0.,1.)) ;
#38907=DIRECTION('ref_axis',(1.,0.,0.)) ;
#38908=DIRECTION('center_axis',(-0.0914824783325312,0.92000541566125,0.381078720623584)) ;
#38909=DIRECTION('ref_axis',(0.995806686138498,0.0845187893148329,0.0350088288095578)) ;
#38910=DIRECTION('center_axis',(0.0914824783325252,-0.920005415661246,0.381078720623595)) ;
#38911=DIRECTION('ref_axis',(0.995806686138499,0.084518789314827,-0.0350088288095565)) ;
#38912=DIRECTION('center_axis',(1.22464679914736E-16,-1.,0.)) ;
#38913=DIRECTION('ref_axis',(-1.,-1.22464679914736E-16,0.)) ;
#38914=DIRECTION('center_axis',(0.0914824783325252,-0.920005415661246,0.381078720623595)) ;
#38915=DIRECTION('ref_axis',(0.995806686138499,0.084518789314827,-0.0350088288095565)) ;
#38916=DIRECTION('center_axis',(0.0914824783325252,-0.920005415661246,0.381078720623595)) ;
#38917=DIRECTION('ref_axis',(0.995806686138499,0.084518789314827,-0.0350088288095565)) ;
#38918=DIRECTION('center_axis',(0.,0.,1.)) ;
#38919=DIRECTION('ref_axis',(-0.0701393346691978,0.997537204184467,0.)) ;
#38920=DIRECTION('center_axis',(-0.0914824783325252,0.920005415661246,-0.381078720623595)) ;
#38921=DIRECTION('ref_axis',(0.995806686138499,0.084518789314827,-0.0350088288095565)) ;
#38922=DIRECTION('center_axis',(0.0914824783325302,-0.381078720623583,0.920005415661251)) ;
#38923=DIRECTION('ref_axis',(0.995806686138499,0.0350088288095573,-0.084518789314832)) ;
#38924=DIRECTION('center_axis',(0.0914824783325302,-0.381078720623583,0.920005415661251)) ;
#38925=DIRECTION('ref_axis',(0.995806686138499,0.0350088288095573,-0.084518789314832)) ;
#38926=DIRECTION('center_axis',(0.,0.,1.)) ;
#38927=DIRECTION('ref_axis',(1.,0.,0.)) ;
#38928=DIRECTION('center_axis',(-0.0914824783325302,0.381078720623583,-0.920005415661251)) ;
#38929=DIRECTION('ref_axis',(0.995806686138499,0.0350088288095573,-0.084518789314832)) ;
#38930=DIRECTION('center_axis',(0.0914824783325264,0.381078720623592,0.920005415661248)) ;
#38931=DIRECTION('ref_axis',(0.995806686138499,-0.0350088288095566,-0.0845187893148281)) ;
#38932=DIRECTION('center_axis',(0.0914824783325264,0.381078720623592,0.920005415661248)) ;
#38933=DIRECTION('ref_axis',(0.995806686138499,-0.0350088288095566,-0.0845187893148281)) ;
#38934=DIRECTION('center_axis',(0.,0.,1.)) ;
#38935=DIRECTION('ref_axis',(1.,0.,0.)) ;
#38936=DIRECTION('center_axis',(-0.0914824783325264,-0.381078720623592,
-0.920005415661248)) ;
#38937=DIRECTION('ref_axis',(0.995806686138499,-0.0350088288095566,-0.0845187893148281)) ;
#38938=DIRECTION('center_axis',(0.0914824783325249,0.920005415661252,0.381078720623582)) ;
#38939=DIRECTION('ref_axis',(0.995806686138499,-0.0845187893148272,-0.0350088288095551)) ;
#38940=DIRECTION('center_axis',(0.0914824783325249,0.920005415661252,0.381078720623582)) ;
#38941=DIRECTION('ref_axis',(0.995806686138499,-0.0845187893148272,-0.0350088288095551)) ;
#38942=DIRECTION('center_axis',(0.,0.,1.)) ;
#38943=DIRECTION('ref_axis',(1.,0.,0.)) ;
#38944=DIRECTION('center_axis',(-0.0914824783325249,-0.920005415661252,
-0.381078720623582)) ;
#38945=DIRECTION('ref_axis',(0.995806686138499,-0.0845187893148272,-0.0350088288095551)) ;
#38946=DIRECTION('center_axis',(0.0914824783325315,0.92000541566125,-0.381078720623585)) ;
#38947=DIRECTION('ref_axis',(0.995806686138498,-0.0845187893148331,0.035008828809558)) ;
#38948=DIRECTION('center_axis',(1.22464679914737E-16,-1.,0.)) ;
#38949=DIRECTION('ref_axis',(-1.,-1.22464679914737E-16,0.)) ;
#38950=DIRECTION('center_axis',(0.0914824783325315,0.92000541566125,-0.381078720623585)) ;
#38951=DIRECTION('ref_axis',(0.995806686138498,-0.0845187893148331,0.035008828809558)) ;
#38952=DIRECTION('center_axis',(0.0914824783325315,0.92000541566125,-0.381078720623585)) ;
#38953=DIRECTION('ref_axis',(0.995806686138498,-0.0845187893148331,0.035008828809558)) ;
#38954=DIRECTION('center_axis',(0.,0.,1.)) ;
#38955=DIRECTION('ref_axis',(-0.0701393346692214,-0.997537204184465,0.)) ;
#38956=DIRECTION('center_axis',(-0.0914824783325315,-0.92000541566125,0.381078720623585)) ;
#38957=DIRECTION('ref_axis',(0.995806686138498,-0.0845187893148331,0.035008828809558)) ;
#38958=DIRECTION('center_axis',(0.0914824783325255,0.381078720623585,-0.920005415661251)) ;
#38959=DIRECTION('ref_axis',(0.995806686138499,-0.0350088288095557,0.0845187893148276)) ;
#38960=DIRECTION('center_axis',(0.0914824783325255,0.381078720623585,-0.920005415661251)) ;
#38961=DIRECTION('ref_axis',(0.995806686138499,-0.0350088288095557,0.0845187893148276)) ;
#38962=DIRECTION('center_axis',(0.,0.,1.)) ;
#38963=DIRECTION('ref_axis',(1.,0.,0.)) ;
#38964=DIRECTION('center_axis',(-0.0914824783325255,-0.381078720623585,
0.920005415661251)) ;
#38965=DIRECTION('ref_axis',(0.995806686138499,-0.0350088288095557,0.0845187893148276)) ;
#38966=DIRECTION('center_axis',(0.09148247833253,-0.381078720623586,-0.92000541566125)) ;
#38967=DIRECTION('ref_axis',(0.995806686138499,0.0350088288095576,0.0845187893148318)) ;
#38968=DIRECTION('center_axis',(0.09148247833253,-0.381078720623586,-0.92000541566125)) ;
#38969=DIRECTION('ref_axis',(0.995806686138499,0.0350088288095576,0.0845187893148318)) ;
#38970=DIRECTION('center_axis',(0.,0.,1.)) ;
#38971=DIRECTION('ref_axis',(1.,0.,0.)) ;
#38972=DIRECTION('center_axis',(-0.09148247833253,0.381078720623586,0.92000541566125)) ;
#38973=DIRECTION('ref_axis',(0.995806686138499,0.0350088288095576,0.0845187893148318)) ;
#38974=DIRECTION('center_axis',(0.0914824783325255,-0.920005415661251,-0.381078720623585)) ;
#38975=DIRECTION('ref_axis',(0.995806686138499,0.0845187893148277,0.0350088288095557)) ;
#38976=DIRECTION('center_axis',(0.0914824783325255,-0.920005415661251,-0.381078720623585)) ;
#38977=DIRECTION('ref_axis',(0.995806686138499,0.0845187893148277,0.0350088288095557)) ;
#38978=DIRECTION('center_axis',(0.,0.,1.)) ;
#38979=DIRECTION('ref_axis',(1.,0.,0.)) ;
#38980=DIRECTION('center_axis',(-0.0914824783325255,0.920005415661251,0.381078720623585)) ;
#38981=DIRECTION('ref_axis',(0.995806686138499,0.0845187893148277,0.0350088288095557)) ;
#38982=DIRECTION('center_axis',(0.0914824783325252,-0.920005415661246,0.381078720623595)) ;
#38983=DIRECTION('ref_axis',(0.995806686138499,0.084518789314827,-0.0350088288095565)) ;
#38984=DIRECTION('center_axis',(1.22464679914736E-16,-1.,0.)) ;
#38985=DIRECTION('ref_axis',(-1.,-1.22464679914736E-16,0.)) ;
#38986=DIRECTION('center_axis',(0.0914824783325252,-0.920005415661246,0.381078720623595)) ;
#38987=DIRECTION('ref_axis',(0.995806686138499,0.084518789314827,-0.0350088288095565)) ;
#38988=DIRECTION('center_axis',(0.0914824783325252,-0.920005415661246,0.381078720623595)) ;
#38989=DIRECTION('ref_axis',(0.995806686138499,0.084518789314827,-0.0350088288095565)) ;
#38990=DIRECTION('center_axis',(0.,0.,1.)) ;
#38991=DIRECTION('ref_axis',(-0.0701393346692214,0.997537204184465,0.)) ;
#38992=DIRECTION('center_axis',(-0.0914824783325252,0.920005415661246,-0.381078720623595)) ;
#38993=DIRECTION('ref_axis',(0.995806686138499,0.084518789314827,-0.0350088288095565)) ;
#38994=DIRECTION('center_axis',(0.0914824783325311,-0.381078720623588,0.920005415661249)) ;
#38995=DIRECTION('ref_axis',(0.995806686138498,0.0350088288095581,-0.0845187893148327)) ;
#38996=DIRECTION('center_axis',(0.0914824783325311,-0.381078720623588,0.920005415661249)) ;
#38997=DIRECTION('ref_axis',(0.995806686138498,0.0350088288095581,-0.0845187893148327)) ;
#38998=DIRECTION('center_axis',(0.,0.,1.)) ;
#38999=DIRECTION('ref_axis',(1.,0.,0.)) ;
#39000=DIRECTION('center_axis',(-0.0914824783325311,0.381078720623588,-0.920005415661249)) ;
#39001=DIRECTION('ref_axis',(0.995806686138498,0.0350088288095581,-0.0845187893148327)) ;
#39002=DIRECTION('center_axis',(0.0914824783325254,0.381078720623588,0.92000541566125)) ;
#39003=DIRECTION('ref_axis',(0.995806686138499,-0.0350088288095559,-0.0845187893148274)) ;
#39004=DIRECTION('center_axis',(0.0914824783325254,0.381078720623588,0.92000541566125)) ;
#39005=DIRECTION('ref_axis',(0.995806686138499,-0.0350088288095559,-0.0845187893148274)) ;
#39006=DIRECTION('center_axis',(0.,0.,1.)) ;
#39007=DIRECTION('ref_axis',(1.,0.,0.)) ;
#39008=DIRECTION('center_axis',(-0.0914824783325254,-0.381078720623588,
-0.92000541566125)) ;
#39009=DIRECTION('ref_axis',(0.995806686138499,-0.0350088288095559,-0.0845187893148274)) ;
#39010=DIRECTION('center_axis',(0.0914824783325313,0.92000541566125,0.381078720623585)) ;
#39011=DIRECTION('ref_axis',(0.995806686138498,-0.084518789314833,-0.0350088288095579)) ;
#39012=DIRECTION('center_axis',(0.0914824783325313,0.92000541566125,0.381078720623585)) ;
#39013=DIRECTION('ref_axis',(0.995806686138498,-0.084518789314833,-0.0350088288095579)) ;
#39014=DIRECTION('center_axis',(0.,0.,1.)) ;
#39015=DIRECTION('ref_axis',(1.,0.,0.)) ;
#39016=DIRECTION('center_axis',(-0.0914824783325313,-0.92000541566125,-0.381078720623585)) ;
#39017=DIRECTION('ref_axis',(0.995806686138498,-0.084518789314833,-0.0350088288095579)) ;
#39018=DIRECTION('center_axis',(0.091482478332525,0.920005415661252,-0.381078720623582)) ;
#39019=DIRECTION('ref_axis',(0.995806686138499,-0.0845187893148272,0.0350088288095552)) ;
#39020=DIRECTION('center_axis',(1.22464679914736E-16,-1.,0.)) ;
#39021=DIRECTION('ref_axis',(-1.,-1.22464679914736E-16,0.)) ;
#39022=DIRECTION('center_axis',(0.091482478332525,0.920005415661252,-0.381078720623582)) ;
#39023=DIRECTION('ref_axis',(0.995806686138499,-0.0845187893148272,0.0350088288095552)) ;
#39024=DIRECTION('center_axis',(0.091482478332525,0.920005415661252,-0.381078720623582)) ;
#39025=DIRECTION('ref_axis',(0.995806686138499,-0.0845187893148272,0.0350088288095552)) ;
#39026=DIRECTION('center_axis',(0.,0.,1.)) ;
#39027=DIRECTION('ref_axis',(-0.0701393346692214,-0.997537204184465,0.)) ;
#39028=DIRECTION('center_axis',(-0.091482478332525,-0.920005415661252,0.381078720623582)) ;
#39029=DIRECTION('ref_axis',(0.995806686138499,-0.0845187893148272,0.0350088288095552)) ;
#39030=DIRECTION('center_axis',(0.0914824783325255,0.381078720623585,-0.920005415661251)) ;
#39031=DIRECTION('ref_axis',(0.995806686138499,-0.0350088288095557,0.0845187893148276)) ;
#39032=DIRECTION('center_axis',(0.0914824783325255,0.381078720623585,-0.920005415661251)) ;
#39033=DIRECTION('ref_axis',(0.995806686138499,-0.0350088288095557,0.0845187893148276)) ;
#39034=DIRECTION('center_axis',(0.,0.,1.)) ;
#39035=DIRECTION('ref_axis',(1.,0.,0.)) ;
#39036=DIRECTION('center_axis',(-0.0914824783325255,-0.381078720623585,
0.920005415661251)) ;
#39037=DIRECTION('ref_axis',(0.995806686138499,-0.0350088288095557,0.0845187893148276)) ;
#39038=DIRECTION('center_axis',(0.09148247833253,-0.381078720623586,-0.92000541566125)) ;
#39039=DIRECTION('ref_axis',(0.995806686138499,0.0350088288095575,0.0845187893148318)) ;
#39040=DIRECTION('center_axis',(0.09148247833253,-0.381078720623586,-0.92000541566125)) ;
#39041=DIRECTION('ref_axis',(0.995806686138499,0.0350088288095575,0.0845187893148318)) ;
#39042=DIRECTION('center_axis',(0.,0.,1.)) ;
#39043=DIRECTION('ref_axis',(1.,0.,0.)) ;
#39044=DIRECTION('center_axis',(-0.09148247833253,0.381078720623586,0.92000541566125)) ;
#39045=DIRECTION('ref_axis',(0.995806686138499,0.0350088288095575,0.0845187893148318)) ;
#39046=DIRECTION('center_axis',(0.0914824783325255,-0.920005415661251,-0.381078720623585)) ;
#39047=DIRECTION('ref_axis',(0.995806686138499,0.0845187893148277,0.0350088288095557)) ;
#39048=DIRECTION('center_axis',(0.0914824783325255,-0.920005415661251,-0.381078720623585)) ;
#39049=DIRECTION('ref_axis',(0.995806686138499,0.0845187893148277,0.0350088288095557)) ;
#39050=DIRECTION('center_axis',(0.,0.,1.)) ;
#39051=DIRECTION('ref_axis',(1.,0.,0.)) ;
#39052=DIRECTION('center_axis',(-0.0914824783325255,0.920005415661251,0.381078720623585)) ;
#39053=DIRECTION('ref_axis',(0.995806686138499,0.0845187893148277,0.0350088288095557)) ;
#39054=DIRECTION('center_axis',(0.091482478332531,-0.920005415661246,0.381078720623595)) ;
#39055=DIRECTION('ref_axis',(0.995806686138498,0.0845187893148323,-0.0350088288095587)) ;
#39056=DIRECTION('center_axis',(1.22464679914736E-16,-1.,0.)) ;
#39057=DIRECTION('ref_axis',(-1.,-1.22464679914736E-16,0.)) ;
#39058=DIRECTION('center_axis',(0.091482478332531,-0.920005415661246,0.381078720623595)) ;
#39059=DIRECTION('ref_axis',(0.995806686138498,0.0845187893148323,-0.0350088288095587)) ;
#39060=DIRECTION('center_axis',(0.091482478332531,-0.920005415661246,0.381078720623595)) ;
#39061=DIRECTION('ref_axis',(0.995806686138498,0.0845187893148323,-0.0350088288095587)) ;
#39062=DIRECTION('center_axis',(0.,0.,1.)) ;
#39063=DIRECTION('ref_axis',(-0.0701393346692214,0.997537204184465,0.)) ;
#39064=DIRECTION('center_axis',(-0.091482478332531,0.920005415661246,-0.381078720623595)) ;
#39065=DIRECTION('ref_axis',(0.995806686138498,0.0845187893148323,-0.0350088288095587)) ;
#39066=DIRECTION('center_axis',(0.0914824783325254,-0.381078720623588,0.920005415661249)) ;
#39067=DIRECTION('ref_axis',(0.995806686138499,0.0350088288095559,-0.0845187893148274)) ;
#39068=DIRECTION('center_axis',(0.0914824783325254,-0.381078720623588,0.920005415661249)) ;
#39069=DIRECTION('ref_axis',(0.995806686138499,0.0350088288095559,-0.0845187893148274)) ;
#39070=DIRECTION('center_axis',(0.,0.,1.)) ;
#39071=DIRECTION('ref_axis',(1.,0.,0.)) ;
#39072=DIRECTION('center_axis',(-0.0914824783325254,0.381078720623588,-0.920005415661249)) ;
#39073=DIRECTION('ref_axis',(0.995806686138499,0.0350088288095559,-0.0845187893148274)) ;
#39074=DIRECTION('center_axis',(0.0914824783325254,0.381078720623587,0.92000541566125)) ;
#39075=DIRECTION('ref_axis',(0.995806686138499,-0.0350088288095559,-0.0845187893148275)) ;
#39076=DIRECTION('center_axis',(0.0914824783325254,0.381078720623587,0.92000541566125)) ;
#39077=DIRECTION('ref_axis',(0.995806686138499,-0.0350088288095559,-0.0845187893148275)) ;
#39078=DIRECTION('center_axis',(0.,0.,1.)) ;
#39079=DIRECTION('ref_axis',(1.,0.,0.)) ;
#39080=DIRECTION('center_axis',(-0.0914824783325254,-0.381078720623587,
-0.92000541566125)) ;
#39081=DIRECTION('ref_axis',(0.995806686138499,-0.0350088288095559,-0.0845187893148275)) ;
#39082=DIRECTION('center_axis',(0.0914824783325306,0.920005415661252,0.381078720623582)) ;
#39083=DIRECTION('ref_axis',(0.995806686138498,-0.0845187893148324,-0.0350088288095574)) ;
#39084=DIRECTION('center_axis',(0.0914824783325306,0.920005415661252,0.381078720623582)) ;
#39085=DIRECTION('ref_axis',(0.995806686138498,-0.0845187893148324,-0.0350088288095574)) ;
#39086=DIRECTION('center_axis',(0.,0.,1.)) ;
#39087=DIRECTION('ref_axis',(1.,0.,0.)) ;
#39088=DIRECTION('center_axis',(-0.0914824783325306,-0.920005415661252,
-0.381078720623582)) ;
#39089=DIRECTION('ref_axis',(0.995806686138498,-0.0845187893148324,-0.0350088288095574)) ;
#39090=DIRECTION('center_axis',(0.0914824783325257,0.92000541566125,-0.381078720623585)) ;
#39091=DIRECTION('ref_axis',(0.995806686138499,-0.0845187893148278,0.0350088288095558)) ;
#39092=DIRECTION('center_axis',(1.22464679914737E-16,-1.,0.)) ;
#39093=DIRECTION('ref_axis',(-1.,-1.22464679914737E-16,0.)) ;
#39094=DIRECTION('center_axis',(0.0914824783325257,0.92000541566125,-0.381078720623585)) ;
#39095=DIRECTION('ref_axis',(0.995806686138499,-0.0845187893148278,0.0350088288095558)) ;
#39096=DIRECTION('center_axis',(0.0914824783325257,0.92000541566125,-0.381078720623585)) ;
#39097=DIRECTION('ref_axis',(0.995806686138499,-0.0845187893148278,0.0350088288095558)) ;
#39098=DIRECTION('center_axis',(0.,0.,1.)) ;
#39099=DIRECTION('ref_axis',(-0.0701393346692214,-0.997537204184465,0.)) ;
#39100=DIRECTION('center_axis',(-0.0914824783325257,-0.92000541566125,0.381078720623585)) ;
#39101=DIRECTION('ref_axis',(0.995806686138499,-0.0845187893148278,0.0350088288095558)) ;
#39102=DIRECTION('center_axis',(0.0914824783325312,0.381078720623585,-0.92000541566125)) ;
#39103=DIRECTION('ref_axis',(0.995806686138498,-0.0350088288095579,0.0845187893148329)) ;
#39104=DIRECTION('center_axis',(0.0914824783325312,0.381078720623585,-0.92000541566125)) ;
#39105=DIRECTION('ref_axis',(0.995806686138498,-0.0350088288095579,0.0845187893148329)) ;
#39106=DIRECTION('center_axis',(0.,0.,1.)) ;
#39107=DIRECTION('ref_axis',(1.,0.,0.)) ;
#39108=DIRECTION('center_axis',(-0.0914824783325312,-0.381078720623585,
0.92000541566125)) ;
#39109=DIRECTION('ref_axis',(0.995806686138498,-0.0350088288095579,0.0845187893148329)) ;
#39110=DIRECTION('center_axis',(0.0914824783325243,-0.381078720623586,-0.92000541566125)) ;
#39111=DIRECTION('ref_axis',(0.995806686138499,0.0350088288095553,0.0845187893148265)) ;
#39112=DIRECTION('center_axis',(0.0914824783325243,-0.381078720623586,-0.92000541566125)) ;
#39113=DIRECTION('ref_axis',(0.995806686138499,0.0350088288095553,0.0845187893148265)) ;
#39114=DIRECTION('center_axis',(0.,0.,1.)) ;
#39115=DIRECTION('ref_axis',(1.,0.,0.)) ;
#39116=DIRECTION('center_axis',(-0.0914824783325243,0.381078720623586,0.92000541566125)) ;
#39117=DIRECTION('ref_axis',(0.995806686138499,0.0350088288095553,0.0845187893148265)) ;
#39118=DIRECTION('center_axis',(0.0914824783325255,-0.920005415661251,-0.381078720623585)) ;
#39119=DIRECTION('ref_axis',(0.995806686138499,0.0845187893148277,0.0350088288095557)) ;
#39120=DIRECTION('center_axis',(0.0914824783325255,-0.920005415661251,-0.381078720623585)) ;
#39121=DIRECTION('ref_axis',(0.995806686138499,0.0845187893148277,0.0350088288095557)) ;
#39122=DIRECTION('center_axis',(0.,0.,1.)) ;
#39123=DIRECTION('ref_axis',(1.,0.,0.)) ;
#39124=DIRECTION('center_axis',(-0.0914824783325255,0.920005415661251,0.381078720623585)) ;
#39125=DIRECTION('ref_axis',(0.995806686138499,0.0845187893148277,0.0350088288095557)) ;
#39126=DIRECTION('center_axis',(0.0914824783325307,-0.920005415661247,0.381078720623594)) ;
#39127=DIRECTION('ref_axis',(0.995806686138498,0.0845187893148321,-0.0350088288095585)) ;
#39128=DIRECTION('center_axis',(1.22464679914736E-16,-1.,0.)) ;
#39129=DIRECTION('ref_axis',(-1.,-1.22464679914736E-16,0.)) ;
#39130=DIRECTION('center_axis',(0.0914824783325307,-0.920005415661247,0.381078720623594)) ;
#39131=DIRECTION('ref_axis',(0.995806686138498,0.0845187893148321,-0.0350088288095585)) ;
#39132=DIRECTION('center_axis',(0.0914824783325307,-0.920005415661247,0.381078720623594)) ;
#39133=DIRECTION('ref_axis',(0.995806686138498,0.0845187893148321,-0.0350088288095585)) ;
#39134=DIRECTION('center_axis',(0.,0.,1.)) ;
#39135=DIRECTION('ref_axis',(-0.0701393346692214,0.997537204184465,0.)) ;
#39136=DIRECTION('center_axis',(-0.0914824783325307,0.920005415661247,-0.381078720623594)) ;
#39137=DIRECTION('ref_axis',(0.995806686138498,0.0845187893148321,-0.0350088288095585)) ;
#39138=DIRECTION('center_axis',(0.0914824783325255,-0.381078720623585,0.920005415661251)) ;
#39139=DIRECTION('ref_axis',(0.995806686138499,0.0350088288095557,-0.0845187893148276)) ;
#39140=DIRECTION('center_axis',(0.0914824783325255,-0.381078720623585,0.920005415661251)) ;
#39141=DIRECTION('ref_axis',(0.995806686138499,0.0350088288095557,-0.0845187893148276)) ;
#39142=DIRECTION('center_axis',(0.,0.,1.)) ;
#39143=DIRECTION('ref_axis',(1.,0.,0.)) ;
#39144=DIRECTION('center_axis',(-0.0914824783325255,0.381078720623585,-0.920005415661251)) ;
#39145=DIRECTION('ref_axis',(0.995806686138499,0.0350088288095557,-0.0845187893148276)) ;
#39146=DIRECTION('center_axis',(0.0914824783325311,0.381078720623587,0.920005415661249)) ;
#39147=DIRECTION('ref_axis',(0.995806686138498,-0.035008828809558,-0.0845187893148328)) ;
#39148=DIRECTION('center_axis',(0.0914824783325311,0.381078720623587,0.920005415661249)) ;
#39149=DIRECTION('ref_axis',(0.995806686138498,-0.035008828809558,-0.0845187893148328)) ;
#39150=DIRECTION('center_axis',(0.,0.,1.)) ;
#39151=DIRECTION('ref_axis',(1.,0.,0.)) ;
#39152=DIRECTION('center_axis',(-0.0914824783325311,-0.381078720623587,
-0.920005415661249)) ;
#39153=DIRECTION('ref_axis',(0.995806686138498,-0.035008828809558,-0.0845187893148328)) ;
#39154=DIRECTION('center_axis',(0.0914824783325253,0.920005415661251,0.381078720623584)) ;
#39155=DIRECTION('ref_axis',(0.995806686138499,-0.0845187893148275,-0.0350088288095555)) ;
#39156=DIRECTION('center_axis',(0.0914824783325253,0.920005415661251,0.381078720623584)) ;
#39157=DIRECTION('ref_axis',(0.995806686138499,-0.0845187893148275,-0.0350088288095555)) ;
#39158=DIRECTION('center_axis',(0.,0.,1.)) ;
#39159=DIRECTION('ref_axis',(1.,0.,0.)) ;
#39160=DIRECTION('center_axis',(-0.0914824783325253,-0.920005415661251,
-0.381078720623584)) ;
#39161=DIRECTION('ref_axis',(0.995806686138499,-0.0845187893148275,-0.0350088288095555)) ;
#39162=DIRECTION('center_axis',(0.0914824783325253,0.920005415661251,-0.381078720623584)) ;
#39163=DIRECTION('ref_axis',(0.995806686138499,-0.0845187893148275,0.0350088288095555)) ;
#39164=DIRECTION('center_axis',(1.22464679914736E-16,-1.,0.)) ;
#39165=DIRECTION('ref_axis',(-1.,-1.22464679914736E-16,0.)) ;
#39166=DIRECTION('center_axis',(0.0914824783325253,0.920005415661251,-0.381078720623584)) ;
#39167=DIRECTION('ref_axis',(0.995806686138499,-0.0845187893148275,0.0350088288095555)) ;
#39168=DIRECTION('center_axis',(0.0914824783325253,0.920005415661251,-0.381078720623584)) ;
#39169=DIRECTION('ref_axis',(0.995806686138499,-0.0845187893148275,0.0350088288095555)) ;
#39170=DIRECTION('center_axis',(0.,0.,1.)) ;
#39171=DIRECTION('ref_axis',(-0.0701393346692214,-0.997537204184465,0.)) ;
#39172=DIRECTION('center_axis',(-0.0914824783325253,-0.920005415661251,
0.381078720623584)) ;
#39173=DIRECTION('ref_axis',(0.995806686138499,-0.0845187893148275,0.0350088288095555)) ;
#39174=DIRECTION('center_axis',(0.0914824783325312,0.381078720623585,-0.92000541566125)) ;
#39175=DIRECTION('ref_axis',(0.995806686138498,-0.0350088288095579,0.0845187893148329)) ;
#39176=DIRECTION('center_axis',(0.0914824783325312,0.381078720623585,-0.92000541566125)) ;
#39177=DIRECTION('ref_axis',(0.995806686138498,-0.0350088288095579,0.0845187893148329)) ;
#39178=DIRECTION('center_axis',(0.,0.,1.)) ;
#39179=DIRECTION('ref_axis',(1.,0.,0.)) ;
#39180=DIRECTION('center_axis',(-0.0914824783325312,-0.381078720623585,
0.92000541566125)) ;
#39181=DIRECTION('ref_axis',(0.995806686138498,-0.0350088288095579,0.0845187893148329)) ;
#39182=DIRECTION('center_axis',(0.0914824783325254,-0.381078720623587,-0.92000541566125)) ;
#39183=DIRECTION('ref_axis',(0.995806686138499,0.0350088288095559,0.0845187893148275)) ;
#39184=DIRECTION('center_axis',(0.0914824783325254,-0.381078720623587,-0.92000541566125)) ;
#39185=DIRECTION('ref_axis',(0.995806686138499,0.0350088288095559,0.0845187893148275)) ;
#39186=DIRECTION('center_axis',(0.,0.,1.)) ;
#39187=DIRECTION('ref_axis',(1.,0.,0.)) ;
#39188=DIRECTION('center_axis',(-0.0914824783325254,0.381078720623587,0.92000541566125)) ;
#39189=DIRECTION('ref_axis',(0.995806686138499,0.0350088288095559,0.0845187893148275)) ;
#39190=DIRECTION('center_axis',(0.0914824783325306,-0.920005415661247,-0.381078720623593)) ;
#39191=DIRECTION('ref_axis',(0.995806686138498,0.084518789314832,0.0350088288095584)) ;
#39192=DIRECTION('center_axis',(0.0914824783325306,-0.920005415661247,-0.381078720623593)) ;
#39193=DIRECTION('ref_axis',(0.995806686138498,0.084518789314832,0.0350088288095584)) ;
#39194=DIRECTION('center_axis',(0.,0.,1.)) ;
#39195=DIRECTION('ref_axis',(1.,0.,0.)) ;
#39196=DIRECTION('center_axis',(-0.0914824783325306,0.920005415661247,0.381078720623593)) ;
#39197=DIRECTION('ref_axis',(0.995806686138498,0.084518789314832,0.0350088288095584)) ;
#39198=DIRECTION('center_axis',(0.0914824783325249,-0.920005415661247,0.381078720623594)) ;
#39199=DIRECTION('ref_axis',(0.995806686138499,0.0845187893148268,-0.0350088288095563)) ;
#39200=DIRECTION('center_axis',(1.22464679914737E-16,-1.,0.)) ;
#39201=DIRECTION('ref_axis',(-1.,-1.22464679914737E-16,0.)) ;
#39202=DIRECTION('center_axis',(0.0914824783325249,-0.920005415661247,0.381078720623594)) ;
#39203=DIRECTION('ref_axis',(0.995806686138499,0.0845187893148268,-0.0350088288095563)) ;
#39204=DIRECTION('center_axis',(0.0914824783325249,-0.920005415661247,0.381078720623594)) ;
#39205=DIRECTION('ref_axis',(0.995806686138499,0.0845187893148268,-0.0350088288095563)) ;
#39206=DIRECTION('center_axis',(0.,0.,1.)) ;
#39207=DIRECTION('ref_axis',(-0.0701393346692214,0.997537204184465,0.)) ;
#39208=DIRECTION('center_axis',(-0.0914824783325249,0.920005415661247,-0.381078720623594)) ;
#39209=DIRECTION('ref_axis',(0.995806686138499,0.0845187893148268,-0.0350088288095563)) ;
#39210=DIRECTION('center_axis',(0.0914824783325255,-0.381078720623586,0.92000541566125)) ;
#39211=DIRECTION('ref_axis',(0.995806686138499,0.0350088288095557,-0.0845187893148276)) ;
#39212=DIRECTION('center_axis',(0.0914824783325255,-0.381078720623586,0.92000541566125)) ;
#39213=DIRECTION('ref_axis',(0.995806686138499,0.0350088288095557,-0.0845187893148276)) ;
#39214=DIRECTION('center_axis',(0.,0.,1.)) ;
#39215=DIRECTION('ref_axis',(1.,0.,0.)) ;
#39216=DIRECTION('center_axis',(-0.0914824783325255,0.381078720623586,-0.92000541566125)) ;
#39217=DIRECTION('ref_axis',(0.995806686138499,0.0350088288095557,-0.0845187893148276)) ;
#39218=DIRECTION('center_axis',(0.0914824783325311,0.381078720623587,0.920005415661249)) ;
#39219=DIRECTION('ref_axis',(0.995806686138498,-0.035008828809558,-0.0845187893148328)) ;
#39220=DIRECTION('center_axis',(0.0914824783325311,0.381078720623587,0.920005415661249)) ;
#39221=DIRECTION('ref_axis',(0.995806686138498,-0.035008828809558,-0.0845187893148328)) ;
#39222=DIRECTION('center_axis',(0.,0.,1.)) ;
#39223=DIRECTION('ref_axis',(1.,0.,0.)) ;
#39224=DIRECTION('center_axis',(-0.0914824783325311,-0.381078720623587,
-0.920005415661249)) ;
#39225=DIRECTION('ref_axis',(0.995806686138498,-0.035008828809558,-0.0845187893148328)) ;
#39226=DIRECTION('center_axis',(0.0914824783325253,0.920005415661251,0.381078720623584)) ;
#39227=DIRECTION('ref_axis',(0.995806686138499,-0.0845187893148275,-0.0350088288095555)) ;
#39228=DIRECTION('center_axis',(0.0914824783325253,0.920005415661251,0.381078720623584)) ;
#39229=DIRECTION('ref_axis',(0.995806686138499,-0.0845187893148275,-0.0350088288095555)) ;
#39230=DIRECTION('center_axis',(0.,0.,1.)) ;
#39231=DIRECTION('ref_axis',(1.,0.,0.)) ;
#39232=DIRECTION('center_axis',(-0.0914824783325253,-0.920005415661251,
-0.381078720623584)) ;
#39233=DIRECTION('ref_axis',(0.995806686138499,-0.0845187893148275,-0.0350088288095555)) ;
#39234=DIRECTION('center_axis',(0.0914824783325311,0.920005415661251,-0.381078720623584)) ;
#39235=DIRECTION('ref_axis',(0.995806686138498,-0.0845187893148328,0.0350088288095577)) ;
#39236=DIRECTION('center_axis',(1.22464679914737E-16,-1.,0.)) ;
#39237=DIRECTION('ref_axis',(-1.,-1.22464679914737E-16,0.)) ;
#39238=DIRECTION('center_axis',(0.0914824783325311,0.920005415661251,-0.381078720623584)) ;
#39239=DIRECTION('ref_axis',(0.995806686138498,-0.0845187893148328,0.0350088288095577)) ;
#39240=DIRECTION('center_axis',(0.0914824783325311,0.920005415661251,-0.381078720623584)) ;
#39241=DIRECTION('ref_axis',(0.995806686138498,-0.0845187893148328,0.0350088288095577)) ;
#39242=DIRECTION('center_axis',(0.,0.,1.)) ;
#39243=DIRECTION('ref_axis',(-0.0701393346692214,-0.997537204184465,0.)) ;
#39244=DIRECTION('center_axis',(-0.0914824783325311,-0.920005415661251,
0.381078720623584)) ;
#39245=DIRECTION('ref_axis',(0.995806686138498,-0.0845187893148328,0.0350088288095577)) ;
#39246=DIRECTION('center_axis',(0.0914824783325255,0.381078720623586,-0.92000541566125)) ;
#39247=DIRECTION('ref_axis',(0.995806686138499,-0.0350088288095557,0.0845187893148276)) ;
#39248=DIRECTION('center_axis',(0.0914824783325255,0.381078720623586,-0.92000541566125)) ;
#39249=DIRECTION('ref_axis',(0.995806686138499,-0.0350088288095557,0.0845187893148276)) ;
#39250=DIRECTION('center_axis',(0.,0.,1.)) ;
#39251=DIRECTION('ref_axis',(1.,0.,0.)) ;
#39252=DIRECTION('center_axis',(-0.0914824783325255,-0.381078720623586,
0.92000541566125)) ;
#39253=DIRECTION('ref_axis',(0.995806686138499,-0.0350088288095557,0.0845187893148276)) ;
#39254=DIRECTION('center_axis',(0.0914824783325254,-0.381078720623587,-0.92000541566125)) ;
#39255=DIRECTION('ref_axis',(0.995806686138499,0.0350088288095558,0.0845187893148275)) ;
#39256=DIRECTION('center_axis',(0.0914824783325254,-0.381078720623587,-0.92000541566125)) ;
#39257=DIRECTION('ref_axis',(0.995806686138499,0.0350088288095558,0.0845187893148275)) ;
#39258=DIRECTION('center_axis',(0.,0.,1.)) ;
#39259=DIRECTION('ref_axis',(1.,0.,0.)) ;
#39260=DIRECTION('center_axis',(-0.0914824783325254,0.381078720623587,0.92000541566125)) ;
#39261=DIRECTION('ref_axis',(0.995806686138499,0.0350088288095558,0.0845187893148275)) ;
#39262=DIRECTION('center_axis',(0.0914824783325306,-0.920005415661247,-0.381078720623593)) ;
#39263=DIRECTION('ref_axis',(0.995806686138498,0.084518789314832,0.0350088288095584)) ;
#39264=DIRECTION('center_axis',(0.0914824783325306,-0.920005415661247,-0.381078720623593)) ;
#39265=DIRECTION('ref_axis',(0.995806686138498,0.084518789314832,0.0350088288095584)) ;
#39266=DIRECTION('center_axis',(0.,0.,1.)) ;
#39267=DIRECTION('ref_axis',(1.,0.,0.)) ;
#39268=DIRECTION('center_axis',(-0.0914824783325306,0.920005415661247,0.381078720623593)) ;
#39269=DIRECTION('ref_axis',(0.995806686138498,0.084518789314832,0.0350088288095584)) ;
#39270=DIRECTION('center_axis',(0.0914824783325249,-0.920005415661247,0.381078720623594)) ;
#39271=DIRECTION('ref_axis',(0.995806686138499,0.0845187893148267,-0.0350088288095562)) ;
#39272=DIRECTION('center_axis',(1.22464679914737E-16,-1.,0.)) ;
#39273=DIRECTION('ref_axis',(-1.,-1.22464679914737E-16,0.)) ;
#39274=DIRECTION('center_axis',(0.0914824783325249,-0.920005415661247,0.381078720623594)) ;
#39275=DIRECTION('ref_axis',(0.995806686138499,0.0845187893148267,-0.0350088288095562)) ;
#39276=DIRECTION('center_axis',(0.0914824783325249,-0.920005415661247,0.381078720623594)) ;
#39277=DIRECTION('ref_axis',(0.995806686138499,0.0845187893148267,-0.0350088288095562)) ;
#39278=DIRECTION('center_axis',(0.,0.,1.)) ;
#39279=DIRECTION('ref_axis',(-0.0701393346692214,0.997537204184465,0.)) ;
#39280=DIRECTION('center_axis',(-0.0914824783325249,0.920005415661247,-0.381078720623594)) ;
#39281=DIRECTION('ref_axis',(0.995806686138499,0.0845187893148267,-0.0350088288095562)) ;
#39282=DIRECTION('center_axis',(0.0914824783325312,-0.381078720623586,0.92000541566125)) ;
#39283=DIRECTION('ref_axis',(0.995806686138498,0.0350088288095579,-0.0845187893148329)) ;
#39284=DIRECTION('center_axis',(0.0914824783325312,-0.381078720623586,0.92000541566125)) ;
#39285=DIRECTION('ref_axis',(0.995806686138498,0.0350088288095579,-0.0845187893148329)) ;
#39286=DIRECTION('center_axis',(0.,0.,1.)) ;
#39287=DIRECTION('ref_axis',(1.,0.,0.)) ;
#39288=DIRECTION('center_axis',(-0.0914824783325312,0.381078720623586,-0.92000541566125)) ;
#39289=DIRECTION('ref_axis',(0.995806686138498,0.0350088288095579,-0.0845187893148329)) ;
#39290=DIRECTION('center_axis',(0.0914824783325254,0.381078720623587,0.92000541566125)) ;
#39291=DIRECTION('ref_axis',(0.995806686138499,-0.0350088288095558,-0.0845187893148275)) ;
#39292=DIRECTION('center_axis',(0.0914824783325254,0.381078720623587,0.92000541566125)) ;
#39293=DIRECTION('ref_axis',(0.995806686138499,-0.0350088288095558,-0.0845187893148275)) ;
#39294=DIRECTION('center_axis',(0.,0.,1.)) ;
#39295=DIRECTION('ref_axis',(1.,0.,0.)) ;
#39296=DIRECTION('center_axis',(-0.0914824783325254,-0.381078720623587,
-0.92000541566125)) ;
#39297=DIRECTION('ref_axis',(0.995806686138499,-0.0350088288095558,-0.0845187893148275)) ;
#39298=DIRECTION('center_axis',(0.0914824783325253,0.920005415661251,0.381078720623584)) ;
#39299=DIRECTION('ref_axis',(0.995806686138499,-0.0845187893148275,-0.0350088288095555)) ;
#39300=DIRECTION('center_axis',(0.0914824783325253,0.920005415661251,0.381078720623584)) ;
#39301=DIRECTION('ref_axis',(0.995806686138499,-0.0845187893148275,-0.0350088288095555)) ;
#39302=DIRECTION('center_axis',(0.,0.,1.)) ;
#39303=DIRECTION('ref_axis',(1.,0.,0.)) ;
#39304=DIRECTION('center_axis',(-0.0914824783325253,-0.920005415661251,
-0.381078720623584)) ;
#39305=DIRECTION('ref_axis',(0.995806686138499,-0.0845187893148275,-0.0350088288095555)) ;
#39306=DIRECTION('center_axis',(0.091482478332531,0.920005415661251,-0.381078720623584)) ;
#39307=DIRECTION('ref_axis',(0.995806686138498,-0.0845187893148328,0.0350088288095577)) ;
#39308=DIRECTION('center_axis',(1.22464679914737E-16,-1.,0.)) ;
#39309=DIRECTION('ref_axis',(-1.,-1.22464679914737E-16,0.)) ;
#39310=DIRECTION('center_axis',(0.091482478332531,0.920005415661251,-0.381078720623584)) ;
#39311=DIRECTION('ref_axis',(0.995806686138498,-0.0845187893148328,0.0350088288095577)) ;
#39312=DIRECTION('center_axis',(0.091482478332531,0.920005415661251,-0.381078720623584)) ;
#39313=DIRECTION('ref_axis',(0.995806686138498,-0.0845187893148328,0.0350088288095577)) ;
#39314=DIRECTION('center_axis',(0.,0.,1.)) ;
#39315=DIRECTION('ref_axis',(-0.0701393346692214,-0.997537204184465,0.)) ;
#39316=DIRECTION('center_axis',(-0.091482478332531,-0.920005415661251,0.381078720623584)) ;
#39317=DIRECTION('ref_axis',(0.995806686138498,-0.0845187893148328,0.0350088288095577)) ;
#39318=DIRECTION('center_axis',(0.0914824783325255,0.381078720623586,-0.92000541566125)) ;
#39319=DIRECTION('ref_axis',(0.995806686138499,-0.0350088288095557,0.0845187893148276)) ;
#39320=DIRECTION('center_axis',(0.0914824783325255,0.381078720623586,-0.92000541566125)) ;
#39321=DIRECTION('ref_axis',(0.995806686138499,-0.0350088288095557,0.0845187893148276)) ;
#39322=DIRECTION('center_axis',(0.,0.,1.)) ;
#39323=DIRECTION('ref_axis',(1.,0.,0.)) ;
#39324=DIRECTION('center_axis',(-0.0914824783325255,-0.381078720623586,
0.92000541566125)) ;
#39325=DIRECTION('ref_axis',(0.995806686138499,-0.0350088288095557,0.0845187893148276)) ;
#39326=DIRECTION('center_axis',(0.0914824783325311,-0.381078720623587,-0.920005415661249)) ;
#39327=DIRECTION('ref_axis',(0.995806686138498,0.035008828809558,0.0845187893148328)) ;
#39328=DIRECTION('center_axis',(0.0914824783325311,-0.381078720623587,-0.920005415661249)) ;
#39329=DIRECTION('ref_axis',(0.995806686138498,0.035008828809558,0.0845187893148328)) ;
#39330=DIRECTION('center_axis',(0.,0.,1.)) ;
#39331=DIRECTION('ref_axis',(1.,0.,0.)) ;
#39332=DIRECTION('center_axis',(-0.0914824783325311,0.381078720623587,0.920005415661249)) ;
#39333=DIRECTION('ref_axis',(0.995806686138498,0.035008828809558,0.0845187893148328)) ;
#39334=DIRECTION('center_axis',(0.0914824783325249,-0.920005415661247,-0.381078720623594)) ;
#39335=DIRECTION('ref_axis',(0.995806686138499,0.0845187893148267,0.0350088288095562)) ;
#39336=DIRECTION('center_axis',(0.0914824783325249,-0.920005415661247,-0.381078720623594)) ;
#39337=DIRECTION('ref_axis',(0.995806686138499,0.0845187893148267,0.0350088288095562)) ;
#39338=DIRECTION('center_axis',(0.,0.,1.)) ;
#39339=DIRECTION('ref_axis',(1.,0.,0.)) ;
#39340=DIRECTION('center_axis',(-0.0914824783325249,0.920005415661247,0.381078720623594)) ;
#39341=DIRECTION('ref_axis',(0.995806686138499,0.0845187893148267,0.0350088288095562)) ;
#39342=DIRECTION('center_axis',(0.0914824783325249,-0.920005415661247,0.381078720623594)) ;
#39343=DIRECTION('ref_axis',(0.995806686138499,0.0845187893148268,-0.0350088288095563)) ;
#39344=DIRECTION('center_axis',(1.22464679914736E-16,-1.,0.)) ;
#39345=DIRECTION('ref_axis',(-1.,-1.22464679914736E-16,0.)) ;
#39346=DIRECTION('center_axis',(0.0914824783325249,-0.920005415661247,0.381078720623594)) ;
#39347=DIRECTION('ref_axis',(0.995806686138499,0.0845187893148268,-0.0350088288095563)) ;
#39348=DIRECTION('center_axis',(0.0914824783325249,-0.920005415661247,0.381078720623594)) ;
#39349=DIRECTION('ref_axis',(0.995806686138499,0.0845187893148268,-0.0350088288095563)) ;
#39350=DIRECTION('center_axis',(0.,0.,1.)) ;
#39351=DIRECTION('ref_axis',(-0.0701393346691978,0.997537204184467,0.)) ;
#39352=DIRECTION('center_axis',(-0.0914824783325249,0.920005415661247,-0.381078720623594)) ;
#39353=DIRECTION('ref_axis',(0.995806686138499,0.0845187893148268,-0.0350088288095563)) ;
#39354=DIRECTION('center_axis',(0.0914824783325312,-0.381078720623586,0.92000541566125)) ;
#39355=DIRECTION('ref_axis',(0.995806686138498,0.035008828809558,-0.0845187893148329)) ;
#39356=DIRECTION('center_axis',(0.0914824783325312,-0.381078720623586,0.92000541566125)) ;
#39357=DIRECTION('ref_axis',(0.995806686138498,0.035008828809558,-0.0845187893148329)) ;
#39358=DIRECTION('center_axis',(0.,0.,1.)) ;
#39359=DIRECTION('ref_axis',(1.,0.,0.)) ;
#39360=DIRECTION('center_axis',(-0.0914824783325312,0.381078720623586,-0.92000541566125)) ;
#39361=DIRECTION('ref_axis',(0.995806686138498,0.035008828809558,-0.0845187893148329)) ;
#39362=DIRECTION('center_axis',(0.0914824783325254,0.381078720623587,0.92000541566125)) ;
#39363=DIRECTION('ref_axis',(0.995806686138499,-0.0350088288095558,-0.0845187893148275)) ;
#39364=DIRECTION('center_axis',(0.0914824783325254,0.381078720623587,0.92000541566125)) ;
#39365=DIRECTION('ref_axis',(0.995806686138499,-0.0350088288095558,-0.0845187893148275)) ;
#39366=DIRECTION('center_axis',(0.,0.,1.)) ;
#39367=DIRECTION('ref_axis',(1.,0.,0.)) ;
#39368=DIRECTION('center_axis',(-0.0914824783325254,-0.381078720623587,
-0.92000541566125)) ;
#39369=DIRECTION('ref_axis',(0.995806686138499,-0.0350088288095558,-0.0845187893148275)) ;
#39370=DIRECTION('center_axis',(0.091482478332531,0.920005415661251,0.381078720623584)) ;
#39371=DIRECTION('ref_axis',(0.995806686138498,-0.0845187893148328,-0.0350088288095577)) ;
#39372=DIRECTION('center_axis',(0.091482478332531,0.920005415661251,0.381078720623584)) ;
#39373=DIRECTION('ref_axis',(0.995806686138498,-0.0845187893148328,-0.0350088288095577)) ;
#39374=DIRECTION('center_axis',(0.,0.,1.)) ;
#39375=DIRECTION('ref_axis',(1.,0.,0.)) ;
#39376=DIRECTION('center_axis',(-0.091482478332531,-0.920005415661251,-0.381078720623584)) ;
#39377=DIRECTION('ref_axis',(0.995806686138498,-0.0845187893148328,-0.0350088288095577)) ;
#39378=DIRECTION('center_axis',(0.0914824783325253,0.920005415661251,-0.381078720623584)) ;
#39379=DIRECTION('ref_axis',(0.995806686138499,-0.0845187893148275,0.0350088288095555)) ;
#39380=DIRECTION('center_axis',(1.22464679914736E-16,-1.,0.)) ;
#39381=DIRECTION('ref_axis',(-1.,-1.22464679914736E-16,0.)) ;
#39382=DIRECTION('center_axis',(0.0914824783325253,0.920005415661251,-0.381078720623584)) ;
#39383=DIRECTION('ref_axis',(0.995806686138499,-0.0845187893148275,0.0350088288095555)) ;
#39384=DIRECTION('center_axis',(0.0914824783325253,0.920005415661251,-0.381078720623584)) ;
#39385=DIRECTION('ref_axis',(0.995806686138499,-0.0845187893148275,0.0350088288095555)) ;
#39386=DIRECTION('center_axis',(0.,0.,1.)) ;
#39387=DIRECTION('ref_axis',(-0.0701393346692214,-0.997537204184465,0.)) ;
#39388=DIRECTION('center_axis',(-0.0914824783325253,-0.920005415661251,
0.381078720623584)) ;
#39389=DIRECTION('ref_axis',(0.995806686138499,-0.0845187893148275,0.0350088288095555)) ;
#39390=DIRECTION('center_axis',(0.0914824783325255,0.381078720623586,-0.92000541566125)) ;
#39391=DIRECTION('ref_axis',(0.995806686138499,-0.0350088288095558,0.0845187893148276)) ;
#39392=DIRECTION('center_axis',(0.0914824783325255,0.381078720623586,-0.92000541566125)) ;
#39393=DIRECTION('ref_axis',(0.995806686138499,-0.0350088288095558,0.0845187893148276)) ;
#39394=DIRECTION('center_axis',(0.,0.,1.)) ;
#39395=DIRECTION('ref_axis',(1.,0.,0.)) ;
#39396=DIRECTION('center_axis',(-0.0914824783325255,-0.381078720623586,
0.92000541566125)) ;
#39397=DIRECTION('ref_axis',(0.995806686138499,-0.0350088288095558,0.0845187893148276)) ;
#39398=DIRECTION('center_axis',(0.0914824783325311,-0.381078720623587,-0.920005415661249)) ;
#39399=DIRECTION('ref_axis',(0.995806686138498,0.035008828809558,0.0845187893148328)) ;
#39400=DIRECTION('center_axis',(0.0914824783325311,-0.381078720623587,-0.920005415661249)) ;
#39401=DIRECTION('ref_axis',(0.995806686138498,0.035008828809558,0.0845187893148328)) ;
#39402=DIRECTION('center_axis',(0.,0.,1.)) ;
#39403=DIRECTION('ref_axis',(1.,0.,0.)) ;
#39404=DIRECTION('center_axis',(-0.0914824783325311,0.381078720623587,0.920005415661249)) ;
#39405=DIRECTION('ref_axis',(0.995806686138498,0.035008828809558,0.0845187893148328)) ;
#39406=DIRECTION('center_axis',(0.091482478332525,-0.920005415661247,-0.381078720623594)) ;
#39407=DIRECTION('ref_axis',(0.995806686138499,0.0845187893148268,0.0350088288095563)) ;
#39408=DIRECTION('center_axis',(0.091482478332525,-0.920005415661247,-0.381078720623594)) ;
#39409=DIRECTION('ref_axis',(0.995806686138499,0.0845187893148268,0.0350088288095563)) ;
#39410=DIRECTION('center_axis',(0.,0.,1.)) ;
#39411=DIRECTION('ref_axis',(1.,0.,0.)) ;
#39412=DIRECTION('center_axis',(-0.091482478332525,0.920005415661247,0.381078720623594)) ;
#39413=DIRECTION('ref_axis',(0.995806686138499,0.0845187893148268,0.0350088288095563)) ;
#39414=DIRECTION('center_axis',(0.0914824783325307,-0.920005415661246,0.381078720623594)) ;
#39415=DIRECTION('ref_axis',(0.995806686138498,0.0845187893148321,-0.0350088288095585)) ;
#39416=DIRECTION('center_axis',(1.22464679914737E-16,-1.,0.)) ;
#39417=DIRECTION('ref_axis',(-1.,-1.22464679914737E-16,0.)) ;
#39418=DIRECTION('center_axis',(0.0914824783325307,-0.920005415661246,0.381078720623594)) ;
#39419=DIRECTION('ref_axis',(0.995806686138498,0.0845187893148321,-0.0350088288095585)) ;
#39420=DIRECTION('center_axis',(0.0914824783325307,-0.920005415661246,0.381078720623594)) ;
#39421=DIRECTION('ref_axis',(0.995806686138498,0.0845187893148321,-0.0350088288095585)) ;
#39422=DIRECTION('center_axis',(0.,0.,1.)) ;
#39423=DIRECTION('ref_axis',(-0.0701393346692214,0.997537204184465,0.)) ;
#39424=DIRECTION('center_axis',(-0.0914824783325307,0.920005415661246,-0.381078720623594)) ;
#39425=DIRECTION('ref_axis',(0.995806686138498,0.0845187893148321,-0.0350088288095585)) ;
#39426=DIRECTION('center_axis',(0.0914824783325254,-0.381078720623587,0.92000541566125)) ;
#39427=DIRECTION('ref_axis',(0.995806686138499,0.0350088288095558,-0.0845187893148275)) ;
#39428=DIRECTION('center_axis',(0.0914824783325254,-0.381078720623587,0.92000541566125)) ;
#39429=DIRECTION('ref_axis',(0.995806686138499,0.0350088288095558,-0.0845187893148275)) ;
#39430=DIRECTION('center_axis',(0.,0.,1.)) ;
#39431=DIRECTION('ref_axis',(1.,0.,0.)) ;
#39432=DIRECTION('center_axis',(-0.0914824783325254,0.381078720623587,-0.92000541566125)) ;
#39433=DIRECTION('ref_axis',(0.995806686138499,0.0350088288095558,-0.0845187893148275)) ;
#39434=DIRECTION('center_axis',(0.0914824783325254,0.381078720623587,0.92000541566125)) ;
#39435=DIRECTION('ref_axis',(0.995806686138499,-0.0350088288095559,-0.0845187893148275)) ;
#39436=DIRECTION('center_axis',(0.0914824783325254,0.381078720623587,0.92000541566125)) ;
#39437=DIRECTION('ref_axis',(0.995806686138499,-0.0350088288095559,-0.0845187893148275)) ;
#39438=DIRECTION('center_axis',(0.,0.,1.)) ;
#39439=DIRECTION('ref_axis',(1.,0.,0.)) ;
#39440=DIRECTION('center_axis',(-0.0914824783325254,-0.381078720623587,
-0.92000541566125)) ;
#39441=DIRECTION('ref_axis',(0.995806686138499,-0.0350088288095559,-0.0845187893148275)) ;
#39442=DIRECTION('center_axis',(0.0914824783325311,0.920005415661251,0.381078720623584)) ;
#39443=DIRECTION('ref_axis',(0.995806686138498,-0.0845187893148328,-0.0350088288095577)) ;
#39444=DIRECTION('center_axis',(0.0914824783325311,0.920005415661251,0.381078720623584)) ;
#39445=DIRECTION('ref_axis',(0.995806686138498,-0.0845187893148328,-0.0350088288095577)) ;
#39446=DIRECTION('center_axis',(0.,0.,1.)) ;
#39447=DIRECTION('ref_axis',(1.,0.,0.)) ;
#39448=DIRECTION('center_axis',(-0.0914824783325311,-0.920005415661251,
-0.381078720623584)) ;
#39449=DIRECTION('ref_axis',(0.995806686138498,-0.0845187893148328,-0.0350088288095577)) ;
#39450=DIRECTION('center_axis',(0.0914824783325254,0.920005415661251,-0.381078720623584)) ;
#39451=DIRECTION('ref_axis',(0.995806686138499,-0.0845187893148275,0.0350088288095555)) ;
#39452=DIRECTION('center_axis',(1.22464679914737E-16,-1.,0.)) ;
#39453=DIRECTION('ref_axis',(-1.,-1.22464679914737E-16,0.)) ;
#39454=DIRECTION('center_axis',(0.0914824783325254,0.920005415661251,-0.381078720623584)) ;
#39455=DIRECTION('ref_axis',(0.995806686138499,-0.0845187893148275,0.0350088288095555)) ;
#39456=DIRECTION('center_axis',(0.0914824783325254,0.920005415661251,-0.381078720623584)) ;
#39457=DIRECTION('ref_axis',(0.995806686138499,-0.0845187893148275,0.0350088288095555)) ;
#39458=DIRECTION('center_axis',(0.,0.,1.)) ;
#39459=DIRECTION('ref_axis',(-0.0701393346692214,-0.997537204184465,0.)) ;
#39460=DIRECTION('center_axis',(-0.0914824783325254,-0.920005415661251,
0.381078720623584)) ;
#39461=DIRECTION('ref_axis',(0.995806686138499,-0.0845187893148275,0.0350088288095555)) ;
#39462=DIRECTION('center_axis',(0.0914824783325311,0.381078720623587,-0.920005415661249)) ;
#39463=DIRECTION('ref_axis',(0.995806686138498,-0.035008828809558,0.0845187893148328)) ;
#39464=DIRECTION('center_axis',(0.0914824783325311,0.381078720623587,-0.920005415661249)) ;
#39465=DIRECTION('ref_axis',(0.995806686138498,-0.035008828809558,0.0845187893148328)) ;
#39466=DIRECTION('center_axis',(0.,0.,1.)) ;
#39467=DIRECTION('ref_axis',(1.,0.,0.)) ;
#39468=DIRECTION('center_axis',(-0.0914824783325311,-0.381078720623587,
0.920005415661249)) ;
#39469=DIRECTION('ref_axis',(0.995806686138498,-0.035008828809558,0.0845187893148328)) ;
#39470=DIRECTION('center_axis',(0.0914824783325254,-0.381078720623587,-0.92000541566125)) ;
#39471=DIRECTION('ref_axis',(0.995806686138499,0.0350088288095559,0.0845187893148275)) ;
#39472=DIRECTION('center_axis',(0.0914824783325254,-0.381078720623587,-0.92000541566125)) ;
#39473=DIRECTION('ref_axis',(0.995806686138499,0.0350088288095559,0.0845187893148275)) ;
#39474=DIRECTION('center_axis',(0.,0.,1.)) ;
#39475=DIRECTION('ref_axis',(1.,0.,0.)) ;
#39476=DIRECTION('center_axis',(-0.0914824783325254,0.381078720623587,0.92000541566125)) ;
#39477=DIRECTION('ref_axis',(0.995806686138499,0.0350088288095559,0.0845187893148275)) ;
#39478=DIRECTION('center_axis',(0.091482478332525,-0.920005415661247,-0.381078720623594)) ;
#39479=DIRECTION('ref_axis',(0.995806686138499,0.0845187893148268,0.0350088288095563)) ;
#39480=DIRECTION('center_axis',(0.091482478332525,-0.920005415661247,-0.381078720623594)) ;
#39481=DIRECTION('ref_axis',(0.995806686138499,0.0845187893148268,0.0350088288095563)) ;
#39482=DIRECTION('center_axis',(0.091482478332531,-0.920005415661246,0.381078720623595)) ;
#39483=DIRECTION('ref_axis',(-0.692805212515615,-0.333687184544024,-0.639275997032796)) ;
#39484=DIRECTION('center_axis',(-0.0989489060815955,0.703636665469238,-0.703636665469181)) ;
#39485=DIRECTION('ref_axis',(-3.31831546202878E-14,0.707106781186516,0.707106781186579)) ;
#39486=DIRECTION('center_axis',(0.0914824783325255,-0.381078720623586,0.92000541566125)) ;
#39487=DIRECTION('ref_axis',(-0.839445610209476,-0.526507333754943,-0.134614616599765)) ;
#39488=DIRECTION('center_axis',(-0.0989489060816109,0.,-0.995092515289535)) ;
#39489=DIRECTION('ref_axis',(1.40655517650999E-14,1.,-1.41604447882206E-15)) ;
#39490=DIRECTION('center_axis',(0.0914824783325241,0.381078720623591,0.920005415661248)) ;
#39491=DIRECTION('ref_axis',(0.995806686138499,-0.0350088288095557,-0.0845187893148261)) ;
#39492=DIRECTION('',(-0.0914824783325241,-0.381078720623591,-0.920005415661248)) ;
#39493=DIRECTION('center_axis',(-0.0989489060815947,-0.703636665469224,
-0.703636665469195)) ;
#39494=DIRECTION('ref_axis',(-2.3378433245451E-14,0.707106781186535,-0.707106781186561)) ;
#39495=DIRECTION('center_axis',(-0.0989489060815947,-0.703636665469224,
-0.703636665469195)) ;
#39496=DIRECTION('ref_axis',(-2.3378433245451E-14,0.707106781186535,-0.707106781186561)) ;
#39497=DIRECTION('center_axis',(0.0914824783325315,0.920005415661255,0.381078720623574)) ;
#39498=DIRECTION('ref_axis',(0.995806686138498,-0.0845187893148336,-0.035008828809557)) ;
#39499=DIRECTION('',(-0.0914824783325315,-0.920005415661255,-0.381078720623574)) ;
#39500=DIRECTION('center_axis',(-0.0989489060816085,-0.995092515289535,
6.08202833592793E-14)) ;
#39501=DIRECTION('ref_axis',(-1.23494582202129E-14,-5.9918929754176E-14,
-1.)) ;
#39502=DIRECTION('center_axis',(-0.0989489060816085,-0.995092515289535,
6.08202833592793E-14)) ;
#39503=DIRECTION('ref_axis',(-1.23494582202129E-14,-5.9918929754176E-14,
-1.)) ;
#39504=DIRECTION('center_axis',(0.0914824783325258,0.92000541566125,-0.381078720623586)) ;
#39505=DIRECTION('ref_axis',(0.995806686138499,-0.0845187893148279,0.0350088288095559)) ;
#39506=DIRECTION('',(-0.0914824783325258,-0.92000541566125,0.381078720623586)) ;
#39507=DIRECTION('center_axis',(-0.0989489060816219,-0.703636665469234,
0.70363666546918)) ;
#39508=DIRECTION('ref_axis',(4.33621020017968E-14,-0.707106781186523,-0.707106781186572)) ;
#39509=DIRECTION('center_axis',(-0.0989489060816219,-0.703636665469234,
0.70363666546918)) ;
#39510=DIRECTION('ref_axis',(4.33621020017968E-14,-0.707106781186523,-0.707106781186572)) ;
#39511=DIRECTION('center_axis',(0.0914824783325313,0.381078720623583,-0.920005415661251)) ;
#39512=DIRECTION('ref_axis',(0.995806686138498,-0.0350088288095578,0.084518789314833)) ;
#39513=DIRECTION('',(-0.0914824783325313,-0.381078720623583,0.920005415661251)) ;
#39514=DIRECTION('center_axis',(-0.0989489060816132,-2.16674034761705E-15,
0.995092515289534)) ;
#39515=DIRECTION('ref_axis',(4.78474679960641E-15,-1.,-1.6933726801959E-15)) ;
#39516=DIRECTION('center_axis',(-0.0989489060816132,-2.16674034761705E-15,
0.995092515289534)) ;
#39517=DIRECTION('ref_axis',(4.78474679960641E-15,-1.,-1.6933726801959E-15)) ;
#39518=DIRECTION('center_axis',(0.0914824783325254,-0.381078720623587,-0.92000541566125)) ;
#39519=DIRECTION('ref_axis',(0.995806686138499,0.0350088288095558,0.0845187893148275)) ;
#39520=DIRECTION('',(-0.0914824783325254,0.381078720623587,0.92000541566125)) ;
#39521=DIRECTION('center_axis',(-0.0989489060815864,0.703636665469225,0.703636665469195)) ;
#39522=DIRECTION('ref_axis',(-4.72700907286251E-14,-0.707106781186536,0.707106781186559)) ;
#39523=DIRECTION('center_axis',(-0.0989489060815864,0.703636665469225,0.703636665469195)) ;
#39524=DIRECTION('ref_axis',(-4.72700907286251E-14,-0.707106781186536,0.707106781186559)) ;
#39525=DIRECTION('center_axis',(0.0914824783325237,-0.920005415661249,-0.381078720623589)) ;
#39526=DIRECTION('ref_axis',(0.995806686138499,0.0845187893148259,0.0350088288095553)) ;
#39527=DIRECTION('',(-0.0914824783325237,0.920005415661249,0.381078720623589)) ;
#39528=DIRECTION('center_axis',(-0.0989489060816074,0.995092515289535,-1.78746959168219E-14)) ;
#39529=DIRECTION('ref_axis',(7.99239828537599E-15,1.86738777329889E-14,
1.)) ;
#39530=DIRECTION('center_axis',(-0.0989489060816074,0.995092515289535,-1.78746959168219E-14)) ;
#39531=DIRECTION('ref_axis',(7.99239828537599E-15,1.86738777329889E-14,
1.)) ;
#39532=DIRECTION('center_axis',(0.0914824783325308,-0.920005415661242,0.381078720623606)) ;
#39533=DIRECTION('ref_axis',(0.995806686138498,0.0845187893148318,-0.0350088288095597)) ;
#39534=DIRECTION('',(-0.0914824783325308,0.920005415661241,-0.381078720623606)) ;
#39535=DIRECTION('center_axis',(-0.0989489060815945,0.703636665469208,-0.70363666546921)) ;
#39536=DIRECTION('ref_axis',(-3.81282839941823E-14,0.707106781186546,0.707106781186549)) ;
#39537=DIRECTION('center_axis',(-0.0989489060815945,0.703636665469208,-0.70363666546921)) ;
#39538=DIRECTION('ref_axis',(-3.81282839941823E-14,0.707106781186546,0.707106781186549)) ;
#39539=DIRECTION('center_axis',(0.0914824783325257,-0.381078720623581,0.920005415661252)) ;
#39540=DIRECTION('ref_axis',(0.995806686138499,0.0350088288095554,-0.0845187893148279)) ;
#39541=DIRECTION('',(-0.0914824783325257,0.381078720623581,-0.920005415661252)) ;
#39542=DIRECTION('center_axis',(-0.0989489060816132,-4.35802109972037E-14,
-0.995092515289534)) ;
#39543=DIRECTION('ref_axis',(1.53539584452172E-14,1.,-4.53187694081149E-14)) ;
#39544=DIRECTION('center_axis',(-0.0989489060816132,-4.35802109972037E-14,
-0.995092515289534)) ;
#39545=DIRECTION('ref_axis',(1.53539584452172E-14,1.,-4.53187694081149E-14)) ;
#39546=DIRECTION('center_axis',(0.091482478332532,0.381078720623593,0.920005415661247)) ;
#39547=DIRECTION('ref_axis',(0.995806686138498,-0.0350088288095589,-0.0845187893148333)) ;
#39548=DIRECTION('',(-0.091482478332532,-0.381078720623593,-0.920005415661247)) ;
#39549=DIRECTION('center_axis',(-0.0989489060816209,-0.703636665469204,
-0.703636665469211)) ;
#39550=DIRECTION('ref_axis',(2.21060648227627E-14,0.707106781186549,-0.707106781186546)) ;
#39551=DIRECTION('center_axis',(-0.0989489060816209,-0.703636665469204,
-0.703636665469211)) ;
#39552=DIRECTION('ref_axis',(2.21060648227627E-14,0.707106781186549,-0.707106781186546)) ;
#39553=DIRECTION('center_axis',(0.0914824783325256,0.920005415661251,0.381078720623585)) ;
#39554=DIRECTION('ref_axis',(0.995806686138499,-0.0845187893148277,-0.0350088288095557)) ;
#39555=DIRECTION('',(-0.0914824783325256,-0.920005415661251,-0.381078720623585)) ;
#39556=DIRECTION('center_axis',(-0.098948906081604,-0.995092515289535,5.2432441356011E-14)) ;
#39557=DIRECTION('ref_axis',(-8.39870080690671E-15,-5.18744071321563E-14,
-1.)) ;
#39558=DIRECTION('center_axis',(-0.098948906081604,-0.995092515289535,5.2432441356011E-14)) ;
#39559=DIRECTION('ref_axis',(-8.39870080690671E-15,-5.18744071321563E-14,
-1.)) ;
#39560=DIRECTION('center_axis',(0.0914824783325256,0.920005415661251,-0.381078720623585)) ;
#39561=DIRECTION('ref_axis',(0.995806686138499,-0.0845187893148277,0.0350088288095557)) ;
#39562=DIRECTION('',(-0.0914824783325256,-0.920005415661251,0.381078720623585)) ;
#39563=DIRECTION('center_axis',(-0.0989489060816204,-0.703636665469235,
0.70363666546918)) ;
#39564=DIRECTION('ref_axis',(4.02934487470771E-14,-0.707106781186523,-0.707106781186572)) ;
#39565=DIRECTION('center_axis',(-0.0989489060816204,-0.703636665469235,
0.70363666546918)) ;
#39566=DIRECTION('ref_axis',(4.02934487470771E-14,-0.707106781186523,-0.707106781186572)) ;
#39567=DIRECTION('center_axis',(0.0914824783325301,0.381078720623585,-0.92000541566125)) ;
#39568=DIRECTION('ref_axis',(0.995806686138499,-0.0350088288095575,0.0845187893148319)) ;
#39569=DIRECTION('',(-0.0914824783325301,-0.381078720623585,0.92000541566125)) ;
#39570=DIRECTION('center_axis',(-0.0989489060816109,0.,0.995092515289535)) ;
#39571=DIRECTION('ref_axis',(1.78024657460216E-15,-1.,1.88449524788967E-16)) ;
#39572=DIRECTION('center_axis',(-0.0989489060816109,0.,0.995092515289535)) ;
#39573=DIRECTION('ref_axis',(1.78024657460216E-15,-1.,1.88449524788967E-16)) ;
#39574=DIRECTION('center_axis',(0.0914824783325252,-0.381078720623592,-0.920005415661248)) ;
#39575=DIRECTION('ref_axis',(0.995806686138499,0.0350088288095562,0.0845187893148271)) ;
#39576=DIRECTION('',(-0.0914824783325252,0.381078720623592,0.920005415661248)) ;
#39577=DIRECTION('center_axis',(-0.098948906081596,0.703636665469203,0.703636665469215)) ;
#39578=DIRECTION('ref_axis',(-2.01600895880624E-14,-0.707106781186555,0.70710678118654)) ;
#39579=DIRECTION('center_axis',(-0.098948906081596,0.703636665469203,0.703636665469215)) ;
#39580=DIRECTION('ref_axis',(-2.01600895880624E-14,-0.707106781186555,0.70710678118654)) ;
#39581=DIRECTION('center_axis',(0.0914824783325312,-0.920005415661251,-0.381078720623584)) ;
#39582=DIRECTION('ref_axis',(0.995806686138498,0.0845187893148329,0.0350088288095578)) ;
#39583=DIRECTION('',(-0.0914824783325312,0.92000541566125,0.381078720623584)) ;
#39584=DIRECTION('center_axis',(-0.0989489060816085,0.995092515289535,-6.26465533084806E-14)) ;
#39585=DIRECTION('ref_axis',(-1.31353328342264E-14,6.16290089525266E-14,
1.)) ;
#39586=DIRECTION('center_axis',(-0.0989489060816085,0.995092515289535,-6.26465533084806E-14)) ;
#39587=DIRECTION('ref_axis',(-1.31353328342264E-14,6.16290089525266E-14,
1.)) ;
#39588=DIRECTION('center_axis',(0.0914824783325253,-0.920005415661246,0.381078720623595)) ;
#39589=DIRECTION('ref_axis',(0.995806686138499,0.0845187893148271,-0.0350088288095565)) ;
#39590=DIRECTION('',(-0.0914824783325253,0.920005415661246,-0.381078720623595)) ;
#39591=DIRECTION('center_axis',(-0.098948906081588,0.703636665469237,-0.703636665469183)) ;
#39592=DIRECTION('ref_axis',(-3.65458425945363E-14,0.707106781186518,0.707106781186577)) ;
#39593=DIRECTION('center_axis',(-0.098948906081588,0.703636665469237,-0.703636665469183)) ;
#39594=DIRECTION('ref_axis',(-3.65458425945363E-14,0.707106781186518,0.707106781186577)) ;
#39595=DIRECTION('center_axis',(0.0914824783325254,-0.381078720623587,0.92000541566125)) ;
#39596=DIRECTION('ref_axis',(0.995806686138499,0.0350088288095558,-0.0845187893148275)) ;
#39597=DIRECTION('',(-0.0914824783325254,0.381078720623587,-0.92000541566125)) ;
#39598=DIRECTION('center_axis',(-0.0989489060816109,0.,-0.995092515289535)) ;
#39599=DIRECTION('ref_axis',(1.4022783078623E-14,1.,-1.41604447882206E-15)) ;
#39600=DIRECTION('center_axis',(-0.0989489060816109,0.,-0.995092515289535)) ;
#39601=DIRECTION('ref_axis',(1.4022783078623E-14,1.,-1.41604447882206E-15)) ;
#39602=DIRECTION('center_axis',(0.0914824783325299,0.38107872062359,0.920005415661248)) ;
#39603=DIRECTION('ref_axis',(0.995806686138498,-0.0350088288095579,-0.0845187893148314)) ;
#39604=DIRECTION('',(-0.0914824783325299,-0.38107872062359,-0.920005415661248)) ;
#39605=DIRECTION('center_axis',(-0.0989489060816232,-0.703636665469224,
-0.703636665469191)) ;
#39606=DIRECTION('ref_axis',(3.05314960587173E-14,0.707106781186529,-0.707106781186566)) ;
#39607=DIRECTION('center_axis',(-0.0989489060816232,-0.703636665469224,
-0.703636665469191)) ;
#39608=DIRECTION('ref_axis',(3.05314960587173E-14,0.707106781186529,-0.707106781186566)) ;
#39609=DIRECTION('center_axis',(0.0914824783325257,0.920005415661255,0.381078720623574)) ;
#39610=DIRECTION('ref_axis',(0.995806686138499,-0.0845187893148283,-0.0350088288095548)) ;
#39611=DIRECTION('',(-0.0914824783325257,-0.920005415661255,-0.381078720623574)) ;
#39612=DIRECTION('center_axis',(-0.0989489060816096,-0.995092515289535,
6.65156456481759E-14)) ;
#39613=DIRECTION('ref_axis',(4.57624945303127E-15,-6.72584373100524E-14,
-1.)) ;
#39614=DIRECTION('center_axis',(-0.0989489060816096,-0.995092515289535,
6.65156456481759E-14)) ;
#39615=DIRECTION('ref_axis',(4.57624945303127E-15,-6.72584373100524E-14,
-1.)) ;
#39616=DIRECTION('center_axis',(0.0914824783325315,0.92000541566125,-0.381078720623586)) ;
#39617=DIRECTION('ref_axis',(0.995806686138498,-0.0845187893148332,0.0350088288095581)) ;
#39618=DIRECTION('',(-0.0914824783325315,-0.92000541566125,0.381078720623586)) ;
#39619=DIRECTION('center_axis',(-0.098948906081596,-0.703636665469235,0.703636665469184)) ;
#39620=DIRECTION('ref_axis',(-3.45945212740262E-14,-0.707106781186519,-0.707106781186576)) ;
#39621=DIRECTION('center_axis',(-0.098948906081596,-0.703636665469235,0.703636665469184)) ;
#39622=DIRECTION('ref_axis',(-3.45945212740262E-14,-0.707106781186519,-0.707106781186576)) ;
#39623=DIRECTION('center_axis',(0.0914824783325256,0.381078720623584,-0.920005415661251)) ;
#39624=DIRECTION('ref_axis',(0.995806686138499,-0.0350088288095556,0.0845187893148277)) ;
#39625=DIRECTION('',(-0.0914824783325255,-0.381078720623584,0.920005415661251)) ;
#39626=DIRECTION('center_axis',(-0.0989489060816109,0.,0.995092515289535)) ;
#39627=DIRECTION('ref_axis',(1.40655517651E-14,-1.,1.3953283963098E-15)) ;
#39628=DIRECTION('center_axis',(-0.0989489060816109,0.,0.995092515289535)) ;
#39629=DIRECTION('ref_axis',(1.40655517651E-14,-1.,1.3953283963098E-15)) ;
#39630=DIRECTION('center_axis',(0.0914824783325255,-0.381078720623586,-0.92000541566125)) ;
#39631=DIRECTION('ref_axis',(0.995806686138499,0.0350088288095558,0.0845187893148275)) ;
#39632=DIRECTION('',(-0.0914824783325255,0.381078720623586,0.92000541566125)) ;
#39633=DIRECTION('center_axis',(-0.0989489060815955,0.70363666546922,0.703636665469198)) ;
#39634=DIRECTION('ref_axis',(-2.49234520444301E-14,-0.707106781186538,0.707106781186557)) ;
#39635=DIRECTION('center_axis',(-0.0989489060815955,0.70363666546922,0.703636665469198)) ;
#39636=DIRECTION('ref_axis',(-2.49234520444301E-14,-0.707106781186538,0.707106781186557)) ;
#39637=DIRECTION('center_axis',(0.091482478332531,-0.920005415661246,-0.381078720623595)) ;
#39638=DIRECTION('ref_axis',(0.995806686138498,0.0845187893148324,0.0350088288095587)) ;
#39639=DIRECTION('',(-0.091482478332531,0.920005415661246,0.381078720623595)) ;
#39640=DIRECTION('center_axis',(-0.0989489060816065,0.995092515289535,-5.10705597623483E-15)) ;
#39641=DIRECTION('ref_axis',(-1.26381468539324E-14,3.88860916576948E-15,
1.)) ;
#39642=DIRECTION('center_axis',(-0.0989489060816065,0.995092515289535,-5.10705597623483E-15)) ;
#39643=DIRECTION('ref_axis',(-1.26381468539324E-14,3.88860916576948E-15,
1.)) ;
#39644=DIRECTION('center_axis',(0.0914824783325236,-0.920005415661245,0.3810787206236)) ;
#39645=DIRECTION('ref_axis',(0.995806686138499,0.0845187893148253,-0.0350088288095563)) ;
#39646=DIRECTION('',(-0.0914824783325235,0.920005415661245,-0.3810787206236)) ;
#39647=DIRECTION('center_axis',(-0.0989489060816173,0.703636665469211,-0.703636665469204)) ;
#39648=DIRECTION('ref_axis',(3.62090391885301E-14,0.707106781186547,0.707106781186548)) ;
#39649=DIRECTION('center_axis',(-0.0989489060816173,0.703636665469211,-0.703636665469204)) ;
#39650=DIRECTION('ref_axis',(3.62090391885301E-14,0.707106781186547,0.707106781186548)) ;
#39651=DIRECTION('center_axis',(0.0914824783325314,-0.381078720623581,0.920005415661252)) ;
#39652=DIRECTION('ref_axis',(0.995806686138498,0.0350088288095576,-0.0845187893148332)) ;
#39653=DIRECTION('',(-0.0914824783325314,0.381078720623581,-0.920005415661252)) ;
#39654=DIRECTION('center_axis',(-0.0989489060816132,-4.14134706495866E-14,
-0.995092515289534)) ;
#39655=DIRECTION('ref_axis',(4.70455551246209E-16,1.,-4.16426671532777E-14)) ;
#39656=DIRECTION('center_axis',(-0.0989489060816132,-4.14134706495866E-14,
-0.995092515289534)) ;
#39657=DIRECTION('ref_axis',(4.70455551246209E-16,1.,-4.16426671532777E-14)) ;
#39658=DIRECTION('center_axis',(0.0914824783325263,0.381078720623593,0.920005415661247)) ;
#39659=DIRECTION('ref_axis',(0.995806686138499,-0.0350088288095567,-0.0845187893148281)) ;
#39660=DIRECTION('',(-0.0914824783325263,-0.381078720623593,-0.920005415661247)) ;
#39661=DIRECTION('center_axis',(-0.098948906081588,-0.703636665469206,-0.703636665469214)) ;
#39662=DIRECTION('ref_axis',(-4.28809542789309E-14,0.707106781186554,-0.707106781186541)) ;
#39663=DIRECTION('center_axis',(-0.098948906081588,-0.703636665469206,-0.703636665469214)) ;
#39664=DIRECTION('ref_axis',(-4.28809542789309E-14,0.707106781186554,-0.707106781186541)) ;
#39665=DIRECTION('center_axis',(0.0914824783325256,0.920005415661251,0.381078720623585)) ;
#39666=DIRECTION('ref_axis',(0.995806686138499,-0.0845187893148277,-0.0350088288095557)) ;
#39667=DIRECTION('',(-0.0914824783325256,-0.920005415661251,-0.381078720623585)) ;
#39668=DIRECTION('center_axis',(-0.0989489060816085,-0.995092515289535,
4.61337389853213E-14)) ;
#39669=DIRECTION('ref_axis',(3.44822534720232E-15,-4.66893721575551E-14,
-1.)) ;
#39670=DIRECTION('center_axis',(-0.0989489060816085,-0.995092515289535,
4.61337389853213E-14)) ;
#39671=DIRECTION('ref_axis',(3.44822534720232E-15,-4.66893721575551E-14,
-1.)) ;
#39672=DIRECTION('center_axis',(0.0914824783325317,0.920005415661254,-0.381078720623575)) ;
#39673=DIRECTION('ref_axis',(0.995806686138498,-0.0845187893148337,0.0350088288095571)) ;
#39674=DIRECTION('',(-0.0914824783325317,-0.920005415661254,0.381078720623575)) ;
#39675=DIRECTION('center_axis',(-0.0989489060815971,-0.703636665469235,
0.703636665469183)) ;
#39676=DIRECTION('ref_axis',(-3.36749945147721E-14,-0.707106781186519,-0.707106781186576)) ;
#39677=DIRECTION('center_axis',(-0.0989489060815971,-0.703636665469235,
0.703636665469183)) ;
#39678=DIRECTION('ref_axis',(-3.36749945147721E-14,-0.707106781186519,-0.707106781186576)) ;
#39679=DIRECTION('center_axis',(0.0914824783325234,0.381078720623582,-0.920005415661252)) ;
#39680=DIRECTION('ref_axis',(0.995806686138499,-0.0350088288095545,0.0845187893148258)) ;
#39681=DIRECTION('',(-0.0914824783325234,-0.381078720623582,0.920005415661252)) ;
#39682=DIRECTION('center_axis',(-0.0989489060816109,4.14134706495867E-14,
0.995092515289535)) ;
#39683=DIRECTION('ref_axis',(1.57549148809384E-14,-1.,4.31629603053873E-14)) ;
#39684=DIRECTION('center_axis',(-0.0989489060816109,4.14134706495867E-14,
0.995092515289535)) ;
#39685=DIRECTION('ref_axis',(1.57549148809384E-14,-1.,4.31629603053873E-14)) ;
#39686=DIRECTION('center_axis',(0.091482478332531,-0.381078720623592,-0.920005415661248)) ;
#39687=DIRECTION('ref_axis',(0.995806686138498,0.0350088288095584,0.0845187893148324)) ;
#39688=DIRECTION('',(-0.091482478332531,0.381078720623591,0.920005415661247)) ;
#39689=DIRECTION('center_axis',(-0.0989489060816217,0.703636665469202,0.703636665469212)) ;
#39690=DIRECTION('ref_axis',(2.68961577081787E-14,-0.707106781186551,0.707106781186544)) ;
#39691=DIRECTION('center_axis',(-0.0989489060816217,0.703636665469202,0.703636665469212)) ;
#39692=DIRECTION('ref_axis',(2.68961577081787E-14,-0.707106781186551,0.707106781186544)) ;
#39693=DIRECTION('center_axis',(0.0914824783325255,-0.920005415661251,-0.381078720623585)) ;
#39694=DIRECTION('ref_axis',(0.995806686138499,0.0845187893148276,0.0350088288095556)) ;
#39695=DIRECTION('',(-0.0914824783325255,0.920005415661251,0.381078720623585)) ;
#39696=DIRECTION('center_axis',(-0.098948906081604,0.995092515289535,-6.50298460973902E-14)) ;
#39697=DIRECTION('ref_axis',(-9.37703451006639E-15,6.44357040025749E-14,
1.)) ;
#39698=DIRECTION('center_axis',(-0.098948906081604,0.995092515289535,-6.50298460973902E-14)) ;
#39699=DIRECTION('ref_axis',(-9.37703451006639E-15,6.44357040025749E-14,
1.)) ;
#39700=DIRECTION('center_axis',(0.0914824783325253,-0.920005415661247,0.381078720623595)) ;
#39701=DIRECTION('ref_axis',(0.995806686138499,0.084518789314827,-0.0350088288095565)) ;
#39702=DIRECTION('',(-0.0914824783325253,0.920005415661246,-0.381078720623595)) ;
#39703=DIRECTION('center_axis',(-0.0989489060816193,0.703636665469236,-0.703636665469179)) ;
#39704=DIRECTION('ref_axis',(3.96946871364003E-14,0.707106781186521,0.707106781186574)) ;
#39705=DIRECTION('center_axis',(-0.0989489060816193,0.703636665469236,-0.703636665469179)) ;
#39706=DIRECTION('ref_axis',(3.96946871364003E-14,0.707106781186521,0.707106781186574)) ;
#39707=DIRECTION('center_axis',(0.0914824783325311,-0.381078720623587,0.920005415661249)) ;
#39708=DIRECTION('ref_axis',(0.995806686138498,0.035008828809558,-0.0845187893148328)) ;
#39709=DIRECTION('',(-0.0914824783325311,0.381078720623587,-0.920005415661249)) ;
#39710=DIRECTION('center_axis',(-0.0989489060816109,2.16674034761701E-15,
-0.995092515289535)) ;
#39711=DIRECTION('ref_axis',(-8.55373729538575E-16,1.,2.21795735026448E-15)) ;
#39712=DIRECTION('center_axis',(-0.0989489060816109,2.16674034761701E-15,
-0.995092515289535)) ;
#39713=DIRECTION('ref_axis',(-8.55373729538575E-16,1.,2.21795735026448E-15)) ;
#39714=DIRECTION('center_axis',(0.0914824783325242,0.38107872062359,0.920005415661249)) ;
#39715=DIRECTION('ref_axis',(0.995806686138499,-0.0350088288095556,-0.0845187893148262)) ;
#39716=DIRECTION('',(-0.0914824783325242,-0.38107872062359,-0.920005415661249)) ;
#39717=DIRECTION('center_axis',(-0.098948906081595,-0.703636665469224,-0.703636665469195)) ;
#39718=DIRECTION('ref_axis',(-2.30683602684933E-14,0.707106781186534,-0.70710678118656)) ;
#39719=DIRECTION('center_axis',(-0.098948906081595,-0.703636665469224,-0.703636665469195)) ;
#39720=DIRECTION('ref_axis',(-2.30683602684933E-14,0.707106781186534,-0.70710678118656)) ;
#39721=DIRECTION('center_axis',(0.0914824783325315,0.920005415661255,0.381078720623574)) ;
#39722=DIRECTION('ref_axis',(0.995806686138498,-0.0845187893148336,-0.035008828809557)) ;
#39723=DIRECTION('',(-0.0914824783325315,-0.920005415661255,-0.381078720623574)) ;
#39724=DIRECTION('center_axis',(-0.0989489060816085,-0.995092515289535,
6.21821649529419E-14)) ;
#39725=DIRECTION('ref_axis',(-1.25098407945014E-14,-6.12460955564131E-14,
-1.)) ;
#39726=DIRECTION('center_axis',(-0.0989489060816085,-0.995092515289535,
6.21821649529419E-14)) ;
#39727=DIRECTION('ref_axis',(-1.25098407945014E-14,-6.12460955564131E-14,
-1.)) ;
#39728=DIRECTION('center_axis',(0.0914824783325258,0.92000541566125,-0.381078720623586)) ;
#39729=DIRECTION('ref_axis',(0.995806686138499,-0.0845187893148279,0.0350088288095559)) ;
#39730=DIRECTION('',(-0.0914824783325258,-0.92000541566125,0.381078720623586)) ;
#39731=DIRECTION('center_axis',(-0.0989489060815885,-0.703636665469235,
0.703636665469185)) ;
#39732=DIRECTION('ref_axis',(-3.78182110172248E-14,-0.70710678118652,-0.707106781186575)) ;
#39733=DIRECTION('center_axis',(-0.0989489060815885,-0.703636665469235,
0.703636665469185)) ;
#39734=DIRECTION('ref_axis',(-3.78182110172248E-14,-0.70710678118652,-0.707106781186575)) ;
#39735=DIRECTION('center_axis',(0.0914824783325255,0.381078720623584,-0.920005415661251)) ;
#39736=DIRECTION('ref_axis',(0.995806686138499,-0.0350088288095556,0.0845187893148277)) ;
#39737=DIRECTION('',(-0.0914824783325255,-0.381078720623584,0.920005415661251)) ;
#39738=DIRECTION('center_axis',(-0.0989489060816109,0.,0.995092515289535)) ;
#39739=DIRECTION('ref_axis',(1.40334752502423E-14,-1.,1.3953283963098E-15)) ;
#39740=DIRECTION('center_axis',(-0.0989489060816109,0.,0.995092515289535)) ;
#39741=DIRECTION('ref_axis',(1.40334752502423E-14,-1.,1.3953283963098E-15)) ;
#39742=DIRECTION('center_axis',(0.0914824783325312,-0.381078720623586,-0.92000541566125)) ;
#39743=DIRECTION('ref_axis',(0.995806686138498,0.0350088288095579,0.0845187893148329)) ;
#39744=DIRECTION('',(-0.0914824783325312,0.381078720623586,0.92000541566125)) ;
#39745=DIRECTION('center_axis',(-0.0989489060816175,0.703636665469224,0.703636665469192)) ;
#39746=DIRECTION('ref_axis',(1.2600724253265E-14,-0.707106781186531,0.707106781186564)) ;
#39747=DIRECTION('center_axis',(-0.0989489060816175,0.703636665469224,0.703636665469192)) ;
#39748=DIRECTION('ref_axis',(1.2600724253265E-14,-0.707106781186531,0.707106781186564)) ;
#39749=DIRECTION('center_axis',(0.0914824783325238,-0.920005415661249,-0.381078720623589)) ;
#39750=DIRECTION('ref_axis',(0.995806686138499,0.0845187893148259,0.0350088288095554)) ;
#39751=DIRECTION('',(-0.0914824783325237,0.920005415661249,0.381078720623589)) ;
#39752=DIRECTION('center_axis',(-0.0989489060816076,0.995092515289535,-1.53211679287045E-14)) ;
#39753=DIRECTION('ref_axis',(8.62858249672031E-15,1.6239403907435E-14,1.)) ;
#39754=DIRECTION('center_axis',(-0.0989489060816076,0.995092515289535,-1.53211679287045E-14)) ;
#39755=DIRECTION('ref_axis',(8.62858249672031E-15,1.6239403907435E-14,1.)) ;
#39756=DIRECTION('center_axis',(0.0914824783325308,-0.920005415661242,0.381078720623606)) ;
#39757=DIRECTION('ref_axis',(0.995806686138498,0.0845187893148317,-0.0350088288095596)) ;
#39758=DIRECTION('',(-0.0914824783325308,0.920005415661242,-0.381078720623606)) ;
#39759=DIRECTION('center_axis',(-0.0989489060815925,0.703636665469211,-0.703636665469208)) ;
#39760=DIRECTION('ref_axis',(-4.25013821864484E-14,0.707106781186543,0.707106781186552)) ;
#39761=DIRECTION('center_axis',(-0.0989489060815925,0.703636665469211,-0.703636665469208)) ;
#39762=DIRECTION('ref_axis',(-4.25013821864484E-14,0.707106781186543,0.707106781186552)) ;
#39763=DIRECTION('center_axis',(0.0914824783325257,-0.381078720623582,0.920005415661252)) ;
#39764=DIRECTION('ref_axis',(0.995806686138499,0.0350088288095554,-0.0845187893148279)) ;
#39765=DIRECTION('',(-0.0914824783325257,0.381078720623582,-0.920005415661252)) ;
#39766=DIRECTION('center_axis',(-0.0989489060816109,-4.35802109972037E-14,
-0.995092515289535)) ;
#39767=DIRECTION('ref_axis',(9.55880142759342E-15,1.,-4.4753420833748E-14)) ;
#39768=DIRECTION('center_axis',(-0.0989489060816109,-4.35802109972037E-14,
-0.995092515289535)) ;
#39769=DIRECTION('ref_axis',(9.55880142759342E-15,1.,-4.4753420833748E-14)) ;
#39770=DIRECTION('center_axis',(0.0914824783325263,0.381078720623592,0.920005415661247)) ;
#39771=DIRECTION('ref_axis',(0.995806686138499,-0.0350088288095567,-0.0845187893148281)) ;
#39772=DIRECTION('',(-0.0914824783325263,-0.381078720623592,-0.920005415661247)) ;
#39773=DIRECTION('center_axis',(-0.0989489060815955,-0.703636665469203,
-0.703636665469215)) ;
#39774=DIRECTION('ref_axis',(-2.4260537404038E-14,0.707106781186555,-0.70710678118654)) ;
#39775=DIRECTION('center_axis',(-0.0989489060815955,-0.703636665469203,
-0.703636665469215)) ;
#39776=DIRECTION('ref_axis',(-2.4260537404038E-14,0.707106781186555,-0.70710678118654)) ;
#39777=DIRECTION('center_axis',(0.0914824783325313,0.92000541566125,0.381078720623585)) ;
#39778=DIRECTION('ref_axis',(0.995806686138498,-0.084518789314833,-0.0350088288095579)) ;
#39779=DIRECTION('',(-0.0914824783325313,-0.92000541566125,-0.381078720623585)) ;
#39780=DIRECTION('center_axis',(-0.0989489060816096,-0.995092515289535,
4.42611517940352E-14)) ;
#39781=DIRECTION('ref_axis',(-8.98142416015488E-15,-4.35926519523351E-14,
-1.)) ;
#39782=DIRECTION('center_axis',(-0.0989489060816096,-0.995092515289535,
4.42611517940352E-14)) ;
#39783=DIRECTION('ref_axis',(-8.98142416015488E-15,-4.35926519523351E-14,
-1.)) ;
#39784=DIRECTION('center_axis',(0.091482478332526,0.920005415661255,-0.381078720623575)) ;
#39785=DIRECTION('ref_axis',(0.995806686138499,-0.0845187893148284,0.0350088288095549)) ;
#39786=DIRECTION('',(-0.0914824783325259,-0.920005415661255,0.381078720623575)) ;
#39787=DIRECTION('center_axis',(-0.0989489060816214,-0.703636665469236,
0.703636665469179)) ;
#39788=DIRECTION('ref_axis',(4.08868642719443E-14,-0.707106781186522,-0.707106781186573)) ;
#39789=DIRECTION('center_axis',(-0.0989489060816214,-0.703636665469236,
0.703636665469179)) ;
#39790=DIRECTION('ref_axis',(4.08868642719443E-14,-0.707106781186522,-0.707106781186573)) ;
#39791=DIRECTION('center_axis',(0.0914824783325291,0.381078720623582,-0.920005415661252)) ;
#39792=DIRECTION('ref_axis',(0.995806686138499,-0.0350088288095568,0.0845187893148311)) ;
#39793=DIRECTION('',(-0.0914824783325291,-0.381078720623582,0.920005415661252)) ;
#39794=DIRECTION('center_axis',(-0.0989489060816133,4.14134706495866E-14,
0.995092515289534)) ;
#39795=DIRECTION('ref_axis',(6.59172380325654E-15,-1.,4.22561304999312E-14)) ;
#39796=DIRECTION('center_axis',(-0.0989489060816133,4.14134706495866E-14,
0.995092515289534)) ;
#39797=DIRECTION('ref_axis',(6.59172380325654E-15,-1.,4.22561304999312E-14)) ;
#39798=DIRECTION('center_axis',(0.0914824783325252,-0.381078720623591,-0.920005415661248)) ;
#39799=DIRECTION('ref_axis',(0.995806686138499,0.0350088288095562,0.0845187893148272)) ;
#39800=DIRECTION('',(-0.0914824783325252,0.381078720623591,0.920005415661248)) ;
#39801=DIRECTION('center_axis',(-0.0989489060815885,0.703636665469205,0.703636665469215)) ;
#39802=DIRECTION('ref_axis',(-3.85987395454284E-14,-0.707106781186555,0.70710678118654)) ;
#39803=DIRECTION('center_axis',(-0.0989489060815885,0.703636665469205,0.703636665469215)) ;
#39804=DIRECTION('ref_axis',(-3.85987395454284E-14,-0.707106781186555,0.70710678118654)) ;
#39805=DIRECTION('center_axis',(0.0914824783325255,-0.920005415661251,-0.381078720623585)) ;
#39806=DIRECTION('ref_axis',(0.995806686138499,0.0845187893148276,0.0350088288095556)) ;
#39807=DIRECTION('',(-0.0914824783325255,0.920005415661251,0.381078720623585)) ;
#39808=DIRECTION('center_axis',(-0.0989489060816085,0.995092515289535,-6.11144365156102E-14)) ;
#39809=DIRECTION('ref_axis',(2.2453560400387E-15,6.1689820678611E-14,1.)) ;
#39810=DIRECTION('center_axis',(-0.0989489060816085,0.995092515289535,-6.11144365156102E-14)) ;
#39811=DIRECTION('ref_axis',(2.2453560400387E-15,6.1689820678611E-14,1.)) ;
#39812=DIRECTION('center_axis',(0.091482478332531,-0.920005415661246,0.381078720623595)) ;
#39813=DIRECTION('ref_axis',(0.995806686138498,0.0845187893148323,-0.0350088288095587)) ;
#39814=DIRECTION('',(-0.091482478332531,0.920005415661246,-0.381078720623595)) ;
#39815=DIRECTION('center_axis',(-0.0989489060815932,0.70363666546921,-0.703636665469208)) ;
#39816=DIRECTION('ref_axis',(-4.25548430445443E-14,0.707106781186543,0.707106781186552)) ;
#39817=DIRECTION('center_axis',(-0.0989489060815932,0.70363666546921,-0.703636665469208)) ;
#39818=DIRECTION('ref_axis',(-4.25548430445443E-14,0.707106781186543,0.707106781186552)) ;
#39819=DIRECTION('center_axis',(0.0914824783325244,-0.381078720623583,0.920005415661252)) ;
#39820=DIRECTION('ref_axis',(0.995806686138499,0.0350088288095551,-0.0845187893148267)) ;
#39821=DIRECTION('',(-0.0914824783325244,0.381078720623583,-0.920005415661251)) ;
#39822=DIRECTION('center_axis',(-0.0989489060815898,-4.35802109972035E-14,
-0.995092515289537)) ;
#39823=DIRECTION('ref_axis',(-3.85720091163795E-14,1.,-3.99259053476647E-14)) ;
#39824=DIRECTION('center_axis',(-0.0989489060815898,-4.35802109972035E-14,
-0.995092515289537)) ;
#39825=DIRECTION('ref_axis',(-3.85720091163795E-14,1.,-3.99259053476647E-14)) ;
#39826=DIRECTION('center_axis',(0.0914824783325321,0.381078720623592,0.920005415661247)) ;
#39827=DIRECTION('ref_axis',(0.995806686138498,-0.0350088288095589,-0.0845187893148334)) ;
#39828=DIRECTION('',(-0.091482478332532,-0.381078720623592,-0.920005415661247)) ;
#39829=DIRECTION('center_axis',(-0.0989489060816185,-0.703636665469205,
-0.70363666546921)) ;
#39830=DIRECTION('ref_axis',(1.60115269998003E-14,0.707106781186549,-0.707106781186546)) ;
#39831=DIRECTION('center_axis',(-0.0989489060816185,-0.703636665469205,
-0.70363666546921)) ;
#39832=DIRECTION('ref_axis',(1.60115269998003E-14,0.707106781186549,-0.707106781186546)) ;
#39833=DIRECTION('center_axis',(0.0914824783325248,0.920005415661252,0.381078720623582)) ;
#39834=DIRECTION('ref_axis',(0.995806686138499,-0.0845187893148271,-0.0350088288095551)) ;
#39835=DIRECTION('',(-0.0914824783325248,-0.920005415661252,-0.381078720623582)) ;
#39836=DIRECTION('center_axis',(-0.0989489060816036,-0.995092515289535,
5.58371453401675E-14)) ;
#39837=DIRECTION('ref_axis',(-7.30809930174505E-15,-5.5452943320968E-14,
-1.)) ;
#39838=DIRECTION('center_axis',(-0.0989489060816036,-0.995092515289535,
5.58371453401675E-14)) ;
#39839=DIRECTION('ref_axis',(-7.30809930174505E-15,-5.5452943320968E-14,
-1.)) ;
#39840=DIRECTION('center_axis',(0.0914824783325258,0.92000541566125,-0.381078720623586)) ;
#39841=DIRECTION('ref_axis',(0.995806686138499,-0.0845187893148278,0.0350088288095558)) ;
#39842=DIRECTION('',(-0.0914824783325258,-0.92000541566125,0.381078720623586)) ;
#39843=DIRECTION('center_axis',(-0.0989489060816206,-0.703636665469235,
0.70363666546918)) ;
#39844=DIRECTION('ref_axis',(4.03736400342214E-14,-0.707106781186522,-0.707106781186573)) ;
#39845=DIRECTION('center_axis',(-0.0989489060816206,-0.703636665469235,
0.70363666546918)) ;
#39846=DIRECTION('ref_axis',(4.03736400342214E-14,-0.707106781186522,-0.707106781186573)) ;
#39847=DIRECTION('center_axis',(0.0914824783325312,0.381078720623584,-0.92000541566125)) ;
#39848=DIRECTION('ref_axis',(0.995806686138498,-0.0350088288095578,0.084518789314833)) ;
#39849=DIRECTION('',(-0.0914824783325312,-0.381078720623584,0.92000541566125)) ;
#39850=DIRECTION('center_axis',(-0.0989489060816133,-2.16674034761706E-15,
0.995092515289534)) ;
#39851=DIRECTION('ref_axis',(4.89166851579873E-15,-1.,-1.67265659768364E-15)) ;
#39852=DIRECTION('center_axis',(-0.0989489060816133,-2.16674034761706E-15,
0.995092515289534)) ;
#39853=DIRECTION('ref_axis',(4.89166851579873E-15,-1.,-1.67265659768364E-15)) ;
#39854=DIRECTION('center_axis',(0.0914824783325243,-0.381078720623587,-0.92000541566125)) ;
#39855=DIRECTION('ref_axis',(0.995806686138499,0.0350088288095554,0.0845187893148264)) ;
#39856=DIRECTION('',(-0.0914824783325243,0.381078720623587,0.92000541566125)) ;
#39857=DIRECTION('center_axis',(-0.0989489060815945,0.703636665469201,0.703636665469218)) ;
#39858=DIRECTION('ref_axis',(-2.16463014431357E-14,-0.707106781186558,0.707106781186537)) ;
#39859=DIRECTION('center_axis',(-0.0989489060815945,0.703636665469201,0.703636665469218)) ;
#39860=DIRECTION('ref_axis',(-2.16463014431357E-14,-0.707106781186558,0.707106781186537)) ;
#39861=DIRECTION('center_axis',(0.0914824783325312,-0.92000541566125,-0.381078720623584)) ;
#39862=DIRECTION('ref_axis',(0.995806686138498,0.0845187893148329,0.0350088288095578)) ;
#39863=DIRECTION('',(-0.0914824783325312,0.92000541566125,0.381078720623584)) ;
#39864=DIRECTION('center_axis',(-0.0989489060816085,0.995092515289535,-6.33274941053119E-14)) ;
#39865=DIRECTION('ref_axis',(-1.32208702071803E-14,6.23146444576098E-14,
1.)) ;
#39866=DIRECTION('center_axis',(-0.0989489060816085,0.995092515289535,-6.33274941053119E-14)) ;
#39867=DIRECTION('ref_axis',(-1.32208702071803E-14,6.23146444576098E-14,
1.)) ;
#39868=DIRECTION('center_axis',(0.0914824783325252,-0.920005415661246,0.381078720623595)) ;
#39869=DIRECTION('ref_axis',(0.995806686138499,0.084518789314827,-0.0350088288095565)) ;
#39870=DIRECTION('',(-0.0914824783325252,0.920005415661246,-0.381078720623595)) ;
#39871=DIRECTION('center_axis',(-0.098948906081588,0.703636665469212,-0.703636665469208)) ;
#39872=DIRECTION('ref_axis',(-3.98443775390689E-14,0.707106781186543,0.707106781186552)) ;
#39873=DIRECTION('center_axis',(-0.098948906081588,0.703636665469212,-0.703636665469208)) ;
#39874=DIRECTION('ref_axis',(-3.98443775390689E-14,0.707106781186543,0.707106781186552)) ;
#39875=DIRECTION('center_axis',(0.0914824783325244,-0.381078720623584,0.920005415661252)) ;
#39876=DIRECTION('ref_axis',(0.995806686138499,0.0350088288095551,-0.0845187893148267)) ;
#39877=DIRECTION('',(-0.0914824783325244,0.381078720623583,-0.920005415661251)) ;
#39878=DIRECTION('center_axis',(-0.0989489060816109,-4.35802109972033E-14,
-0.995092515289535)) ;
#39879=DIRECTION('ref_axis',(1.24831103654534E-14,1.,-4.50601525070747E-14)) ;
#39880=DIRECTION('center_axis',(-0.0989489060816109,-4.35802109972033E-14,
-0.995092515289535)) ;
#39881=DIRECTION('ref_axis',(1.24831103654534E-14,1.,-4.50601525070747E-14)) ;
#39882=DIRECTION('center_axis',(0.0914824783325321,0.381078720623592,0.920005415661247)) ;
#39883=DIRECTION('ref_axis',(0.995806686138498,-0.0350088288095588,-0.0845187893148334)) ;
#39884=DIRECTION('',(-0.0914824783325321,-0.381078720623592,-0.920005415661247)) ;
#39885=DIRECTION('center_axis',(-0.0989489060816214,-0.703636665469203,
-0.703636665469212)) ;
#39886=DIRECTION('ref_axis',(2.32073584995436E-14,0.707106781186551,-0.707106781186544)) ;
#39887=DIRECTION('center_axis',(-0.0989489060816214,-0.703636665469203,
-0.703636665469212)) ;
#39888=DIRECTION('ref_axis',(2.32073584995436E-14,0.707106781186551,-0.707106781186544)) ;
#39889=DIRECTION('center_axis',(0.0914824783325256,0.920005415661251,0.381078720623585)) ;
#39890=DIRECTION('ref_axis',(0.995806686138499,-0.0845187893148278,-0.0350088288095557)) ;
#39891=DIRECTION('',(-0.0914824783325256,-0.92000541566125,-0.381078720623585)) ;
#39892=DIRECTION('center_axis',(-0.0989489060816082,-0.995092515289535,
5.17051833170949E-14)) ;
#39893=DIRECTION('ref_axis',(1.83370743269828E-15,-5.20962696932553E-14,
-1.)) ;
#39894=DIRECTION('center_axis',(-0.0989489060816082,-0.995092515289535,
5.17051833170949E-14)) ;
#39895=DIRECTION('ref_axis',(1.83370743269828E-15,-5.20962696932553E-14,
-1.)) ;
#39896=DIRECTION('center_axis',(0.0914824783325307,0.920005415661251,-0.381078720623582)) ;
#39897=DIRECTION('ref_axis',(0.995806686138498,-0.0845187893148325,0.0350088288095574)) ;
#39898=DIRECTION('',(-0.0914824783325307,-0.920005415661251,0.381078720623582)) ;
#39899=DIRECTION('center_axis',(-0.0989489060815945,-0.703636665469239,
0.70363666546918)) ;
#39900=DIRECTION('ref_axis',(-3.59845035845265E-14,-0.707106781186516,-0.707106781186579)) ;
#39901=DIRECTION('center_axis',(-0.0989489060815945,-0.703636665469239,
0.70363666546918)) ;
#39902=DIRECTION('ref_axis',(-3.59845035845265E-14,-0.707106781186516,-0.707106781186579)) ;
#39903=DIRECTION('center_axis',(0.0914824783325255,0.381078720623585,-0.920005415661251)) ;
#39904=DIRECTION('ref_axis',(0.995806686138499,-0.0350088288095557,0.0845187893148276)) ;
#39905=DIRECTION('',(-0.0914824783325255,-0.381078720623585,0.920005415661251)) ;
#39906=DIRECTION('center_axis',(-0.0989489060816109,0.,0.995092515289535)) ;
#39907=DIRECTION('ref_axis',(1.39853604779557E-14,-1.,1.3953283963098E-15)) ;
#39908=DIRECTION('center_axis',(-0.0989489060816109,0.,0.995092515289535)) ;
#39909=DIRECTION('ref_axis',(1.39853604779557E-14,-1.,1.3953283963098E-15)) ;
#39910=DIRECTION('center_axis',(0.0914824783325243,-0.381078720623587,-0.92000541566125)) ;
#39911=DIRECTION('ref_axis',(0.995806686138499,0.0350088288095554,0.0845187893148264)) ;
#39912=DIRECTION('',(-0.0914824783325243,0.381078720623587,0.92000541566125)) ;
#39913=DIRECTION('center_axis',(-0.0989489060815945,0.7036366654692,0.703636665469218)) ;
#39914=DIRECTION('ref_axis',(-2.16195710140876E-14,-0.707106781186558,0.707106781186537)) ;
#39915=DIRECTION('center_axis',(-0.0989489060815945,0.7036366654692,0.703636665469218)) ;
#39916=DIRECTION('ref_axis',(-2.16195710140876E-14,-0.707106781186558,0.707106781186537)) ;
#39917=DIRECTION('center_axis',(0.0914824783325312,-0.92000541566125,-0.381078720623584)) ;
#39918=DIRECTION('ref_axis',(0.995806686138498,0.0845187893148329,0.0350088288095578)) ;
#39919=DIRECTION('',(-0.0914824783325312,0.92000541566125,0.381078720623584)) ;
#39920=DIRECTION('center_axis',(-0.0989489060816096,0.995092515289535,-6.26465533084806E-14)) ;
#39921=DIRECTION('ref_axis',(-1.0510404701705E-14,6.19317310614961E-14,
1.)) ;
#39922=DIRECTION('center_axis',(-0.0989489060816096,0.995092515289535,-6.26465533084806E-14)) ;
#39923=DIRECTION('ref_axis',(-1.0510404701705E-14,6.19317310614961E-14,
1.)) ;
#39924=DIRECTION('center_axis',(0.0914824783325252,-0.920005415661246,0.381078720623595)) ;
#39925=DIRECTION('ref_axis',(0.995806686138499,0.084518789314827,-0.0350088288095565)) ;
#39926=DIRECTION('',(-0.0914824783325252,0.920005415661247,-0.381078720623595)) ;
#39927=DIRECTION('center_axis',(-0.0989489060816214,0.703636665469211,-0.703636665469204)) ;
#39928=DIRECTION('ref_axis',(4.14909719684307E-14,0.707106781186547,0.707106781186548)) ;
#39929=DIRECTION('center_axis',(-0.0989489060816214,0.703636665469211,-0.703636665469204)) ;
#39930=DIRECTION('ref_axis',(4.14909719684307E-14,0.707106781186547,0.707106781186548)) ;
#39931=DIRECTION('center_axis',(0.0914824783325302,-0.381078720623583,0.920005415661251)) ;
#39932=DIRECTION('ref_axis',(0.995806686138499,0.0350088288095573,-0.084518789314832)) ;
#39933=DIRECTION('',(-0.0914824783325301,0.381078720623583,-0.920005415661251)) ;
#39934=DIRECTION('center_axis',(-0.0989489060815886,-4.14134706495869E-14,
-0.995092515289537)) ;
#39935=DIRECTION('ref_axis',(-5.62996296610662E-14,1.,-3.60112340135734E-14)) ;
#39936=DIRECTION('center_axis',(-0.0989489060815886,-4.14134706495869E-14,
-0.995092515289537)) ;
#39937=DIRECTION('ref_axis',(-5.62996296610662E-14,1.,-3.60112340135734E-14)) ;
#39938=DIRECTION('center_axis',(0.0914824783325264,0.381078720623592,0.920005415661248)) ;
#39939=DIRECTION('ref_axis',(0.995806686138499,-0.0350088288095566,-0.0845187893148281)) ;
#39940=DIRECTION('',(-0.0914824783325264,-0.381078720623592,-0.920005415661248)) ;
#39941=DIRECTION('center_axis',(-0.0989489060815706,-0.703636665469207,
-0.703636665469215)) ;
#39942=DIRECTION('ref_axis',(-8.51150321748982E-14,0.707106781186557,-0.707106781186538)) ;
#39943=DIRECTION('center_axis',(-0.0989489060815706,-0.703636665469207,
-0.703636665469215)) ;
#39944=DIRECTION('ref_axis',(-8.51150321748982E-14,0.707106781186557,-0.707106781186538)) ;
#39945=DIRECTION('center_axis',(0.0914824783325249,0.920005415661252,0.381078720623582)) ;
#39946=DIRECTION('ref_axis',(0.995806686138499,-0.0845187893148272,-0.0350088288095551)) ;
#39947=DIRECTION('',(-0.0914824783325248,-0.920005415661252,-0.381078720623582)) ;
#39948=DIRECTION('center_axis',(-0.098948906081608,-0.995092515289535,5.73229448909532E-14)) ;
#39949=DIRECTION('ref_axis',(3.14349845605419E-15,-5.7904791925403E-14,
-1.)) ;
#39950=DIRECTION('center_axis',(-0.098948906081608,-0.995092515289535,5.73229448909532E-14)) ;
#39951=DIRECTION('ref_axis',(3.14349845605419E-15,-5.7904791925403E-14,
-1.)) ;
#39952=DIRECTION('center_axis',(0.0914824783325315,0.92000541566125,-0.381078720623585)) ;
#39953=DIRECTION('ref_axis',(0.995806686138498,-0.0845187893148331,0.035008828809558)) ;
#39954=DIRECTION('',(-0.0914824783325315,-0.92000541566125,0.381078720623585)) ;
#39955=DIRECTION('center_axis',(-0.098948906081596,-0.703636665469235,0.703636665469183)) ;
#39956=DIRECTION('ref_axis',(-3.43379091551647E-14,-0.707106781186519,-0.707106781186576)) ;
#39957=DIRECTION('center_axis',(-0.098948906081596,-0.703636665469235,0.703636665469183)) ;
#39958=DIRECTION('ref_axis',(-3.43379091551647E-14,-0.707106781186519,-0.707106781186576)) ;
#39959=DIRECTION('center_axis',(0.0914824783325255,0.381078720623585,-0.920005415661251)) ;
#39960=DIRECTION('ref_axis',(0.995806686138499,-0.0350088288095557,0.0845187893148276)) ;
#39961=DIRECTION('',(-0.0914824783325255,-0.381078720623585,0.920005415661251)) ;
#39962=DIRECTION('center_axis',(-0.0989489060816133,0.,0.995092515289534)) ;
#39963=DIRECTION('ref_axis',(1.96896340368161E-14,-1.,1.9600087099505E-15)) ;
#39964=DIRECTION('center_axis',(-0.0989489060816133,0.,0.995092515289534)) ;
#39965=DIRECTION('ref_axis',(1.96896340368161E-14,-1.,1.9600087099505E-15)) ;
#39966=DIRECTION('center_axis',(0.09148247833253,-0.381078720623586,-0.92000541566125)) ;
#39967=DIRECTION('ref_axis',(0.995806686138499,0.0350088288095576,0.0845187893148318)) ;
#39968=DIRECTION('',(-0.09148247833253,0.381078720623586,0.92000541566125)) ;
#39969=DIRECTION('center_axis',(-0.0989489060816217,0.703636665469199,0.703636665469216)) ;
#39970=DIRECTION('ref_axis',(2.92377432927906E-14,-0.707106781186554,0.707106781186541)) ;
#39971=DIRECTION('center_axis',(-0.0989489060816217,0.703636665469199,0.703636665469216)) ;
#39972=DIRECTION('ref_axis',(2.92377432927906E-14,-0.707106781186554,0.707106781186541)) ;
#39973=DIRECTION('center_axis',(0.0914824783325255,-0.920005415661251,-0.381078720623585)) ;
#39974=DIRECTION('ref_axis',(0.995806686138499,0.0845187893148277,0.0350088288095557)) ;
#39975=DIRECTION('',(-0.0914824783325255,0.920005415661251,0.381078720623585)) ;
#39976=DIRECTION('center_axis',(-0.098948906081604,0.995092515289535,-6.1284671714818E-14)) ;
#39977=DIRECTION('ref_axis',(-9.02953893244136E-15,6.07114869754513E-14,
1.)) ;
#39978=DIRECTION('center_axis',(-0.098948906081604,0.995092515289535,-6.1284671714818E-14)) ;
#39979=DIRECTION('ref_axis',(-9.02953893244136E-15,6.07114869754513E-14,
1.)) ;
#39980=DIRECTION('center_axis',(0.0914824783325252,-0.920005415661246,0.381078720623595)) ;
#39981=DIRECTION('ref_axis',(0.995806686138499,0.084518789314827,-0.0350088288095565)) ;
#39982=DIRECTION('',(-0.0914824783325252,0.920005415661247,-0.381078720623595)) ;
#39983=DIRECTION('center_axis',(-0.0989489060816196,0.703636665469237,-0.703636665469178)) ;
#39984=DIRECTION('ref_axis',(4.05660991233678E-14,0.707106781186521,0.707106781186574)) ;
#39985=DIRECTION('center_axis',(-0.0989489060816196,0.703636665469237,-0.703636665469178)) ;
#39986=DIRECTION('ref_axis',(4.05660991233678E-14,0.707106781186521,0.707106781186574)) ;
#39987=DIRECTION('center_axis',(0.0914824783325311,-0.381078720623588,0.920005415661249)) ;
#39988=DIRECTION('ref_axis',(0.995806686138498,0.0350088288095581,-0.0845187893148327)) ;
#39989=DIRECTION('',(-0.0914824783325311,0.381078720623588,-0.920005415661249)) ;
#39990=DIRECTION('center_axis',(-0.0989489060816132,0.,-0.995092515289534)) ;
#39991=DIRECTION('ref_axis',(4.56021119560253E-15,1.,-4.86493808675064E-16)) ;
#39992=DIRECTION('center_axis',(-0.0989489060816132,0.,-0.995092515289534)) ;
#39993=DIRECTION('ref_axis',(4.56021119560253E-15,1.,-4.86493808675064E-16)) ;
#39994=DIRECTION('center_axis',(0.0914824783325254,0.381078720623588,0.92000541566125)) ;
#39995=DIRECTION('ref_axis',(0.995806686138499,-0.0350088288095559,-0.0845187893148274)) ;
#39996=DIRECTION('',(-0.0914824783325254,-0.381078720623588,-0.92000541566125)) ;
#39997=DIRECTION('center_axis',(-0.098948906081596,-0.7036366654692,-0.703636665469218)) ;
#39998=DIRECTION('ref_axis',(-2.07588511987394E-14,0.707106781186558,-0.707106781186537)) ;
#39999=DIRECTION('center_axis',(-0.098948906081596,-0.7036366654692,-0.703636665469218)) ;
#40000=DIRECTION('ref_axis',(-2.07588511987394E-14,0.707106781186558,-0.707106781186537)) ;
#40001=DIRECTION('center_axis',(0.0914824783325313,0.92000541566125,0.381078720623585)) ;
#40002=DIRECTION('ref_axis',(0.995806686138498,-0.084518789314833,-0.0350088288095579)) ;
#40003=DIRECTION('',(-0.0914824783325313,-0.92000541566125,-0.381078720623585)) ;
#40004=DIRECTION('center_axis',(-0.098948906081607,-0.995092515289535,4.78824082194844E-14)) ;
#40005=DIRECTION('ref_axis',(-1.56693775079845E-14,-4.65096100222067E-14,
-1.)) ;
#40006=DIRECTION('center_axis',(-0.098948906081607,-0.995092515289535,4.78824082194844E-14)) ;
#40007=DIRECTION('ref_axis',(-1.56693775079845E-14,-4.65096100222067E-14,
-1.)) ;
#40008=DIRECTION('center_axis',(0.091482478332525,0.920005415661252,-0.381078720623582)) ;
#40009=DIRECTION('ref_axis',(0.995806686138499,-0.0845187893148272,0.0350088288095552)) ;
#40010=DIRECTION('',(-0.091482478332525,-0.920005415661252,0.381078720623582)) ;
#40011=DIRECTION('center_axis',(-0.098948906081588,-0.703636665469236,0.703636665469183)) ;
#40012=DIRECTION('ref_axis',(-3.72408337497862E-14,-0.707106781186518,-0.707106781186577)) ;
#40013=DIRECTION('center_axis',(-0.098948906081588,-0.703636665469236,0.703636665469183)) ;
#40014=DIRECTION('ref_axis',(-3.72408337497862E-14,-0.707106781186518,-0.707106781186577)) ;
#40015=DIRECTION('center_axis',(0.0914824783325255,0.381078720623585,-0.920005415661251)) ;
#40016=DIRECTION('ref_axis',(0.995806686138499,-0.0350088288095557,0.0845187893148276)) ;
#40017=DIRECTION('',(-0.0914824783325255,-0.381078720623585,0.920005415661251)) ;
#40018=DIRECTION('center_axis',(-0.0989489060816109,0.,0.995092515289535)) ;
#40019=DIRECTION('ref_axis',(1.3953283963098E-14,-1.,1.3953283963098E-15)) ;
#40020=DIRECTION('center_axis',(-0.0989489060816109,0.,0.995092515289535)) ;
#40021=DIRECTION('ref_axis',(1.3953283963098E-14,-1.,1.3953283963098E-15)) ;
#40022=DIRECTION('center_axis',(0.09148247833253,-0.381078720623586,-0.92000541566125)) ;
#40023=DIRECTION('ref_axis',(0.995806686138499,0.0350088288095575,0.0845187893148318)) ;
#40024=DIRECTION('',(-0.09148247833253,0.381078720623586,0.92000541566125)) ;
#40025=DIRECTION('center_axis',(-0.0989489060816199,0.7036366654692,0.703636665469215)) ;
#40026=DIRECTION('ref_axis',(2.45438799519476E-14,-0.707106781186553,0.707106781186542)) ;
#40027=DIRECTION('center_axis',(-0.0989489060816199,0.7036366654692,0.703636665469215)) ;
#40028=DIRECTION('ref_axis',(2.45438799519476E-14,-0.707106781186553,0.707106781186542)) ;
#40029=DIRECTION('center_axis',(0.0914824783325255,-0.920005415661251,-0.381078720623585)) ;
#40030=DIRECTION('ref_axis',(0.995806686138499,0.0845187893148277,0.0350088288095557)) ;
#40031=DIRECTION('',(-0.0914824783325255,0.920005415661251,0.381078720623585)) ;
#40032=DIRECTION('center_axis',(-0.0989489060816096,0.995092515289535,-6.40084349021432E-14)) ;
#40033=DIRECTION('ref_axis',(4.3891364496947E-15,6.47517913260685E-14,1.)) ;
#40034=DIRECTION('center_axis',(-0.0989489060816096,0.995092515289535,-6.40084349021432E-14)) ;
#40035=DIRECTION('ref_axis',(4.3891364496947E-15,6.47517913260685E-14,1.)) ;
#40036=DIRECTION('center_axis',(0.091482478332531,-0.920005415661246,0.381078720623595)) ;
#40037=DIRECTION('ref_axis',(0.995806686138498,0.0845187893148323,-0.0350088288095587)) ;
#40038=DIRECTION('',(-0.0914824783325309,0.920005415661246,-0.381078720623595)) ;
#40039=DIRECTION('center_axis',(-0.098948906081595,0.703636665469237,-0.703636665469181)) ;
#40040=DIRECTION('ref_axis',(-3.42791022112591E-14,0.707106781186517,0.707106781186578)) ;
#40041=DIRECTION('center_axis',(-0.098948906081595,0.703636665469237,-0.703636665469181)) ;
#40042=DIRECTION('ref_axis',(-3.42791022112591E-14,0.707106781186517,0.707106781186578)) ;
#40043=DIRECTION('center_axis',(0.0914824783325254,-0.381078720623588,0.920005415661249)) ;
#40044=DIRECTION('ref_axis',(0.995806686138499,0.0350088288095559,-0.0845187893148274)) ;
#40045=DIRECTION('',(-0.0914824783325254,0.381078720623588,-0.920005415661249)) ;
#40046=DIRECTION('center_axis',(-0.0989489060816109,0.,-0.995092515289535)) ;
#40047=DIRECTION('ref_axis',(1.38784387617634E-14,1.,-1.37327579234513E-15)) ;
#40048=DIRECTION('center_axis',(-0.0989489060816109,0.,-0.995092515289535)) ;
#40049=DIRECTION('ref_axis',(1.38784387617634E-14,1.,-1.37327579234513E-15)) ;
#40050=DIRECTION('center_axis',(0.0914824783325254,0.381078720623587,0.92000541566125)) ;
#40051=DIRECTION('ref_axis',(0.995806686138499,-0.0350088288095559,-0.0845187893148275)) ;
#40052=DIRECTION('',(-0.0914824783325254,-0.381078720623587,-0.92000541566125)) ;
#40053=DIRECTION('center_axis',(-0.0989489060815934,-0.7036366654692,-0.703636665469219)) ;
#40054=DIRECTION('ref_axis',(-2.68052742494152E-14,0.707106781186559,-0.707106781186536)) ;
#40055=DIRECTION('center_axis',(-0.0989489060815934,-0.7036366654692,-0.703636665469219)) ;
#40056=DIRECTION('ref_axis',(-2.68052742494152E-14,0.707106781186559,-0.707106781186536)) ;
#40057=DIRECTION('center_axis',(0.0914824783325306,0.920005415661252,0.381078720623582)) ;
#40058=DIRECTION('ref_axis',(0.995806686138498,-0.0845187893148324,-0.0350088288095574)) ;
#40059=DIRECTION('',(-0.0914824783325306,-0.920005415661251,-0.381078720623582)) ;
#40060=DIRECTION('center_axis',(-0.0989489060816092,-0.995092515289535,
5.41347933480892E-14)) ;
#40061=DIRECTION('ref_axis',(-8.53235295214711E-15,-5.35470637298399E-14,
-1.)) ;
#40062=DIRECTION('center_axis',(-0.0989489060816092,-0.995092515289535,
5.41347933480892E-14)) ;
#40063=DIRECTION('ref_axis',(-8.53235295214711E-15,-5.35470637298399E-14,
-1.)) ;
#40064=DIRECTION('center_axis',(0.0914824783325257,0.92000541566125,-0.381078720623585)) ;
#40065=DIRECTION('ref_axis',(0.995806686138499,-0.0845187893148278,0.0350088288095558)) ;
#40066=DIRECTION('',(-0.0914824783325257,-0.92000541566125,0.381078720623585)) ;
#40067=DIRECTION('center_axis',(-0.0989489060816219,-0.703636665469235,
0.703636665469179)) ;
#40068=DIRECTION('ref_axis',(4.37042514936123E-14,-0.707106781186522,-0.707106781186573)) ;
#40069=DIRECTION('center_axis',(-0.0989489060816219,-0.703636665469235,
0.703636665469179)) ;
#40070=DIRECTION('ref_axis',(4.37042514936123E-14,-0.707106781186522,-0.707106781186573)) ;
#40071=DIRECTION('center_axis',(0.0914824783325312,0.381078720623585,-0.92000541566125)) ;
#40072=DIRECTION('ref_axis',(0.995806686138498,-0.0350088288095579,0.0845187893148329)) ;
#40073=DIRECTION('',(-0.0914824783325312,-0.381078720623585,0.92000541566125)) ;
#40074=DIRECTION('center_axis',(-0.0989489060816132,-2.16674034761706E-15,
0.995092515289534)) ;
#40075=DIRECTION('ref_axis',(4.81682331446411E-15,-1.,-1.67332485840984E-15)) ;
#40076=DIRECTION('center_axis',(-0.0989489060816132,-2.16674034761706E-15,
0.995092515289534)) ;
#40077=DIRECTION('ref_axis',(4.81682331446411E-15,-1.,-1.67332485840984E-15)) ;
#40078=DIRECTION('center_axis',(0.0914824783325243,-0.381078720623586,-0.92000541566125)) ;
#40079=DIRECTION('ref_axis',(0.995806686138499,0.0350088288095553,0.0845187893148265)) ;
#40080=DIRECTION('',(-0.0914824783325243,0.381078720623586,0.92000541566125)) ;
#40081=DIRECTION('center_axis',(-0.098948906081589,0.703636665469202,0.703636665469218)) ;
#40082=DIRECTION('ref_axis',(-3.5150514198226E-14,-0.707106781186558,0.707106781186537)) ;
#40083=DIRECTION('center_axis',(-0.098948906081589,0.703636665469202,0.703636665469218)) ;
#40084=DIRECTION('ref_axis',(-3.5150514198226E-14,-0.707106781186558,0.707106781186537)) ;
#40085=DIRECTION('center_axis',(0.0914824783325255,-0.920005415661251,-0.381078720623585)) ;
#40086=DIRECTION('ref_axis',(0.995806686138499,0.0845187893148277,0.0350088288095557)) ;
#40087=DIRECTION('',(-0.0914824783325255,0.920005415661251,0.381078720623585)) ;
#40088=DIRECTION('center_axis',(-0.0989489060816082,0.995092515289535,-6.24763181092728E-14)) ;
#40089=DIRECTION('ref_axis',(1.06387107611358E-15,6.29020456359414E-14,
1.)) ;
#40090=DIRECTION('center_axis',(-0.0989489060816082,0.995092515289535,-6.24763181092728E-14)) ;
#40091=DIRECTION('ref_axis',(1.06387107611358E-15,6.29020456359414E-14,
1.)) ;
#40092=DIRECTION('center_axis',(0.0914824783325307,-0.920005415661247,0.381078720623594)) ;
#40093=DIRECTION('ref_axis',(0.995806686138498,0.0845187893148321,-0.0350088288095585)) ;
#40094=DIRECTION('',(-0.0914824783325307,0.920005415661247,-0.381078720623594)) ;
#40095=DIRECTION('center_axis',(-0.098948906081595,0.703636665469237,-0.703636665469182)) ;
#40096=DIRECTION('ref_axis',(-3.37712240593455E-14,0.707106781186517,0.707106781186578)) ;
#40097=DIRECTION('center_axis',(-0.098948906081595,0.703636665469237,-0.703636665469182)) ;
#40098=DIRECTION('ref_axis',(-3.37712240593455E-14,0.707106781186517,0.707106781186578)) ;
#40099=DIRECTION('center_axis',(0.0914824783325255,-0.381078720623585,0.920005415661251)) ;
#40100=DIRECTION('ref_axis',(0.995806686138499,0.0350088288095557,-0.0845187893148276)) ;
#40101=DIRECTION('',(-0.0914824783325255,0.381078720623585,-0.92000541566125)) ;
#40102=DIRECTION('center_axis',(-0.0989489060816132,0.,-0.995092515289534)) ;
#40103=DIRECTION('ref_axis',(1.96468653503392E-14,1.,-1.9593404492243E-15)) ;
#40104=DIRECTION('center_axis',(-0.0989489060816132,0.,-0.995092515289534)) ;
#40105=DIRECTION('ref_axis',(1.96468653503392E-14,1.,-1.9593404492243E-15)) ;
#40106=DIRECTION('center_axis',(0.0914824783325311,0.381078720623587,0.920005415661249)) ;
#40107=DIRECTION('ref_axis',(0.995806686138498,-0.035008828809558,-0.0845187893148328)) ;
#40108=DIRECTION('',(-0.0914824783325311,-0.381078720623587,-0.920005415661249)) ;
#40109=DIRECTION('center_axis',(-0.09894890608162,-0.7036366654692,-0.703636665469215)) ;
#40110=DIRECTION('ref_axis',(2.22022943673357E-14,0.707106781186553,-0.707106781186542)) ;
#40111=DIRECTION('center_axis',(-0.09894890608162,-0.7036366654692,-0.703636665469215)) ;
#40112=DIRECTION('ref_axis',(2.22022943673357E-14,0.707106781186553,-0.707106781186542)) ;
#40113=DIRECTION('center_axis',(0.0914824783325253,0.920005415661251,0.381078720623584)) ;
#40114=DIRECTION('ref_axis',(0.995806686138499,-0.0845187893148275,-0.0350088288095555)) ;
#40115=DIRECTION('',(-0.0914824783325253,-0.920005415661251,-0.381078720623584)) ;
#40116=DIRECTION('center_axis',(-0.0989489060816036,-0.995092515289535,
5.34538525512579E-14)) ;
#40117=DIRECTION('ref_axis',(-8.23831823261823E-15,-5.28888269145309E-14,
-1.)) ;
#40118=DIRECTION('center_axis',(-0.0989489060816036,-0.995092515289535,
5.34538525512579E-14)) ;
#40119=DIRECTION('ref_axis',(-8.23831823261823E-15,-5.28888269145309E-14,
-1.)) ;
#40120=DIRECTION('center_axis',(0.0914824783325253,0.920005415661251,-0.381078720623584)) ;
#40121=DIRECTION('ref_axis',(0.995806686138499,-0.0845187893148275,0.0350088288095555)) ;
#40122=DIRECTION('',(-0.0914824783325253,-0.920005415661251,0.381078720623584)) ;
#40123=DIRECTION('center_axis',(-0.0989489060816199,-0.703636665469237,
0.703636665469178)) ;
#40124=DIRECTION('ref_axis',(3.98336853674502E-14,-0.70710678118652,-0.707106781186575)) ;
#40125=DIRECTION('center_axis',(-0.0989489060816199,-0.703636665469237,
0.703636665469178)) ;
#40126=DIRECTION('ref_axis',(3.98336853674502E-14,-0.70710678118652,-0.707106781186575)) ;
#40127=DIRECTION('center_axis',(0.0914824783325312,0.381078720623585,-0.92000541566125)) ;
#40128=DIRECTION('ref_axis',(0.995806686138498,-0.0350088288095579,0.0845187893148329)) ;
#40129=DIRECTION('',(-0.0914824783325312,-0.381078720623585,0.92000541566125)) ;
#40130=DIRECTION('center_axis',(-0.0989489060816132,0.,0.995092515289534)) ;
#40131=DIRECTION('ref_axis',(4.59228771046023E-15,-1.,4.67114247615206E-16)) ;
#40132=DIRECTION('center_axis',(-0.0989489060816132,0.,0.995092515289534)) ;
#40133=DIRECTION('ref_axis',(4.59228771046023E-15,-1.,4.67114247615206E-16)) ;
#40134=DIRECTION('center_axis',(0.0914824783325254,-0.381078720623587,-0.92000541566125)) ;
#40135=DIRECTION('ref_axis',(0.995806686138499,0.0350088288095559,0.0845187893148275)) ;
#40136=DIRECTION('',(-0.0914824783325254,0.381078720623587,0.92000541566125)) ;
#40137=DIRECTION('center_axis',(-0.098948906081595,0.703636665469222,0.703636665469197)) ;
#40138=DIRECTION('ref_axis',(-2.62172048103571E-14,-0.707106781186537,0.707106781186558)) ;
#40139=DIRECTION('center_axis',(-0.098948906081595,0.703636665469222,0.703636665469197)) ;
#40140=DIRECTION('ref_axis',(-2.62172048103571E-14,-0.707106781186537,0.707106781186558)) ;
#40141=DIRECTION('center_axis',(0.0914824783325306,-0.920005415661247,-0.381078720623593)) ;
#40142=DIRECTION('ref_axis',(0.995806686138498,0.084518789314832,0.0350088288095584)) ;
#40143=DIRECTION('',(-0.0914824783325306,0.920005415661247,0.381078720623593)) ;
#40144=DIRECTION('center_axis',(-0.0989489060816068,0.995092515289535,-5.43976630314667E-14)) ;
#40145=DIRECTION('ref_axis',(-1.57174922802709E-14,5.30879686109389E-14,
1.)) ;
#40146=DIRECTION('center_axis',(-0.0989489060816068,0.995092515289535,-5.43976630314667E-14)) ;
#40147=DIRECTION('ref_axis',(-1.57174922802709E-14,5.30879686109389E-14,
1.)) ;
#40148=DIRECTION('center_axis',(0.0914824783325249,-0.920005415661247,0.381078720623594)) ;
#40149=DIRECTION('ref_axis',(0.995806686138499,0.0845187893148268,-0.0350088288095563)) ;
#40150=DIRECTION('',(-0.0914824783325249,0.920005415661247,-0.381078720623594)) ;
#40151=DIRECTION('center_axis',(-0.0989489060815875,0.703636665469236,-0.703636665469183)) ;
#40152=DIRECTION('ref_axis',(-3.72889485220729E-14,0.707106781186518,0.707106781186577)) ;
#40153=DIRECTION('center_axis',(-0.0989489060815875,0.703636665469236,-0.703636665469183)) ;
#40154=DIRECTION('ref_axis',(-3.72889485220729E-14,0.707106781186518,0.707106781186577)) ;
#40155=DIRECTION('center_axis',(0.0914824783325255,-0.381078720623586,0.92000541566125)) ;
#40156=DIRECTION('ref_axis',(0.995806686138499,0.0350088288095557,-0.0845187893148276)) ;
#40157=DIRECTION('',(-0.0914824783325255,0.381078720623586,-0.92000541566125)) ;
#40158=DIRECTION('center_axis',(-0.0989489060816132,0.,-0.995092515289534)) ;
#40159=DIRECTION('ref_axis',(1.96094427496718E-14,1.,-1.9600087099505E-15)) ;
#40160=DIRECTION('center_axis',(-0.0989489060816132,0.,-0.995092515289534)) ;
#40161=DIRECTION('ref_axis',(1.96094427496718E-14,1.,-1.9600087099505E-15)) ;
#40162=DIRECTION('center_axis',(0.0914824783325311,0.381078720623587,0.920005415661249)) ;
#40163=DIRECTION('ref_axis',(0.995806686138498,-0.035008828809558,-0.0845187893148328)) ;
#40164=DIRECTION('',(-0.0914824783325311,-0.381078720623587,-0.920005415661249)) ;
#40165=DIRECTION('center_axis',(-0.0989489060816214,-0.7036366654692,-0.703636665469215)) ;
#40166=DIRECTION('ref_axis',(2.56772501435862E-14,0.707106781186553,-0.707106781186542)) ;
#40167=DIRECTION('center_axis',(-0.0989489060816214,-0.7036366654692,-0.703636665469215)) ;
#40168=DIRECTION('ref_axis',(2.56772501435862E-14,0.707106781186553,-0.707106781186542)) ;
#40169=DIRECTION('center_axis',(0.0914824783325253,0.920005415661251,0.381078720623584)) ;
#40170=DIRECTION('ref_axis',(0.995806686138499,-0.0845187893148275,-0.0350088288095555)) ;
#40171=DIRECTION('',(-0.0914824783325253,-0.920005415661251,-0.381078720623584)) ;
#40172=DIRECTION('center_axis',(-0.0989489060816092,-0.995092515289535,
5.22158889147184E-14)) ;
#40173=DIRECTION('ref_axis',(5.37281623866406E-15,-5.30144599310569E-14,
-1.)) ;
#40174=DIRECTION('center_axis',(-0.0989489060816092,-0.995092515289535,
5.22158889147184E-14)) ;
#40175=DIRECTION('ref_axis',(5.37281623866406E-15,-5.30144599310569E-14,
-1.)) ;
#40176=DIRECTION('center_axis',(0.0914824783325311,0.920005415661251,-0.381078720623584)) ;
#40177=DIRECTION('ref_axis',(0.995806686138498,-0.0845187893148328,0.0350088288095577)) ;
#40178=DIRECTION('',(-0.0914824783325311,-0.920005415661251,0.381078720623584)) ;
#40179=DIRECTION('center_axis',(-0.0989489060815955,-0.703636665469238,
0.70363666546918)) ;
#40180=DIRECTION('ref_axis',(-3.43699856700224E-14,-0.707106781186516,-0.707106781186579)) ;
#40181=DIRECTION('center_axis',(-0.0989489060815955,-0.703636665469238,
0.70363666546918)) ;
#40182=DIRECTION('ref_axis',(-3.43699856700224E-14,-0.707106781186516,-0.707106781186579)) ;
#40183=DIRECTION('center_axis',(0.0914824783325255,0.381078720623586,-0.92000541566125)) ;
#40184=DIRECTION('ref_axis',(0.995806686138499,-0.0350088288095557,0.0845187893148276)) ;
#40185=DIRECTION('',(-0.0914824783325255,-0.381078720623586,0.92000541566125)) ;
#40186=DIRECTION('center_axis',(-0.0989489060816109,0.,0.995092515289535)) ;
#40187=DIRECTION('ref_axis',(1.38944770191922E-14,-1.,1.3953283963098E-15)) ;
#40188=DIRECTION('center_axis',(-0.0989489060816109,0.,0.995092515289535)) ;
#40189=DIRECTION('ref_axis',(1.38944770191922E-14,-1.,1.3953283963098E-15)) ;
#40190=DIRECTION('center_axis',(0.0914824783325254,-0.381078720623587,-0.92000541566125)) ;
#40191=DIRECTION('ref_axis',(0.995806686138499,0.0350088288095558,0.0845187893148275)) ;
#40192=DIRECTION('',(-0.0914824783325254,0.381078720623587,0.92000541566125)) ;
#40193=DIRECTION('center_axis',(-0.0989489060815929,0.70363666546922,0.703636665469198)) ;
#40194=DIRECTION('ref_axis',(-3.11569880984424E-14,-0.707106781186539,0.707106781186557)) ;
#40195=DIRECTION('center_axis',(-0.0989489060815929,0.70363666546922,0.703636665469198)) ;
#40196=DIRECTION('ref_axis',(-3.11569880984424E-14,-0.707106781186539,0.707106781186557)) ;
#40197=DIRECTION('center_axis',(0.0914824783325306,-0.920005415661247,-0.381078720623593)) ;
#40198=DIRECTION('ref_axis',(0.995806686138498,0.084518789314832,0.0350088288095584)) ;
#40199=DIRECTION('',(-0.0914824783325306,0.920005415661247,0.381078720623593)) ;
#40200=DIRECTION('center_axis',(-0.0989489060816092,0.995092515289535,-5.6858556535412E-14)) ;
#40201=DIRECTION('ref_axis',(-1.00399491504588E-14,5.61579583871108E-14,
1.)) ;
#40202=DIRECTION('center_axis',(-0.0989489060816092,0.995092515289535,-5.6858556535412E-14)) ;
#40203=DIRECTION('ref_axis',(-1.00399491504588E-14,5.61579583871108E-14,
1.)) ;
#40204=DIRECTION('center_axis',(0.0914824783325249,-0.920005415661247,0.381078720623594)) ;
#40205=DIRECTION('ref_axis',(0.995806686138499,0.0845187893148267,-0.0350088288095562)) ;
#40206=DIRECTION('',(-0.0914824783325249,0.920005415661247,-0.381078720623594)) ;
#40207=DIRECTION('center_axis',(-0.0989489060816196,0.703636665469237,-0.703636665469178)) ;
#40208=DIRECTION('ref_axis',(4.13680119948102E-14,0.707106781186521,0.707106781186574)) ;
#40209=DIRECTION('center_axis',(-0.0989489060816196,0.703636665469237,-0.703636665469178)) ;
#40210=DIRECTION('ref_axis',(4.13680119948102E-14,0.707106781186521,0.707106781186574)) ;
#40211=DIRECTION('center_axis',(0.0914824783325312,-0.381078720623586,0.92000541566125)) ;
#40212=DIRECTION('ref_axis',(0.995806686138498,0.0350088288095579,-0.0845187893148329)) ;
#40213=DIRECTION('',(-0.0914824783325312,0.381078720623586,-0.92000541566125)) ;
#40214=DIRECTION('center_axis',(-0.0989489060816121,2.16674034761703E-15,
-0.995092515289534)) ;
#40215=DIRECTION('ref_axis',(1.91924480565218E-15,1.,1.95599914559329E-15)) ;
#40216=DIRECTION('center_axis',(-0.0989489060816121,2.16674034761703E-15,
-0.995092515289534)) ;
#40217=DIRECTION('ref_axis',(1.91924480565218E-15,1.,1.95599914559329E-15)) ;
#40218=DIRECTION('center_axis',(0.0914824783325254,0.381078720623587,0.92000541566125)) ;
#40219=DIRECTION('ref_axis',(0.995806686138499,-0.0350088288095558,-0.0845187893148275)) ;
#40220=DIRECTION('',(-0.0914824783325254,-0.381078720623587,-0.92000541566125)) ;
#40221=DIRECTION('center_axis',(-0.098948906081588,-0.703636665469202,-0.703636665469218)) ;
#40222=DIRECTION('ref_axis',(-4.05554069517479E-14,0.707106781186558,-0.707106781186537)) ;
#40223=DIRECTION('center_axis',(-0.098948906081588,-0.703636665469202,-0.703636665469218)) ;
#40224=DIRECTION('ref_axis',(-4.05554069517479E-14,0.707106781186558,-0.707106781186537)) ;
#40225=DIRECTION('center_axis',(0.0914824783325253,0.920005415661251,0.381078720623584)) ;
#40226=DIRECTION('ref_axis',(0.995806686138499,-0.0845187893148275,-0.0350088288095555)) ;
#40227=DIRECTION('',(-0.0914824783325253,-0.920005415661251,-0.381078720623584)) ;
#40228=DIRECTION('center_axis',(-0.0989489060816078,-0.995092515289535,
5.47694169028358E-14)) ;
#40229=DIRECTION('ref_axis',(1.61451791450403E-15,-5.51883120733919E-14,
-1.)) ;
#40230=DIRECTION('center_axis',(-0.0989489060816078,-0.995092515289535,
5.47694169028358E-14)) ;
#40231=DIRECTION('ref_axis',(1.61451791450403E-15,-5.51883120733919E-14,
-1.)) ;
#40232=DIRECTION('center_axis',(0.091482478332531,0.920005415661251,-0.381078720623584)) ;
#40233=DIRECTION('ref_axis',(0.995806686138498,-0.0845187893148328,0.0350088288095577)) ;
#40234=DIRECTION('',(-0.091482478332531,-0.920005415661251,0.381078720623584)) ;
#40235=DIRECTION('center_axis',(-0.098948906081596,-0.703636665469235,0.703636665469183)) ;
#40236=DIRECTION('ref_axis',(-3.3343537194576E-14,-0.707106781186519,-0.707106781186576)) ;
#40237=DIRECTION('center_axis',(-0.098948906081596,-0.703636665469235,0.703636665469183)) ;
#40238=DIRECTION('ref_axis',(-3.3343537194576E-14,-0.707106781186519,-0.707106781186576)) ;
#40239=DIRECTION('center_axis',(0.0914824783325255,0.381078720623586,-0.92000541566125)) ;
#40240=DIRECTION('ref_axis',(0.995806686138499,-0.0350088288095557,0.0845187893148276)) ;
#40241=DIRECTION('',(-0.0914824783325255,-0.381078720623586,0.92000541566125)) ;
#40242=DIRECTION('center_axis',(-0.0989489060816109,0.,0.995092515289535)) ;
#40243=DIRECTION('ref_axis',(1.3883784847573E-14,-1.,1.3953283963098E-15)) ;
#40244=DIRECTION('center_axis',(-0.0989489060816109,0.,0.995092515289535)) ;
#40245=DIRECTION('ref_axis',(1.3883784847573E-14,-1.,1.3953283963098E-15)) ;
#40246=DIRECTION('center_axis',(0.0914824783325311,-0.381078720623587,-0.920005415661249)) ;
#40247=DIRECTION('ref_axis',(0.995806686138498,0.035008828809558,0.0845187893148328)) ;
#40248=DIRECTION('',(-0.0914824783325311,0.381078720623587,0.920005415661249)) ;
#40249=DIRECTION('center_axis',(-0.0989489060816206,0.703636665469221,0.703636665469194)) ;
#40250=DIRECTION('ref_axis',(2.08016198852161E-14,-0.707106781186532,0.707106781186563)) ;
#40251=DIRECTION('center_axis',(-0.0989489060816206,0.703636665469221,0.703636665469194)) ;
#40252=DIRECTION('ref_axis',(2.08016198852161E-14,-0.707106781186532,0.707106781186563)) ;
#40253=DIRECTION('center_axis',(0.0914824783325249,-0.920005415661247,-0.381078720623594)) ;
#40254=DIRECTION('ref_axis',(0.995806686138499,0.0845187893148267,0.0350088288095562)) ;
#40255=DIRECTION('',(-0.0914824783325249,0.920005415661247,0.381078720623593)) ;
#40256=DIRECTION('center_axis',(-0.0989489060816038,0.995092515289535,-5.70287917346198E-14)) ;
#40257=DIRECTION('ref_axis',(-8.29712517652396E-15,5.64834013607711E-14,
1.)) ;
#40258=DIRECTION('center_axis',(-0.0989489060816038,0.995092515289535,-5.70287917346198E-14)) ;
#40259=DIRECTION('ref_axis',(-8.29712517652396E-15,5.64834013607711E-14,
1.)) ;
#40260=DIRECTION('center_axis',(0.0914824783325249,-0.920005415661247,0.381078720623594)) ;
#40261=DIRECTION('ref_axis',(0.995806686138499,0.0845187893148268,-0.0350088288095563)) ;
#40262=DIRECTION('',(-0.0914824783325249,0.920005415661247,-0.381078720623594)) ;
#40263=DIRECTION('center_axis',(-0.0989489060816196,0.703636665469236,-0.703636665469179)) ;
#40264=DIRECTION('ref_axis',(4.1063285103662E-14,0.707106781186522,0.707106781186573)) ;
#40265=DIRECTION('center_axis',(-0.0989489060816196,0.703636665469236,-0.703636665469179)) ;
#40266=DIRECTION('ref_axis',(4.1063285103662E-14,0.707106781186522,0.707106781186573)) ;
#40267=DIRECTION('center_axis',(0.0914824783325312,-0.381078720623586,0.92000541566125)) ;
#40268=DIRECTION('ref_axis',(0.995806686138498,0.035008828809558,-0.0845187893148329)) ;
#40269=DIRECTION('',(-0.0914824783325312,0.381078720623586,-0.92000541566125)) ;
#40270=DIRECTION('center_axis',(-0.0989489060816132,0.,-0.995092515289534)) ;
#40271=DIRECTION('ref_axis',(4.52813468074483E-15,1.,-4.24345561138278E-16)) ;
#40272=DIRECTION('center_axis',(-0.0989489060816132,0.,-0.995092515289534)) ;
#40273=DIRECTION('ref_axis',(4.52813468074483E-15,1.,-4.24345561138278E-16)) ;
#40274=DIRECTION('center_axis',(0.0914824783325254,0.381078720623587,0.92000541566125)) ;
#40275=DIRECTION('ref_axis',(0.995806686138499,-0.0350088288095558,-0.0845187893148275)) ;
#40276=DIRECTION('',(-0.0914824783325254,-0.381078720623587,-0.92000541566125)) ;
#40277=DIRECTION('center_axis',(-0.098948906081596,-0.7036366654692,-0.703636665469218)) ;
#40278=DIRECTION('ref_axis',(-2.08123120568356E-14,0.707106781186558,-0.707106781186537)) ;
#40279=DIRECTION('center_axis',(-0.098948906081596,-0.7036366654692,-0.703636665469218)) ;
#40280=DIRECTION('ref_axis',(-2.08123120568356E-14,0.707106781186558,-0.707106781186537)) ;
#40281=DIRECTION('center_axis',(0.091482478332531,0.920005415661251,0.381078720623584)) ;
#40282=DIRECTION('ref_axis',(0.995806686138498,-0.0845187893148328,-0.0350088288095577)) ;
#40283=DIRECTION('',(-0.091482478332531,-0.920005415661251,-0.381078720623583)) ;
#40284=DIRECTION('center_axis',(-0.098948906081607,-0.995092515289535,4.92442898131471E-14)) ;
#40285=DIRECTION('ref_axis',(-1.47070820622536E-14,-4.8002504484542E-14,
-1.)) ;
#40286=DIRECTION('center_axis',(-0.098948906081607,-0.995092515289535,4.92442898131471E-14)) ;
#40287=DIRECTION('ref_axis',(-1.47070820622536E-14,-4.8002504484542E-14,
-1.)) ;
#40288=DIRECTION('center_axis',(0.0914824783325253,0.920005415661251,-0.381078720623584)) ;
#40289=DIRECTION('ref_axis',(0.995806686138499,-0.0845187893148275,0.0350088288095555)) ;
#40290=DIRECTION('',(-0.0914824783325253,-0.920005415661251,0.381078720623584)) ;
#40291=DIRECTION('center_axis',(-0.098948906081588,-0.703636665469236,0.703636665469184)) ;
#40292=DIRECTION('ref_axis',(-3.79197866476075E-14,-0.707106781186519,-0.707106781186576)) ;
#40293=DIRECTION('center_axis',(-0.098948906081588,-0.703636665469236,0.703636665469184)) ;
#40294=DIRECTION('ref_axis',(-3.79197866476075E-14,-0.707106781186519,-0.707106781186576)) ;
#40295=DIRECTION('center_axis',(0.0914824783325255,0.381078720623586,-0.92000541566125)) ;
#40296=DIRECTION('ref_axis',(0.995806686138499,-0.0350088288095558,0.0845187893148276)) ;
#40297=DIRECTION('',(-0.0914824783325255,-0.381078720623586,0.92000541566125)) ;
#40298=DIRECTION('center_axis',(-0.0989489060816109,0.,0.995092515289535)) ;
#40299=DIRECTION('ref_axis',(1.38624005043345E-14,-1.,1.3953283963098E-15)) ;
#40300=DIRECTION('center_axis',(-0.0989489060816109,0.,0.995092515289535)) ;
#40301=DIRECTION('ref_axis',(1.38624005043345E-14,-1.,1.3953283963098E-15)) ;
#40302=DIRECTION('center_axis',(0.0914824783325311,-0.381078720623587,-0.920005415661249)) ;
#40303=DIRECTION('ref_axis',(0.995806686138498,0.035008828809558,0.0845187893148328)) ;
#40304=DIRECTION('',(-0.0914824783325311,0.381078720623587,0.920005415661249)) ;
#40305=DIRECTION('center_axis',(-0.0989489060816206,0.703636665469222,0.703636665469193)) ;
#40306=DIRECTION('ref_axis',(2.07588511987391E-14,-0.707106781186531,0.707106781186564)) ;
#40307=DIRECTION('center_axis',(-0.0989489060816206,0.703636665469222,0.703636665469193)) ;
#40308=DIRECTION('ref_axis',(2.07588511987391E-14,-0.707106781186531,0.707106781186564)) ;
#40309=DIRECTION('center_axis',(0.091482478332525,-0.920005415661247,-0.381078720623594)) ;
#40310=DIRECTION('ref_axis',(0.995806686138499,0.0845187893148268,0.0350088288095563)) ;
#40311=DIRECTION('',(-0.0914824783325249,0.920005415661247,0.381078720623594)) ;
#40312=DIRECTION('center_axis',(-0.0989489060816092,0.995092515289535,-5.69824744925375E-14)) ;
#40313=DIRECTION('ref_axis',(4.72059376989088E-15,5.77611158692693E-14,
1.)) ;
#40314=DIRECTION('center_axis',(-0.0989489060816092,0.995092515289535,-5.69824744925375E-14)) ;
#40315=DIRECTION('ref_axis',(4.72059376989088E-15,5.77611158692693E-14,
1.)) ;
#40316=DIRECTION('center_axis',(0.0914824783325307,-0.920005415661246,0.381078720623594)) ;
#40317=DIRECTION('ref_axis',(0.995806686138498,0.0845187893148321,-0.0350088288095585)) ;
#40318=DIRECTION('',(-0.0914824783325307,0.920005415661246,-0.381078720623594)) ;
#40319=DIRECTION('center_axis',(-0.0989489060815939,0.703636665469237,-0.703636665469181)) ;
#40320=DIRECTION('ref_axis',(-3.61716165878632E-14,0.707106781186517,0.707106781186578)) ;
#40321=DIRECTION('center_axis',(-0.0989489060815939,0.703636665469237,-0.703636665469181)) ;
#40322=DIRECTION('ref_axis',(-3.61716165878632E-14,0.707106781186517,0.707106781186578)) ;
#40323=DIRECTION('center_axis',(0.0914824783325254,-0.381078720623587,0.92000541566125)) ;
#40324=DIRECTION('ref_axis',(0.995806686138499,0.0350088288095558,-0.0845187893148275)) ;
#40325=DIRECTION('',(-0.0914824783325254,0.381078720623587,-0.92000541566125)) ;
#40326=DIRECTION('center_axis',(-0.0989489060816109,0.,-0.995092515289535)) ;
#40327=DIRECTION('ref_axis',(1.39800143921461E-14,1.,-1.41604447882206E-15)) ;
#40328=DIRECTION('center_axis',(-0.0989489060816109,0.,-0.995092515289535)) ;
#40329=DIRECTION('ref_axis',(1.39800143921461E-14,1.,-1.41604447882206E-15)) ;
#40330=DIRECTION('center_axis',(0.0914824783325254,0.381078720623587,0.92000541566125)) ;
#40331=DIRECTION('ref_axis',(0.995806686138499,-0.0350088288095559,-0.0845187893148275)) ;
#40332=DIRECTION('',(-0.0914824783325254,-0.381078720623587,-0.92000541566125)) ;
#40333=DIRECTION('center_axis',(-0.0989489060815942,-0.7036366654692,-0.703636665469218)) ;
#40334=DIRECTION('ref_axis',(-2.50624502754804E-14,0.707106781186558,-0.707106781186537)) ;
#40335=DIRECTION('center_axis',(-0.0989489060815942,-0.7036366654692,-0.703636665469218)) ;
#40336=DIRECTION('ref_axis',(-2.50624502754804E-14,0.707106781186558,-0.707106781186537)) ;
#40337=DIRECTION('center_axis',(0.0914824783325311,0.920005415661251,0.381078720623584)) ;
#40338=DIRECTION('ref_axis',(0.995806686138498,-0.0845187893148328,-0.0350088288095577)) ;
#40339=DIRECTION('',(-0.0914824783325311,-0.920005415661251,-0.381078720623584)) ;
#40340=DIRECTION('center_axis',(-0.0989489060816092,-0.995092515289535,
5.34538525512579E-14)) ;
#40341=DIRECTION('ref_axis',(-9.87956657617033E-15,-5.27197569508018E-14,
-1.)) ;
#40342=DIRECTION('center_axis',(-0.0989489060816092,-0.995092515289535,
5.34538525512579E-14)) ;
#40343=DIRECTION('ref_axis',(-9.87956657617033E-15,-5.27197569508018E-14,
-1.)) ;
#40344=DIRECTION('center_axis',(0.0914824783325254,0.920005415661251,-0.381078720623584)) ;
#40345=DIRECTION('ref_axis',(0.995806686138499,-0.0845187893148275,0.0350088288095555)) ;
#40346=DIRECTION('',(-0.0914824783325254,-0.920005415661251,0.381078720623584)) ;
#40347=DIRECTION('center_axis',(-0.0989489060816209,-0.703636665469237,
0.703636665469178)) ;
#40348=DIRECTION('ref_axis',(4.24104987276851E-14,-0.707106781186521,-0.707106781186574)) ;
#40349=DIRECTION('center_axis',(-0.0989489060816209,-0.703636665469237,
0.703636665469178)) ;
#40350=DIRECTION('ref_axis',(4.24104987276851E-14,-0.707106781186521,-0.707106781186574)) ;
#40351=DIRECTION('center_axis',(0.0914824783325311,0.381078720623587,-0.920005415661249)) ;
#40352=DIRECTION('ref_axis',(0.995806686138498,-0.035008828809558,0.0845187893148328)) ;
#40353=DIRECTION('',(-0.0914824783325311,-0.381078720623587,0.920005415661249)) ;
#40354=DIRECTION('center_axis',(-0.0989489060816121,-2.16674034761703E-15,
0.995092515289534)) ;
#40355=DIRECTION('ref_axis',(2.00478217860604E-15,-1.,-1.93595132380723E-15)) ;
#40356=DIRECTION('center_axis',(-0.0989489060816121,-2.16674034761703E-15,
0.995092515289534)) ;
#40357=DIRECTION('ref_axis',(2.00478217860604E-15,-1.,-1.93595132380723E-15)) ;
#40358=DIRECTION('center_axis',(0.0914824783325254,-0.381078720623587,-0.92000541566125)) ;
#40359=DIRECTION('ref_axis',(0.995806686138499,0.0350088288095559,0.0845187893148275)) ;
#40360=DIRECTION('',(-0.0914824783325254,0.381078720623587,0.92000541566125)) ;
#40361=DIRECTION('center_axis',(-0.0989489060815875,0.703636665469224,0.703636665469196)) ;
#40362=DIRECTION('ref_axis',(-4.46184321670556E-14,-0.707106781186537,0.707106781186558)) ;
#40363=DIRECTION('center_axis',(-0.0989489060815875,0.703636665469224,0.703636665469196)) ;
#40364=DIRECTION('ref_axis',(-4.46184321670556E-14,-0.707106781186537,0.707106781186558)) ;
#40365=DIRECTION('center_axis',(0.091482478332525,-0.920005415661247,-0.381078720623594)) ;
#40366=DIRECTION('ref_axis',(0.995806686138499,0.0845187893148268,0.0350088288095563)) ;
#40367=DIRECTION('',(-0.0914824783325249,0.920005415661247,0.381078720623594)) ;
#40368=DIRECTION('center_axis',(-0.091482478332525,0.920005415661247,0.381078720623594)) ;
#40369=DIRECTION('ref_axis',(0.995806686138499,0.0845187893148268,0.0350088288095563)) ;
#40370=DIRECTION('center_axis',(-0.091482478332525,0.920005415661247,0.381078720623594)) ;
#40371=DIRECTION('ref_axis',(-0.995806686138499,-0.0845187893148268,-0.0350088288095563)) ;
#40372=DIRECTION('center_axis',(0.,0.,1.)) ;
#40373=DIRECTION('ref_axis',(1.,0.,0.)) ;
#40374=DIRECTION('center_axis',(0.,0.,1.)) ;
#40375=DIRECTION('ref_axis',(1.,0.,0.)) ;
#40376=DIRECTION('',(0.,0.,-1.)) ;
#40377=DIRECTION('',(0.,0.,-1.)) ;
#40378=DIRECTION('center_axis',(0.,0.,-1.)) ;
#40379=DIRECTION('ref_axis',(1.,0.,0.)) ;
#40380=DIRECTION('center_axis',(0.,0.,1.)) ;
#40381=DIRECTION('ref_axis',(1.,0.,0.)) ;
#40382=DIRECTION('center_axis',(0.,0.,1.)) ;
#40383=DIRECTION('ref_axis',(1.,0.,0.)) ;
#40384=DIRECTION('',(0.,0.,1.)) ;
#40385=DIRECTION('center_axis',(0.,0.,-1.)) ;
#40386=DIRECTION('ref_axis',(1.,0.,0.)) ;
#40387=DIRECTION('center_axis',(0.,0.,-1.)) ;
#40388=DIRECTION('ref_axis',(-1.,0.,0.)) ;
#40389=DIRECTION('center_axis',(0.,0.,1.)) ;
#40390=DIRECTION('ref_axis',(1.,0.,0.)) ;
#40391=DIRECTION('center_axis',(0.948683298050515,0.,-0.316227766016835)) ;
#40392=DIRECTION('ref_axis',(0.316227766016835,0.,0.948683298050515)) ;
#40393=DIRECTION('',(-0.948683298050515,0.,0.316227766016834)) ;
#40394=DIRECTION('center_axis',(-0.948683298050515,0.,0.316227766016835)) ;
#40395=DIRECTION('ref_axis',(0.316227766016835,0.,0.948683298050515)) ;
#40396=DIRECTION('center_axis',(-0.948683298050515,0.,0.316227766016835)) ;
#40397=DIRECTION('ref_axis',(-0.316227766016835,0.,-0.948683298050515)) ;
#47520=CARTESIAN_POINT('',(0.,0.,0.)) ;
#47521=CARTESIAN_POINT('Origin',(21.5,0.,43.2)) ;
#47522=CARTESIAN_POINT('',(20.95,-6.73555739531044E-17,43.6)) ;
#47523=CARTESIAN_POINT('Origin',(21.5,0.,43.6)) ;
#47524=CARTESIAN_POINT('',(20.95,-6.73555739531044E-17,42.8)) ;
#47525=CARTESIAN_POINT('',(20.95,-6.73555739531044E-17,43.2)) ;
#47526=CARTESIAN_POINT('Origin',(21.5,0.,42.8)) ;
#47527=CARTESIAN_POINT('',(22.0291502622129,0.149999999999999,43.3279353866634)) ;
#47528=CARTESIAN_POINT('',(22.05,-5.24397723358717E-16,43.4943625562705)) ;
#47529=CARTESIAN_POINT('Ctrl Pts',(22.0291502622129,0.149999999999999,43.3279353866634)) ;
#47530=CARTESIAN_POINT('Ctrl Pts',(22.0291502622129,0.15,43.3482640855675)) ;
#47531=CARTESIAN_POINT('Ctrl Pts',(22.0302886323727,0.146138210109205,43.3699496533073)) ;
#47532=CARTESIAN_POINT('Ctrl Pts',(22.0342671466072,0.13084733724015,43.410330079765)) ;
#47533=CARTESIAN_POINT('Ctrl Pts',(22.0370500041276,0.119426507636106,43.4290336867825)) ;
#47534=CARTESIAN_POINT('Ctrl Pts',(22.0421962389769,0.0932418857328599,
43.4586176511119)) ;
#47535=CARTESIAN_POINT('Ctrl Pts',(22.0449278595246,0.0767918256322746,
43.4717830449028)) ;
#47536=CARTESIAN_POINT('Ctrl Pts',(22.0488606852484,0.0399412858806604,
43.4896777850851)) ;
#47537=CARTESIAN_POINT('Ctrl Pts',(22.05,0.019512600055463,43.4943625562705)) ;
#47538=CARTESIAN_POINT('Ctrl Pts',(22.05,1.28369537222284E-16,43.4943625562705)) ;
#47539=CARTESIAN_POINT('Ctrl Pts',(22.05,-1.07205910815367E-15,43.4943625562705)) ;
#47540=CARTESIAN_POINT('Ctrl Pts',(22.05,-0.019512600055464,43.4943625562705)) ;
#47541=CARTESIAN_POINT('Ctrl Pts',(22.0488606852484,-0.0399412858806645,
43.4896777850851)) ;
#47542=CARTESIAN_POINT('Ctrl Pts',(22.0449278595246,-0.0767918256322786,
43.4717830449028)) ;
#47543=CARTESIAN_POINT('Ctrl Pts',(22.0421962389769,-0.0932418857328599,
43.4586176511119)) ;
#47544=CARTESIAN_POINT('Ctrl Pts',(22.0370500041276,-0.119426507636106,
43.4290336867825)) ;
#47545=CARTESIAN_POINT('Ctrl Pts',(22.0342671466072,-0.13084733724015,43.410330079765)) ;
#47546=CARTESIAN_POINT('Ctrl Pts',(22.0302886323727,-0.146138210109205,
43.3699496533073)) ;
#47547=CARTESIAN_POINT('Ctrl Pts',(22.0291502622129,-0.15,43.3482640855675)) ;
#47548=CARTESIAN_POINT('Ctrl Pts',(22.0291502622129,-0.15,43.308519632144)) ;
#47549=CARTESIAN_POINT('Ctrl Pts',(22.0302085659904,-0.146426832233699,
43.2877474258495)) ;
#47550=CARTESIAN_POINT('Ctrl Pts',(22.0341811514524,-0.131196166457133,
43.2497089483429)) ;
#47551=CARTESIAN_POINT('Ctrl Pts',(22.037037832312,-0.119519687559714,43.2324442857003)) ;
#47552=CARTESIAN_POINT('Ctrl Pts',(22.0423222675757,-0.0925698332601531,
43.2058565502346)) ;
#47553=CARTESIAN_POINT('Ctrl Pts',(22.0450738363931,-0.075751613095341,
43.1946402298968)) ;
#47554=CARTESIAN_POINT('Ctrl Pts',(22.0489379804298,-0.0388701328861759,
43.1798339464663)) ;
#47555=CARTESIAN_POINT('Ctrl Pts',(22.05,-0.01880894404086,43.1762256790236)) ;
#47556=CARTESIAN_POINT('Ctrl Pts',(22.05,0.0188089440408599,43.1762256790237)) ;
#47557=CARTESIAN_POINT('Ctrl Pts',(22.0489379804298,0.038870132886171,43.1798339464663)) ;
#47558=CARTESIAN_POINT('Ctrl Pts',(22.0450738363931,0.0757516130953385,
43.1946402298968)) ;
#47559=CARTESIAN_POINT('Ctrl Pts',(22.0423222675757,0.0925698332601531,
43.2058565502346)) ;
#47560=CARTESIAN_POINT('Ctrl Pts',(22.037037832312,0.119519687559714,43.2324442857003)) ;
#47561=CARTESIAN_POINT('Ctrl Pts',(22.0341811514524,0.131196166457133,43.2497089483429)) ;
#47562=CARTESIAN_POINT('Ctrl Pts',(22.0302085659904,0.146426832233699,43.2877474258495)) ;
#47563=CARTESIAN_POINT('Ctrl Pts',(22.0291502622129,0.15,43.308519632144)) ;
#47564=CARTESIAN_POINT('Ctrl Pts',(22.0291502622129,0.15,43.3279353866634)) ;
#47565=CARTESIAN_POINT('Origin',(21.5,0.,43.2)) ;
#47566=CARTESIAN_POINT('',(21.25,-3.06161699786838E-17,42.8)) ;
#47567=CARTESIAN_POINT('Origin',(21.5,0.,42.8)) ;
#47568=CARTESIAN_POINT('',(21.25,3.06161699786838E-17,43.6)) ;
#47569=CARTESIAN_POINT('',(21.25,-3.06161699786838E-17,43.2)) ;
#47570=CARTESIAN_POINT('Origin',(21.5,0.,43.6)) ;
#47571=CARTESIAN_POINT('Origin',(21.5,0.,42.8)) ;
#47572=CARTESIAN_POINT('Origin',(21.5,0.,43.6)) ;
#47573=CARTESIAN_POINT('Origin',(22.375,0.,43.45)) ;
#47574=CARTESIAN_POINT('',(22.7500769823397,-1.83697019872103E-17,43.7414485500374)) ;
#47575=CARTESIAN_POINT('Origin',(22.8,0.,43.6)) ;
#47576=CARTESIAN_POINT('',(22.3250769823397,-1.83697019872103E-17,43.5914485500374)) ;
#47577=CARTESIAN_POINT('Origin',(22.8,0.,43.6)) ;
#47578=CARTESIAN_POINT('Origin',(22.75,0.,43.6)) ;
#47579=CARTESIAN_POINT('',(22.6,-9.79717439317883E-17,44.4)) ;
#47580=CARTESIAN_POINT('Origin',(22.6,0.,43.6)) ;
#47581=CARTESIAN_POINT('',(22.9,9.79717439317883E-17,44.4)) ;
#47582=CARTESIAN_POINT('',(22.75,-9.79717439317883E-17,44.4)) ;
#47583=CARTESIAN_POINT('Origin',(22.9,0.,43.6)) ;
#47584=CARTESIAN_POINT('Origin',(22.75,0.,43.6)) ;
#47585=CARTESIAN_POINT('',(22.9,-1.34711147906209E-16,44.7)) ;
#47586=CARTESIAN_POINT('Origin',(22.9,0.,43.6)) ;
#47587=CARTESIAN_POINT('',(22.6,-1.34711147906209E-16,44.7)) ;
#47588=CARTESIAN_POINT('',(22.75,-1.34711147906209E-16,44.7)) ;
#47589=CARTESIAN_POINT('Origin',(22.6,0.,43.6)) ;
#47590=CARTESIAN_POINT('Origin',(22.6,0.,43.6)) ;
#47591=CARTESIAN_POINT('Origin',(22.9,0.,43.6)) ;
#47592=CARTESIAN_POINT('Origin',(30.55,0.,43.6)) ;
#47593=CARTESIAN_POINT('',(30.549269378395,0.014786277360407,44.399863342079)) ;
#47594=CARTESIAN_POINT('',(30.4,-9.79717439317883E-17,44.4)) ;
#47595=CARTESIAN_POINT('Origin',(33.7324739562774,0.,43.6)) ;
#47596=CARTESIAN_POINT('',(30.4930138235359,0.576083171705783,44.155092946521)) ;
#47597=CARTESIAN_POINT('Ctrl Pts',(30.4930138235359,0.576083171705784,44.155092946521)) ;
#47598=CARTESIAN_POINT('Ctrl Pts',(30.4975561420248,0.544490046590428,44.1878807306833)) ;
#47599=CARTESIAN_POINT('Ctrl Pts',(30.4989740974443,0.508397435011936,44.2195320006755)) ;
#47600=CARTESIAN_POINT('Ctrl Pts',(30.5019483280108,0.417669414774168,44.2853318237253)) ;
#47601=CARTESIAN_POINT('Ctrl Pts',(30.5041008614886,0.360794086722511,44.3164679562894)) ;
#47602=CARTESIAN_POINT('Ctrl Pts',(30.5149996703933,0.251188800558993,44.3618679523262)) ;
#47603=CARTESIAN_POINT('Ctrl Pts',(30.5246605716675,0.189242972393476,44.3799145318681)) ;
#47604=CARTESIAN_POINT('Ctrl Pts',(30.5401014529422,0.0890575887576062,
44.3959153638972)) ;
#47605=CARTESIAN_POINT('Ctrl Pts',(30.5456292162213,0.0515279069685374,
44.3991841361479)) ;
#47606=CARTESIAN_POINT('Ctrl Pts',(30.549269378395,0.0147862773604065,44.399863342079)) ;
#47607=CARTESIAN_POINT('',(30.4367638235359,0.79986230391446,43.5851576694332)) ;
#47608=CARTESIAN_POINT('Ctrl Pts',(30.4367638235359,0.799862303914459,43.5851576694332)) ;
#47609=CARTESIAN_POINT('Ctrl Pts',(30.4413061420248,0.800707055427765,43.6306818469624)) ;
#47610=CARTESIAN_POINT('Ctrl Pts',(30.4427240974443,0.797566552674501,43.6785840050049)) ;
#47611=CARTESIAN_POINT('Ctrl Pts',(30.4456983280108,0.779939655400098,43.7892659044381)) ;
#47612=CARTESIAN_POINT('Ctrl Pts',(30.4478508614886,0.761739295728619,43.8514994050616)) ;
#47613=CARTESIAN_POINT('Ctrl Pts',(30.4587496703933,0.716339299691906,43.9611046912252)) ;
#47614=CARTESIAN_POINT('Ctrl Pts',(30.4684105716675,0.685297843301198,44.0176678651586)) ;
#47615=CARTESIAN_POINT('Ctrl Pts',(30.4838485444283,0.625781588850216,44.0998084508506)) ;
#47616=CARTESIAN_POINT('Ctrl Pts',(30.4893735852195,0.601568925505817,44.1286434771584)) ;
#47617=CARTESIAN_POINT('Ctrl Pts',(30.4930138235359,0.576083171705781,44.155092946521)) ;
#47618=CARTESIAN_POINT('',(30.4,0.749934102053461,43.3214343119168)) ;
#47619=CARTESIAN_POINT('Ctrl Pts',(30.4,0.749934102053461,43.3214343119168)) ;
#47620=CARTESIAN_POINT('Ctrl Pts',(30.405505133701,0.767659246796581,43.3691526457797)) ;
#47621=CARTESIAN_POINT('Ctrl Pts',(30.4137552132925,0.781567001849141,43.4211035732546)) ;
#47622=CARTESIAN_POINT('Ctrl Pts',(30.4275985444283,0.795912349908512,43.5109235398731)) ;
#47623=CARTESIAN_POINT('Ctrl Pts',(30.4331235852195,0.799180854104993,43.5484339209525)) ;
#47624=CARTESIAN_POINT('Ctrl Pts',(30.4367638235359,0.79986230391446,43.5851576694333)) ;
#47625=CARTESIAN_POINT('Origin',(30.4,0.,43.6)) ;
#47626=CARTESIAN_POINT('',(30.7,9.79717439317883E-17,44.4)) ;
#47627=CARTESIAN_POINT('',(30.55,-9.79717439317883E-17,44.4)) ;
#47628=CARTESIAN_POINT('Origin',(30.7,0.,43.6)) ;
#47629=CARTESIAN_POINT('Origin',(30.55,0.,43.6)) ;
#47630=CARTESIAN_POINT('',(30.7,-1.34711147906209E-16,44.7)) ;
#47631=CARTESIAN_POINT('Origin',(30.7,0.,43.6)) ;
#47632=CARTESIAN_POINT('',(30.4,-1.34711147906209E-16,44.7)) ;
#47633=CARTESIAN_POINT('',(30.55,-1.34711147906209E-16,44.7)) ;
#47634=CARTESIAN_POINT('Origin',(30.4,0.,43.6)) ;
#47635=CARTESIAN_POINT('Origin',(30.4,0.,43.6)) ;
#47636=CARTESIAN_POINT('',(30.4,0.0574025148547688,44.5385819298767)) ;
#47637=CARTESIAN_POINT('',(30.4,-0.141421356237311,44.0585786437627)) ;
#47638=CARTESIAN_POINT('',(30.4,0.887209576122323,43.5526899605521)) ;
#47639=CARTESIAN_POINT('Origin',(30.4,1.26862915010156,44.7313708498986)) ;
#47640=CARTESIAN_POINT('',(30.4,0.895119732372327,43.6282132329487)) ;
#47641=CARTESIAN_POINT('Origin',(30.4,0.8,43.6)) ;
#47642=CARTESIAN_POINT('',(30.4,0.696043110499698,44.2140880211392)) ;
#47643=CARTESIAN_POINT('Origin',(30.4,0.331370849898448,44.7313708498985)) ;
#47644=CARTESIAN_POINT('',(30.4,0.623636424388808,44.2920880323747)) ;
#47645=CARTESIAN_POINT('Origin',(30.4,0.565685424949239,44.1656854249492)) ;
#47646=CARTESIAN_POINT('Origin',(30.4,-1.47659662275146E-14,44.4)) ;
#47647=CARTESIAN_POINT('Origin',(30.7,0.,43.6)) ;
#47648=CARTESIAN_POINT('Origin',(30.4,3.05311331771918E-15,44.4)) ;
#47649=CARTESIAN_POINT('Origin',(30.4,3.05311331771918E-15,44.4)) ;
#47650=CARTESIAN_POINT('Origin',(30.34375,0.565685424949239,44.1656854249492)) ;
#47651=CARTESIAN_POINT('',(30.1944861227066,0.555190308577042,44.1761805413214)) ;
#47652=CARTESIAN_POINT('Origin',(30.34375,0.565685424949239,44.1656854249492)) ;
#47653=CARTESIAN_POINT('Origin',(30.34375,0.565685424949239,44.1656854249492)) ;
#47654=CARTESIAN_POINT('Origin',(30.2875,0.8,43.6)) ;
#47655=CARTESIAN_POINT('',(30.1381289970792,0.805251324321435,43.6126778183972)) ;
#47656=CARTESIAN_POINT('Origin',(30.2875,0.8,43.6)) ;
#47657=CARTESIAN_POINT('',(30.1382361227066,0.799999999999998,43.6148423359122)) ;
#47658=CARTESIAN_POINT('Origin',(30.2875,0.8,43.6)) ;
#47659=CARTESIAN_POINT('Origin',(30.2875,0.8,43.6)) ;
#47660=CARTESIAN_POINT('Origin',(30.23125,0.565685424949232,43.0343145750508)) ;
#47661=CARTESIAN_POINT('',(30.0819861227066,0.576180541321441,43.0448096914229)) ;
#47662=CARTESIAN_POINT('',(30.3805138772934,0.55519030857705,43.0238194586786)) ;
#47663=CARTESIAN_POINT('Origin',(30.23125,0.565685424949232,43.0343145750508)) ;
#47664=CARTESIAN_POINT('',(30.0818789970792,0.57836324334647,43.0395658993722)) ;
#47665=CARTESIAN_POINT('Origin',(30.23125,0.565685424949232,43.0343145750508)) ;
#47666=CARTESIAN_POINT('Origin',(30.23125,0.565685424949232,43.0343145750508)) ;
#47667=CARTESIAN_POINT('Origin',(30.175,-5.87929500492584E-15,42.8)) ;
#47668=CARTESIAN_POINT('',(30.0257361227066,0.0148423359122354,42.8)) ;
#47669=CARTESIAN_POINT('',(30.3242638772934,-0.014842335912247,42.8)) ;
#47670=CARTESIAN_POINT('Origin',(30.175,-5.88418203051333E-15,42.8)) ;
#47671=CARTESIAN_POINT('',(30.0291439534833,-5.89715721897613E-15,42.7649855216442)) ;
#47672=CARTESIAN_POINT('Origin',(30.175,-5.82867087928207E-15,42.8)) ;
#47673=CARTESIAN_POINT('',(30.175,-5.87929500492584E-15,42.65)) ;
#47674=CARTESIAN_POINT('Origin',(30.175,-5.87929500492584E-15,42.8)) ;
#47675=CARTESIAN_POINT('',(30.0256289970792,0.0126778183972199,42.7947486756786)) ;
#47676=CARTESIAN_POINT('Origin',(30.175,-5.82867087928207E-15,42.8)) ;
#47677=CARTESIAN_POINT('Origin',(30.175,-5.82867087928207E-15,42.8)) ;
#47678=CARTESIAN_POINT('Origin',(30.11875,-0.565685424949241,43.0343145750508)) ;
#47679=CARTESIAN_POINT('',(29.9694861227066,-0.555190308577047,43.0238194586786)) ;
#47680=CARTESIAN_POINT('',(30.2680138772934,-0.576180541321434,43.044809691423)) ;
#47681=CARTESIAN_POINT('Origin',(30.11875,-0.565685424949241,43.0343145750508)) ;
#47682=CARTESIAN_POINT('',(29.9693789970792,-0.560434100627805,43.0216367566535)) ;
#47683=CARTESIAN_POINT('Origin',(30.11875,-0.565685424949241,43.0343145750508)) ;
#47684=CARTESIAN_POINT('Origin',(30.11875,-0.565685424949241,43.0343145750508)) ;
#47685=CARTESIAN_POINT('Origin',(30.0625,-0.8,43.6)) ;
#47686=CARTESIAN_POINT('',(29.9132361227066,-0.799999999999999,43.5851576640878)) ;
#47687=CARTESIAN_POINT('',(30.2117638772934,-0.800000000000001,43.6148423359122)) ;
#47688=CARTESIAN_POINT('Origin',(30.0625,-0.8,43.6)) ;
#47689=CARTESIAN_POINT('',(29.9131289970792,-0.805251324321434,43.5873221816028)) ;
#47690=CARTESIAN_POINT('Origin',(30.0625,-0.8,43.6)) ;
#47691=CARTESIAN_POINT('Origin',(30.0625,-0.8,43.6)) ;
#47692=CARTESIAN_POINT('Origin',(30.00625,-0.565685424949238,44.1656854249492)) ;
#47693=CARTESIAN_POINT('',(29.8569861227066,-0.576180541321436,44.155190308577)) ;
#47694=CARTESIAN_POINT('',(30.1555138772934,-0.555190308577049,44.1761805413214)) ;
#47695=CARTESIAN_POINT('Origin',(30.00625,-0.565685424949238,44.1656854249492)) ;
#47696=CARTESIAN_POINT('',(29.8568789970792,-0.578363243346471,44.1604341006278)) ;
#47697=CARTESIAN_POINT('Origin',(30.00625,-0.565685424949238,44.1656854249492)) ;
#47698=CARTESIAN_POINT('Origin',(30.00625,-0.565685424949238,44.1656854249492)) ;
#47699=CARTESIAN_POINT('Origin',(29.95,8.62349420403445E-15,44.4)) ;
#47700=CARTESIAN_POINT('',(29.8007361227066,-0.0148423359122325,44.4)) ;
#47701=CARTESIAN_POINT('',(30.0992638772934,0.0148423359122498,44.4)) ;
#47702=CARTESIAN_POINT('Origin',(29.95,8.65973959207622E-15,44.4)) ;
#47703=CARTESIAN_POINT('',(29.8041439534833,8.60563198998416E-15,44.4350144783558)) ;
#47704=CARTESIAN_POINT('Origin',(29.95,8.65973959207622E-15,44.4)) ;
#47705=CARTESIAN_POINT('',(29.95,8.62349420403445E-15,44.55)) ;
#47706=CARTESIAN_POINT('Origin',(29.95,8.62349420403445E-15,44.4)) ;
#47707=CARTESIAN_POINT('',(29.8006289970792,-0.0126778183972173,44.4052513243214)) ;
#47708=CARTESIAN_POINT('Origin',(29.95,8.65973959207622E-15,44.4)) ;
#47709=CARTESIAN_POINT('Origin',(29.95,8.65973959207622E-15,44.4)) ;
#47710=CARTESIAN_POINT('Origin',(29.89375,0.565685424949243,44.1656854249492)) ;
#47711=CARTESIAN_POINT('',(29.7444861227066,0.555190308577048,44.1761805413214)) ;
#47712=CARTESIAN_POINT('',(30.0430138772934,0.576180541321437,44.155190308577)) ;
#47713=CARTESIAN_POINT('Origin',(29.89375,0.565685424949243,44.1656854249492)) ;
#47714=CARTESIAN_POINT('',(29.7443789970792,0.560434100627808,44.1783632433465)) ;
#47715=CARTESIAN_POINT('Origin',(29.89375,0.565685424949242,44.1656854249492)) ;
#47716=CARTESIAN_POINT('Origin',(29.89375,0.565685424949242,44.1656854249492)) ;
#47717=CARTESIAN_POINT('Origin',(29.8375,0.8,43.6)) ;
#47718=CARTESIAN_POINT('',(29.6882361227066,0.8,43.6148423359122)) ;
#47719=CARTESIAN_POINT('',(29.9867638772934,0.799999999999997,43.5851576640878)) ;
#47720=CARTESIAN_POINT('Origin',(29.8375,0.8,43.6)) ;
#47721=CARTESIAN_POINT('',(29.6881289970792,0.805251324321436,43.6126778183972)) ;
#47722=CARTESIAN_POINT('Origin',(29.8375,0.8,43.6)) ;
#47723=CARTESIAN_POINT('Origin',(29.8375,0.8,43.6)) ;
#47724=CARTESIAN_POINT('Origin',(29.78125,0.565685424949237,43.0343145750508)) ;
#47725=CARTESIAN_POINT('',(29.6319861227066,0.576180541321439,43.0448096914229)) ;
#47726=CARTESIAN_POINT('',(29.9305138772934,0.555190308577052,43.0238194586786)) ;
#47727=CARTESIAN_POINT('Origin',(29.78125,0.565685424949237,43.0343145750508)) ;
#47728=CARTESIAN_POINT('',(29.6318789970792,0.578363243346468,43.0395658993722)) ;
#47729=CARTESIAN_POINT('Origin',(29.78125,0.565685424949237,43.0343145750508)) ;
#47730=CARTESIAN_POINT('Origin',(29.78125,0.565685424949237,43.0343145750508)) ;
#47731=CARTESIAN_POINT('Origin',(29.725,9.90369018541372E-19,42.8)) ;
#47732=CARTESIAN_POINT('',(29.5757361227066,0.0148423359122408,42.8)) ;
#47733=CARTESIAN_POINT('',(29.8742638772934,-0.0148423359122408,42.8)) ;
#47734=CARTESIAN_POINT('Origin',(29.725,-5.55111512312578E-17,42.8)) ;
#47735=CARTESIAN_POINT('',(29.5791439534833,-1.68718450317509E-17,42.7649855216442)) ;
#47736=CARTESIAN_POINT('Origin',(29.725,5.55111512312578E-17,42.8)) ;
#47737=CARTESIAN_POINT('',(29.725,9.90369018541371E-19,42.65)) ;
#47738=CARTESIAN_POINT('Origin',(29.725,9.90369018541372E-19,42.8)) ;
#47739=CARTESIAN_POINT('',(29.5756289970792,0.0126778183972255,42.7947486756786)) ;
#47740=CARTESIAN_POINT('Origin',(29.725,5.55111512312578E-17,42.8)) ;
#47741=CARTESIAN_POINT('Origin',(29.725,5.55111512312578E-17,42.8)) ;
#47742=CARTESIAN_POINT('Origin',(29.66875,-0.565685424949237,43.0343145750508)) ;
#47743=CARTESIAN_POINT('',(29.5194861227066,-0.555190308577044,43.0238194586786)) ;
#47744=CARTESIAN_POINT('',(29.8180138772934,-0.576180541321431,43.044809691423)) ;
#47745=CARTESIAN_POINT('Origin',(29.66875,-0.565685424949237,43.0343145750508)) ;
#47746=CARTESIAN_POINT('',(29.5193789970792,-0.5604341006278,43.0216367566535)) ;
#47747=CARTESIAN_POINT('Origin',(29.66875,-0.565685424949237,43.0343145750508)) ;
#47748=CARTESIAN_POINT('Origin',(29.66875,-0.565685424949237,43.0343145750508)) ;
#47749=CARTESIAN_POINT('Origin',(29.6125,-0.8,43.6)) ;
#47750=CARTESIAN_POINT('',(29.4632361227066,-0.800000000000003,43.5851576640878)) ;
#47751=CARTESIAN_POINT('',(29.7617638772934,-0.800000000000005,43.6148423359123)) ;
#47752=CARTESIAN_POINT('Origin',(29.6125,-0.8,43.6)) ;
#47753=CARTESIAN_POINT('',(29.4631289970792,-0.805251324321435,43.5873221816028)) ;
#47754=CARTESIAN_POINT('Origin',(29.6125,-0.8,43.6)) ;
#47755=CARTESIAN_POINT('Origin',(29.6125,-0.8,43.6)) ;
#47756=CARTESIAN_POINT('Origin',(29.55625,-0.565685424949235,44.1656854249492)) ;
#47757=CARTESIAN_POINT('',(29.4069861227066,-0.57618054132143,44.155190308577)) ;
#47758=CARTESIAN_POINT('',(29.7055138772934,-0.555190308577039,44.1761805413214)) ;
#47759=CARTESIAN_POINT('Origin',(29.55625,-0.565685424949234,44.1656854249492)) ;
#47760=CARTESIAN_POINT('',(29.4068789970792,-0.578363243346462,44.1604341006278)) ;
#47761=CARTESIAN_POINT('Origin',(29.55625,-0.565685424949235,44.1656854249492)) ;
#47762=CARTESIAN_POINT('Origin',(29.55625,-0.565685424949235,44.1656854249492)) ;
#47763=CARTESIAN_POINT('Origin',(29.5,2.74320883009007E-15,44.4)) ;
#47764=CARTESIAN_POINT('',(29.3507361227066,-0.0148423359122402,44.4)) ;
#47765=CARTESIAN_POINT('',(29.6492638772934,0.0148423359122423,44.4)) ;
#47766=CARTESIAN_POINT('Origin',(29.5,2.83106871279415E-15,44.4)) ;
#47767=CARTESIAN_POINT('',(29.3541439534833,2.72534661603978E-15,44.4350144783558)) ;
#47768=CARTESIAN_POINT('Origin',(29.5,2.72004641033163E-15,44.4)) ;
#47769=CARTESIAN_POINT('',(29.5,2.74320883009007E-15,44.55)) ;
#47770=CARTESIAN_POINT('Origin',(29.5,2.74320883009007E-15,44.4)) ;
#47771=CARTESIAN_POINT('',(29.3506289970792,-0.0126778183972286,44.4052513243214)) ;
#47772=CARTESIAN_POINT('Origin',(29.5,2.72004641033163E-15,44.4)) ;
#47773=CARTESIAN_POINT('Origin',(29.5,2.72004641033163E-15,44.4)) ;
#47774=CARTESIAN_POINT('Origin',(29.44375,0.565685424949238,44.1656854249492)) ;
#47775=CARTESIAN_POINT('',(29.2944861227066,0.555190308577043,44.1761805413214)) ;
#47776=CARTESIAN_POINT('',(29.5930138772934,0.576180541321431,44.155190308577)) ;
#47777=CARTESIAN_POINT('Origin',(29.44375,0.565685424949238,44.1656854249492)) ;
#47778=CARTESIAN_POINT('',(29.2943789970792,0.560434100627805,44.1783632433465)) ;
#47779=CARTESIAN_POINT('Origin',(29.44375,0.565685424949238,44.1656854249492)) ;
#47780=CARTESIAN_POINT('Origin',(29.44375,0.565685424949238,44.1656854249492)) ;
#47781=CARTESIAN_POINT('Origin',(29.3875,0.8,43.6)) ;
#47782=CARTESIAN_POINT('',(29.2382361227066,0.799999999999999,43.6148423359122)) ;
#47783=CARTESIAN_POINT('',(29.5367638772934,0.799999999999997,43.5851576640878)) ;
#47784=CARTESIAN_POINT('Origin',(29.3875,0.8,43.6)) ;
#47785=CARTESIAN_POINT('',(29.2381289970792,0.805251324321435,43.6126778183972)) ;
#47786=CARTESIAN_POINT('Origin',(29.3875,0.8,43.6)) ;
#47787=CARTESIAN_POINT('Origin',(29.3875,0.8,43.6)) ;
#47788=CARTESIAN_POINT('Origin',(29.33125,0.565685424949233,43.0343145750508)) ;
#47789=CARTESIAN_POINT('',(29.1819861227066,0.576180541321431,43.044809691423)) ;
#47790=CARTESIAN_POINT('',(29.4805138772934,0.555190308577043,43.0238194586786)) ;
#47791=CARTESIAN_POINT('Origin',(29.33125,0.565685424949233,43.0343145750508)) ;
#47792=CARTESIAN_POINT('',(29.1818789970792,0.578363243346465,43.0395658993722)) ;
#47793=CARTESIAN_POINT('Origin',(29.33125,0.565685424949233,43.0343145750508)) ;
#47794=CARTESIAN_POINT('Origin',(29.33125,0.565685424949233,43.0343145750508)) ;
#47795=CARTESIAN_POINT('Origin',(29.275,-5.48740802919868E-15,42.8)) ;
#47796=CARTESIAN_POINT('',(29.1257361227066,0.0148423359122358,42.8)) ;
#47797=CARTESIAN_POINT('',(29.4242638772934,-0.0148423359122466,42.8)) ;
#47798=CARTESIAN_POINT('Origin',(29.275,-5.44009282066327E-15,42.8)) ;
#47799=CARTESIAN_POINT('',(29.1291439534833,-5.50527024324898E-15,42.7649855216442)) ;
#47800=CARTESIAN_POINT('Origin',(29.275,-5.38458166943201E-15,42.8)) ;
#47801=CARTESIAN_POINT('',(29.275,-5.48740802919868E-15,42.65)) ;
#47802=CARTESIAN_POINT('Origin',(29.275,-5.48740802919868E-15,42.8)) ;
#47803=CARTESIAN_POINT('',(29.1256289970792,0.012677818397221,42.7947486756786)) ;
#47804=CARTESIAN_POINT('Origin',(29.275,-5.38458166943201E-15,42.8)) ;
#47805=CARTESIAN_POINT('Origin',(29.275,-5.38458166943201E-15,42.8)) ;
#47806=CARTESIAN_POINT('Origin',(29.21875,-0.56568542494924,43.0343145750508)) ;
#47807=CARTESIAN_POINT('',(29.0694861227066,-0.555190308577045,43.0238194586786)) ;
#47808=CARTESIAN_POINT('',(29.3680138772934,-0.576180541321436,43.044809691423)) ;
#47809=CARTESIAN_POINT('Origin',(29.21875,-0.56568542494924,43.0343145750508)) ;
#47810=CARTESIAN_POINT('',(29.0693789970792,-0.560434100627806,43.0216367566535)) ;
#47811=CARTESIAN_POINT('Origin',(29.21875,-0.56568542494924,43.0343145750508)) ;
#47812=CARTESIAN_POINT('Origin',(29.21875,-0.56568542494924,43.0343145750508)) ;
#47813=CARTESIAN_POINT('Origin',(29.1625,-0.8,43.6)) ;
#47814=CARTESIAN_POINT('',(29.0132361227066,-0.8,43.5851576640878)) ;
#47815=CARTESIAN_POINT('',(29.3117638772934,-0.8,43.6148423359123)) ;
#47816=CARTESIAN_POINT('Origin',(29.1625,-0.8,43.6)) ;
#47817=CARTESIAN_POINT('',(29.0131289970792,-0.805251324321434,43.5873221816028)) ;
#47818=CARTESIAN_POINT('Origin',(29.1625,-0.8,43.6)) ;
#47819=CARTESIAN_POINT('Origin',(29.1625,-0.8,43.6)) ;
#47820=CARTESIAN_POINT('Origin',(29.10625,-0.565685424949239,44.1656854249492)) ;
#47821=CARTESIAN_POINT('',(28.9569861227066,-0.576180541321438,44.155190308577)) ;
#47822=CARTESIAN_POINT('',(29.2555138772934,-0.555190308577048,44.1761805413214)) ;
#47823=CARTESIAN_POINT('Origin',(29.10625,-0.565685424949239,44.1656854249492)) ;
#47824=CARTESIAN_POINT('',(28.9568789970792,-0.578363243346472,44.1604341006278)) ;
#47825=CARTESIAN_POINT('Origin',(29.10625,-0.565685424949239,44.1656854249492)) ;
#47826=CARTESIAN_POINT('Origin',(29.10625,-0.565685424949239,44.1656854249492)) ;
#47827=CARTESIAN_POINT('Origin',(29.05,-3.13707654385431E-15,44.4)) ;
#47828=CARTESIAN_POINT('',(28.9007361227066,-0.0148423359122443,44.4)) ;
#47829=CARTESIAN_POINT('',(29.1992638772934,0.014842335912238,44.4)) ;
#47830=CARTESIAN_POINT('Origin',(29.05,-3.05311331771918E-15,44.4)) ;
#47831=CARTESIAN_POINT('',(28.9041439534833,-3.1549387579046E-15,44.4350144783558)) ;
#47832=CARTESIAN_POINT('Origin',(29.05,-3.1641356201817E-15,44.4)) ;
#47833=CARTESIAN_POINT('',(29.05,-3.13707654385431E-15,44.55)) ;
#47834=CARTESIAN_POINT('Origin',(29.05,-3.13707654385431E-15,44.4)) ;
#47835=CARTESIAN_POINT('',(28.9006289970792,-0.0126778183972283,44.4052513243214)) ;
#47836=CARTESIAN_POINT('Origin',(29.05,-3.1641356201817E-15,44.4)) ;
#47837=CARTESIAN_POINT('Origin',(29.05,-3.1641356201817E-15,44.4)) ;
#47838=CARTESIAN_POINT('Origin',(28.99375,0.565685424949242,44.1656854249492)) ;
#47839=CARTESIAN_POINT('',(28.8444861227066,0.55519030857705,44.1761805413214)) ;
#47840=CARTESIAN_POINT('',(29.1430138772934,0.576180541321436,44.155190308577)) ;
#47841=CARTESIAN_POINT('Origin',(28.99375,0.565685424949242,44.1656854249492)) ;
#47842=CARTESIAN_POINT('',(28.8443789970792,0.560434100627807,44.1783632433465)) ;
#47843=CARTESIAN_POINT('Origin',(28.99375,0.565685424949242,44.1656854249492)) ;
#47844=CARTESIAN_POINT('Origin',(28.99375,0.565685424949242,44.1656854249492)) ;
#47845=CARTESIAN_POINT('Origin',(28.9375,0.8,43.6)) ;
#47846=CARTESIAN_POINT('',(28.7882361227066,0.799999999999998,43.6148423359122)) ;
#47847=CARTESIAN_POINT('',(29.0867638772934,0.799999999999999,43.5851576640878)) ;
#47848=CARTESIAN_POINT('Origin',(28.9375,0.8,43.6)) ;
#47849=CARTESIAN_POINT('',(28.7881289970792,0.805251324321436,43.6126778183972)) ;
#47850=CARTESIAN_POINT('Origin',(28.9375,0.8,43.6)) ;
#47851=CARTESIAN_POINT('Origin',(28.9375,0.8,43.6)) ;
#47852=CARTESIAN_POINT('Origin',(28.88125,0.565685424949237,43.0343145750508)) ;
#47853=CARTESIAN_POINT('',(28.7319861227066,0.576180541321439,43.0448096914229)) ;
#47854=CARTESIAN_POINT('',(29.0305138772934,0.555190308577051,43.0238194586786)) ;
#47855=CARTESIAN_POINT('Origin',(28.88125,0.565685424949237,43.0343145750508)) ;
#47856=CARTESIAN_POINT('',(28.7318789970792,0.578363243346472,43.0395658993722)) ;
#47857=CARTESIAN_POINT('Origin',(28.88125,0.565685424949237,43.0343145750508)) ;
#47858=CARTESIAN_POINT('Origin',(28.88125,0.565685424949237,43.0343145750508)) ;
#47859=CARTESIAN_POINT('Origin',(28.825,3.92877344745694E-16,42.8)) ;
#47860=CARTESIAN_POINT('',(28.6757361227066,0.0148423359122434,42.8)) ;
#47861=CARTESIAN_POINT('',(28.9742638772934,-0.0148423359122391,42.8)) ;
#47862=CARTESIAN_POINT('Origin',(28.825,4.44089209850063E-16,42.8)) ;
#47863=CARTESIAN_POINT('',(28.6791439534833,3.75015130695402E-16,42.7649855216442)) ;
#47864=CARTESIAN_POINT('Origin',(28.825,4.44089209850063E-16,42.8)) ;
#47865=CARTESIAN_POINT('',(28.825,3.92877344745694E-16,42.65)) ;
#47866=CARTESIAN_POINT('Origin',(28.825,3.92877344745694E-16,42.8)) ;
#47867=CARTESIAN_POINT('',(28.6756289970792,0.0126778183972335,42.7947486756786)) ;
#47868=CARTESIAN_POINT('Origin',(28.825,4.44089209850063E-16,42.8)) ;
#47869=CARTESIAN_POINT('Origin',(28.825,4.44089209850063E-16,42.8)) ;
#47870=CARTESIAN_POINT('Origin',(28.76875,-0.565685424949236,43.0343145750508)) ;
#47871=CARTESIAN_POINT('',(28.6194861227066,-0.555190308577039,43.0238194586786)) ;
#47872=CARTESIAN_POINT('',(28.9180138772934,-0.57618054132143,43.044809691423)) ;
#47873=CARTESIAN_POINT('Origin',(28.76875,-0.565685424949236,43.0343145750508)) ;
#47874=CARTESIAN_POINT('',(28.6193789970792,-0.560434100627803,43.0216367566535)) ;
#47875=CARTESIAN_POINT('Origin',(28.76875,-0.565685424949236,43.0343145750508)) ;
#47876=CARTESIAN_POINT('Origin',(28.76875,-0.565685424949236,43.0343145750508)) ;
#47877=CARTESIAN_POINT('Origin',(28.7125,-0.8,43.6)) ;
#47878=CARTESIAN_POINT('',(28.5632361227066,-0.800000000000002,43.5851576640878)) ;
#47879=CARTESIAN_POINT('',(28.8617638772934,-0.799999999999998,43.6148423359123)) ;
#47880=CARTESIAN_POINT('Origin',(28.7125,-0.8,43.6)) ;
#47881=CARTESIAN_POINT('',(28.5631289970792,-0.805251324321435,43.5873221816028)) ;
#47882=CARTESIAN_POINT('Origin',(28.7125,-0.8,43.6)) ;
#47883=CARTESIAN_POINT('Origin',(28.7125,-0.8,43.6)) ;
#47884=CARTESIAN_POINT('Origin',(28.65625,-0.565685424949235,44.1656854249492)) ;
#47885=CARTESIAN_POINT('',(28.5069861227066,-0.576180541321428,44.155190308577)) ;
#47886=CARTESIAN_POINT('',(28.8055138772934,-0.555190308577041,44.1761805413214)) ;
#47887=CARTESIAN_POINT('Origin',(28.65625,-0.565685424949235,44.1656854249492)) ;
#47888=CARTESIAN_POINT('',(28.5068789970792,-0.57836324334646,44.1604341006278)) ;
#47889=CARTESIAN_POINT('Origin',(28.65625,-0.565685424949235,44.1656854249492)) ;
#47890=CARTESIAN_POINT('Origin',(28.65625,-0.565685424949235,44.1656854249492)) ;
#47891=CARTESIAN_POINT('Origin',(28.6,2.35132185436292E-15,44.4)) ;
#47892=CARTESIAN_POINT('',(28.4507361227066,-0.0148423359122402,44.4)) ;
#47893=CARTESIAN_POINT('',(28.7492638772934,0.0148423359122414,44.4)) ;
#47894=CARTESIAN_POINT('Origin',(28.6,2.38697950294409E-15,44.4)) ;
#47895=CARTESIAN_POINT('',(28.4541439534833,2.33345964031263E-15,44.4350144783558)) ;
#47896=CARTESIAN_POINT('Origin',(28.6,2.27595720048157E-15,44.4)) ;
#47897=CARTESIAN_POINT('',(28.6,2.35132185436292E-15,44.55)) ;
#47898=CARTESIAN_POINT('Origin',(28.6,2.35132185436292E-15,44.4)) ;
#47899=CARTESIAN_POINT('',(28.4506289970792,-0.0126778183972291,44.4052513243214)) ;
#47900=CARTESIAN_POINT('Origin',(28.6,2.27595720048157E-15,44.4)) ;
#47901=CARTESIAN_POINT('Origin',(28.6,2.27595720048157E-15,44.4)) ;
#47902=CARTESIAN_POINT('Origin',(28.54375,0.565685424949238,44.1656854249492)) ;
#47903=CARTESIAN_POINT('',(28.3944861227066,0.555190308577043,44.1761805413214)) ;
#47904=CARTESIAN_POINT('',(28.6930138772934,0.57618054132143,44.155190308577)) ;
#47905=CARTESIAN_POINT('Origin',(28.54375,0.565685424949238,44.1656854249492)) ;
#47906=CARTESIAN_POINT('',(28.3943789970792,0.560434100627804,44.1783632433465)) ;
#47907=CARTESIAN_POINT('Origin',(28.54375,0.565685424949238,44.1656854249492)) ;
#47908=CARTESIAN_POINT('Origin',(28.54375,0.565685424949238,44.1656854249492)) ;
#47909=CARTESIAN_POINT('Origin',(28.4875,0.8,43.6)) ;
#47910=CARTESIAN_POINT('',(28.3382361227066,0.799999999999997,43.6148423359122)) ;
#47911=CARTESIAN_POINT('',(28.6367638772934,0.8,43.5851576640878)) ;
#47912=CARTESIAN_POINT('Origin',(28.4875,0.8,43.6)) ;
#47913=CARTESIAN_POINT('',(28.3381289970792,0.805251324321436,43.6126778183972)) ;
#47914=CARTESIAN_POINT('Origin',(28.4875,0.8,43.6)) ;
#47915=CARTESIAN_POINT('Origin',(28.4875,0.8,43.6)) ;
#47916=CARTESIAN_POINT('Origin',(28.43125,0.565685424949233,43.0343145750508)) ;
#47917=CARTESIAN_POINT('',(28.2819861227066,0.576180541321441,43.0448096914229)) ;
#47918=CARTESIAN_POINT('',(28.5805138772934,0.555190308577051,43.0238194586786)) ;
#47919=CARTESIAN_POINT('Origin',(28.43125,0.565685424949233,43.0343145750508)) ;
#47920=CARTESIAN_POINT('',(28.2818789970792,0.57836324334647,43.0395658993722)) ;
#47921=CARTESIAN_POINT('Origin',(28.43125,0.565685424949233,43.0343145750508)) ;
#47922=CARTESIAN_POINT('Origin',(28.43125,0.565685424949233,43.0343145750508)) ;
#47923=CARTESIAN_POINT('Origin',(28.375,-5.09552105347153E-15,42.8)) ;
#47924=CARTESIAN_POINT('',(28.2257361227066,0.0148423359122326,42.8)) ;
#47925=CARTESIAN_POINT('',(28.5242638772934,-0.0148423359122499,42.8)) ;
#47926=CARTESIAN_POINT('Origin',(28.375,-5.10702591327572E-15,42.8)) ;
#47927=CARTESIAN_POINT('',(28.2291439534833,-5.11338326752182E-15,42.7649855216442)) ;
#47928=CARTESIAN_POINT('Origin',(28.375,-5.10702591327572E-15,42.8)) ;
#47929=CARTESIAN_POINT('',(28.375,-5.09552105347153E-15,42.65)) ;
#47930=CARTESIAN_POINT('Origin',(28.375,-5.09552105347153E-15,42.8)) ;
#47931=CARTESIAN_POINT('',(28.2256289970792,0.0126778183972205,42.7947486756786)) ;
#47932=CARTESIAN_POINT('Origin',(28.375,-5.10702591327572E-15,42.8)) ;
#47933=CARTESIAN_POINT('Origin',(28.375,-5.10702591327572E-15,42.8)) ;
#47934=CARTESIAN_POINT('Origin',(28.31875,-0.56568542494924,43.0343145750508)) ;
#47935=CARTESIAN_POINT('',(28.1694861227066,-0.555190308577046,43.0238194586786)) ;
#47936=CARTESIAN_POINT('',(28.4680138772934,-0.576180541321434,43.044809691423)) ;
#47937=CARTESIAN_POINT('Origin',(28.31875,-0.56568542494924,43.0343145750508)) ;
#47938=CARTESIAN_POINT('',(28.1693789970792,-0.560434100627805,43.0216367566535)) ;
#47939=CARTESIAN_POINT('Origin',(28.31875,-0.56568542494924,43.0343145750508)) ;
#47940=CARTESIAN_POINT('Origin',(28.31875,-0.56568542494924,43.0343145750508)) ;
#47941=CARTESIAN_POINT('Origin',(28.2625,-0.8,43.6)) ;
#47942=CARTESIAN_POINT('',(28.1132361227066,-0.800000000000001,43.5851576640878)) ;
#47943=CARTESIAN_POINT('',(28.4117638772934,-0.799999999999999,43.6148423359122)) ;
#47944=CARTESIAN_POINT('Origin',(28.2625,-0.8,43.6)) ;
#47945=CARTESIAN_POINT('',(28.1131289970792,-0.805251324321435,43.5873221816028)) ;
#47946=CARTESIAN_POINT('Origin',(28.2625,-0.8,43.6)) ;
#47947=CARTESIAN_POINT('Origin',(28.2625,-0.8,43.6)) ;
#47948=CARTESIAN_POINT('Origin',(28.20625,-0.565685424949239,44.1656854249492)) ;
#47949=CARTESIAN_POINT('',(28.0569861227066,-0.576180541321436,44.155190308577)) ;
#47950=CARTESIAN_POINT('',(28.3555138772934,-0.55519030857705,44.1761805413214)) ;
#47951=CARTESIAN_POINT('Origin',(28.20625,-0.565685424949239,44.1656854249492)) ;
#47952=CARTESIAN_POINT('',(28.0568789970792,-0.578363243346472,44.1604341006278)) ;
#47953=CARTESIAN_POINT('Origin',(28.20625,-0.565685424949239,44.1656854249492)) ;
#47954=CARTESIAN_POINT('Origin',(28.20625,-0.565685424949239,44.1656854249492)) ;
#47955=CARTESIAN_POINT('Origin',(28.15,7.83972025258014E-15,44.4)) ;
#47956=CARTESIAN_POINT('',(28.0007361227066,-0.0148423359122333,44.4)) ;
#47957=CARTESIAN_POINT('',(28.2992638772934,0.014842335912249,44.4)) ;
#47958=CARTESIAN_POINT('Origin',(28.15,7.93809462606987E-15,44.4)) ;
#47959=CARTESIAN_POINT('',(28.0041439534833,7.82185803852985E-15,44.4350144783558)) ;
#47960=CARTESIAN_POINT('Origin',(28.15,7.88258347483861E-15,44.4)) ;
#47961=CARTESIAN_POINT('',(28.15,7.83972025258014E-15,44.55)) ;
#47962=CARTESIAN_POINT('Origin',(28.15,7.83972025258014E-15,44.4)) ;
#47963=CARTESIAN_POINT('',(28.0006289970792,-0.0126778183972181,44.4052513243214)) ;
#47964=CARTESIAN_POINT('Origin',(28.15,7.88258347483861E-15,44.4)) ;
#47965=CARTESIAN_POINT('Origin',(28.15,7.88258347483861E-15,44.4)) ;
#47966=CARTESIAN_POINT('Origin',(28.09375,0.565685424949242,44.1656854249492)) ;
#47967=CARTESIAN_POINT('',(27.9444861227066,0.555190308577047,44.1761805413214)) ;
#47968=CARTESIAN_POINT('',(28.2430138772934,0.576180541321437,44.155190308577)) ;
#47969=CARTESIAN_POINT('Origin',(28.09375,0.565685424949242,44.1656854249492)) ;
#47970=CARTESIAN_POINT('',(27.9443789970792,0.560434100627808,44.1783632433465)) ;
#47971=CARTESIAN_POINT('Origin',(28.09375,0.565685424949242,44.1656854249492)) ;
#47972=CARTESIAN_POINT('Origin',(28.09375,0.565685424949242,44.1656854249492)) ;
#47973=CARTESIAN_POINT('Origin',(28.0375,0.8,43.6)) ;
#47974=CARTESIAN_POINT('',(27.8882361227066,0.799999999999999,43.6148423359122)) ;
#47975=CARTESIAN_POINT('',(28.1867638772934,0.799999999999998,43.5851576640877)) ;
#47976=CARTESIAN_POINT('Origin',(28.0375,0.8,43.6)) ;
#47977=CARTESIAN_POINT('',(27.8881289970792,0.805251324321436,43.6126778183972)) ;
#47978=CARTESIAN_POINT('Origin',(28.0375,0.8,43.6)) ;
#47979=CARTESIAN_POINT('Origin',(28.0375,0.8,43.6)) ;
#47980=CARTESIAN_POINT('Origin',(27.98125,0.565685424949237,43.0343145750508)) ;
#47981=CARTESIAN_POINT('',(27.8319861227066,0.576180541321441,43.0448096914229)) ;
#47982=CARTESIAN_POINT('',(28.1305138772934,0.555190308577051,43.0238194586786)) ;
#47983=CARTESIAN_POINT('Origin',(27.98125,0.565685424949237,43.0343145750508)) ;
#47984=CARTESIAN_POINT('',(27.8318789970792,0.578363243346469,43.0395658993722)) ;
#47985=CARTESIAN_POINT('Origin',(27.98125,0.565685424949237,43.0343145750508)) ;
#47986=CARTESIAN_POINT('Origin',(27.98125,0.565685424949237,43.0343145750508)) ;
#47987=CARTESIAN_POINT('Origin',(27.925,7.84764320472847E-16,42.8)) ;
#47988=CARTESIAN_POINT('',(27.7757361227066,0.0148423359122439,42.8)) ;
#47989=CARTESIAN_POINT('',(28.0742638772934,-0.0148423359122386,42.8)) ;
#47990=CARTESIAN_POINT('Origin',(27.925,7.7715611723761E-16,42.8)) ;
#47991=CARTESIAN_POINT('',(27.7791439534833,7.66902106422555E-16,42.7649855216442)) ;
#47992=CARTESIAN_POINT('Origin',(27.925,8.32667268468867E-16,42.8)) ;
#47993=CARTESIAN_POINT('',(27.925,7.84764320472847E-16,42.65)) ;
#47994=CARTESIAN_POINT('Origin',(27.925,7.84764320472847E-16,42.8)) ;
#47995=CARTESIAN_POINT('',(27.7756289970792,0.0126778183972334,42.7947486756786)) ;
#47996=CARTESIAN_POINT('Origin',(27.925,8.32667268468867E-16,42.8)) ;
#47997=CARTESIAN_POINT('Origin',(27.925,8.32667268468867E-16,42.8)) ;
#47998=CARTESIAN_POINT('Origin',(27.86875,-0.565685424949236,43.0343145750508)) ;
#47999=CARTESIAN_POINT('',(27.7194861227066,-0.555190308577041,43.0238194586786)) ;
#48000=CARTESIAN_POINT('',(28.0180138772934,-0.576180541321428,43.044809691423)) ;
#48001=CARTESIAN_POINT('Origin',(27.86875,-0.565685424949236,43.0343145750508)) ;
#48002=CARTESIAN_POINT('',(27.7193789970792,-0.560434100627802,43.0216367566535)) ;
#48003=CARTESIAN_POINT('Origin',(27.86875,-0.565685424949236,43.0343145750508)) ;
#48004=CARTESIAN_POINT('Origin',(27.86875,-0.565685424949236,43.0343145750508)) ;
#48005=CARTESIAN_POINT('Origin',(27.8125,-0.8,43.6)) ;
#48006=CARTESIAN_POINT('',(27.6632361227066,-0.8,43.5851576640878)) ;
#48007=CARTESIAN_POINT('',(27.9617638772934,-0.8,43.6148423359123)) ;
#48008=CARTESIAN_POINT('Origin',(27.8125,-0.8,43.6)) ;
#48009=CARTESIAN_POINT('',(27.6631289970792,-0.805251324321434,43.5873221816028)) ;
#48010=CARTESIAN_POINT('Origin',(27.8125,-0.8,43.6)) ;
#48011=CARTESIAN_POINT('Origin',(27.8125,-0.8,43.6)) ;
#48012=CARTESIAN_POINT('Origin',(27.75625,-0.565685424949235,44.1656854249492)) ;
#48013=CARTESIAN_POINT('',(27.6069861227066,-0.576180541321429,44.1551903085771)) ;
#48014=CARTESIAN_POINT('',(27.9055138772934,-0.555190308577041,44.1761805413214)) ;
#48015=CARTESIAN_POINT('Origin',(27.75625,-0.565685424949235,44.1656854249492)) ;
#48016=CARTESIAN_POINT('',(27.6068789970792,-0.578363243346462,44.1604341006278)) ;
#48017=CARTESIAN_POINT('Origin',(27.75625,-0.565685424949235,44.1656854249492)) ;
#48018=CARTESIAN_POINT('Origin',(27.75625,-0.565685424949235,44.1656854249492)) ;
#48019=CARTESIAN_POINT('Origin',(27.7,1.95943487863577E-15,44.4)) ;
#48020=CARTESIAN_POINT('',(27.5507361227066,-0.0148423359122409,44.4)) ;
#48021=CARTESIAN_POINT('',(27.8492638772934,0.0148423359122416,44.4)) ;
#48022=CARTESIAN_POINT('Origin',(27.7,2.05391259555654E-15,44.4)) ;
#48023=CARTESIAN_POINT('',(27.5541439534833,1.94157266458547E-15,44.4350144783558)) ;
#48024=CARTESIAN_POINT('Origin',(27.7,1.94289029309402E-15,44.4)) ;
#48025=CARTESIAN_POINT('',(27.7,1.95943487863577E-15,44.55)) ;
#48026=CARTESIAN_POINT('Origin',(27.7,1.95943487863577E-15,44.4)) ;
#48027=CARTESIAN_POINT('',(27.5506289970792,-0.0126778183972306,44.4052513243214)) ;
#48028=CARTESIAN_POINT('Origin',(27.7,1.94289029309402E-15,44.4)) ;
#48029=CARTESIAN_POINT('Origin',(27.7,1.94289029309402E-15,44.4)) ;
#48030=CARTESIAN_POINT('Origin',(27.64375,0.565685424949238,44.1656854249492)) ;
#48031=CARTESIAN_POINT('',(27.4944861227066,0.555190308577042,44.1761805413214)) ;
#48032=CARTESIAN_POINT('',(27.7930138772934,0.576180541321432,44.155190308577)) ;
#48033=CARTESIAN_POINT('Origin',(27.64375,0.565685424949238,44.1656854249492)) ;
#48034=CARTESIAN_POINT('',(27.4943789970792,0.560434100627803,44.1783632433465)) ;
#48035=CARTESIAN_POINT('Origin',(27.64375,0.565685424949238,44.1656854249492)) ;
#48036=CARTESIAN_POINT('Origin',(27.64375,0.565685424949238,44.1656854249492)) ;
#48037=CARTESIAN_POINT('Origin',(27.5875,0.8,43.6)) ;
#48038=CARTESIAN_POINT('',(27.4382361227066,0.8,43.6148423359122)) ;
#48039=CARTESIAN_POINT('',(27.7367638772934,0.799999999999996,43.5851576640877)) ;
#48040=CARTESIAN_POINT('Origin',(27.5875,0.8,43.6)) ;
#48041=CARTESIAN_POINT('',(27.4381289970792,0.805251324321436,43.6126778183972)) ;
#48042=CARTESIAN_POINT('Origin',(27.5875,0.8,43.6)) ;
#48043=CARTESIAN_POINT('Origin',(27.5875,0.8,43.6)) ;
#48044=CARTESIAN_POINT('Origin',(27.53125,0.565685424949237,43.0343145750508)) ;
#48045=CARTESIAN_POINT('',(27.3819861227066,0.576180541321439,43.0448096914229)) ;
#48046=CARTESIAN_POINT('',(27.6805138772934,0.555190308577052,43.0238194586786)) ;
#48047=CARTESIAN_POINT('Origin',(27.53125,0.565685424949237,43.0343145750508)) ;
#48048=CARTESIAN_POINT('',(27.3818789970792,0.578363243346468,43.0395658993722)) ;
#48049=CARTESIAN_POINT('Origin',(27.53125,0.565685424949237,43.0343145750508)) ;
#48050=CARTESIAN_POINT('Origin',(27.53125,0.565685424949237,43.0343145750508)) ;
#48051=CARTESIAN_POINT('Origin',(27.475,-4.70363407774438E-15,42.8)) ;
#48052=CARTESIAN_POINT('',(27.3257361227066,0.0148423359122361,42.8)) ;
#48053=CARTESIAN_POINT('',(27.6242638772934,-0.0148423359122454,42.8)) ;
#48054=CARTESIAN_POINT('Origin',(27.475,-4.66293670342566E-15,42.8)) ;
#48055=CARTESIAN_POINT('',(27.3291439534833,-4.72149629179467E-15,42.7649855216442)) ;
#48056=CARTESIAN_POINT('Origin',(27.475,-4.6074255521944E-15,42.8)) ;
#48057=CARTESIAN_POINT('',(27.475,-4.70363407774438E-15,42.65)) ;
#48058=CARTESIAN_POINT('Origin',(27.475,-4.70363407774438E-15,42.8)) ;
#48059=CARTESIAN_POINT('',(27.3256289970792,0.0126778183972205,42.7947486756786)) ;
#48060=CARTESIAN_POINT('Origin',(27.475,-4.6074255521944E-15,42.8)) ;
#48061=CARTESIAN_POINT('Origin',(27.475,-4.6074255521944E-15,42.8)) ;
#48062=CARTESIAN_POINT('Origin',(27.41875,-0.56568542494924,43.0343145750508)) ;
#48063=CARTESIAN_POINT('',(27.2694861227066,-0.555190308577046,43.0238194586786)) ;
#48064=CARTESIAN_POINT('',(27.5680138772934,-0.576180541321434,43.044809691423)) ;
#48065=CARTESIAN_POINT('Origin',(27.41875,-0.56568542494924,43.0343145750508)) ;
#48066=CARTESIAN_POINT('',(27.2693789970792,-0.560434100627804,43.0216367566535)) ;
#48067=CARTESIAN_POINT('Origin',(27.41875,-0.56568542494924,43.0343145750508)) ;
#48068=CARTESIAN_POINT('Origin',(27.41875,-0.56568542494924,43.0343145750508)) ;
#48069=CARTESIAN_POINT('Origin',(27.3625,-0.8,43.6)) ;
#48070=CARTESIAN_POINT('',(27.2132361227066,-0.799999999999997,43.5851576640878)) ;
#48071=CARTESIAN_POINT('',(27.5117638772934,-0.799999999999999,43.6148423359122)) ;
#48072=CARTESIAN_POINT('Origin',(27.3625,-0.8,43.6)) ;
#48073=CARTESIAN_POINT('',(27.2131289970792,-0.805251324321435,43.5873221816028)) ;
#48074=CARTESIAN_POINT('Origin',(27.3625,-0.8,43.6)) ;
#48075=CARTESIAN_POINT('Origin',(27.3625,-0.8,43.6)) ;
#48076=CARTESIAN_POINT('Origin',(27.30625,-0.565685424949235,44.1656854249492)) ;
#48077=CARTESIAN_POINT('',(27.1569861227066,-0.576180541321439,44.1551903085771)) ;
#48078=CARTESIAN_POINT('',(27.4555138772934,-0.555190308577049,44.1761805413214)) ;
#48079=CARTESIAN_POINT('Origin',(27.30625,-0.565685424949235,44.1656854249493)) ;
#48080=CARTESIAN_POINT('',(27.1568789970792,-0.578363243346466,44.1604341006278)) ;
#48081=CARTESIAN_POINT('Origin',(27.30625,-0.565685424949235,44.1656854249492)) ;
#48082=CARTESIAN_POINT('Origin',(27.30625,-0.565685424949235,44.1656854249492)) ;
#48083=CARTESIAN_POINT('Origin',(27.25,1.76349139077219E-15,44.4)) ;
#48084=CARTESIAN_POINT('',(27.1007361227066,-0.0148423359122413,44.4)) ;
#48085=CARTESIAN_POINT('',(27.3992638772934,0.0148423359122413,44.4)) ;
#48086=CARTESIAN_POINT('Origin',(27.25,1.77635683940025E-15,44.4)) ;
#48087=CARTESIAN_POINT('',(27.1041439534833,1.7456291767219E-15,44.4350144783558)) ;
#48088=CARTESIAN_POINT('Origin',(27.25,1.77635683940025E-15,44.4)) ;
#48089=CARTESIAN_POINT('',(27.25,1.76349139077219E-15,44.55)) ;
#48090=CARTESIAN_POINT('Origin',(27.25,1.76349139077219E-15,44.4)) ;
#48091=CARTESIAN_POINT('',(27.1006289970792,-0.0126778183972294,44.4052513243214)) ;
#48092=CARTESIAN_POINT('Origin',(27.25,1.77635683940025E-15,44.4)) ;
#48093=CARTESIAN_POINT('Origin',(27.25,1.77635683940025E-15,44.4)) ;
#48094=CARTESIAN_POINT('Origin',(27.19375,0.565685424949238,44.1656854249492)) ;
#48095=CARTESIAN_POINT('',(27.0444861227066,0.555190308577043,44.1761805413214)) ;
#48096=CARTESIAN_POINT('',(27.3430138772934,0.576180541321431,44.155190308577)) ;
#48097=CARTESIAN_POINT('Origin',(27.19375,0.565685424949238,44.1656854249492)) ;
#48098=CARTESIAN_POINT('',(27.0443789970792,0.560434100627803,44.1783632433465)) ;
#48099=CARTESIAN_POINT('Origin',(27.19375,0.565685424949238,44.1656854249492)) ;
#48100=CARTESIAN_POINT('Origin',(27.19375,0.565685424949238,44.1656854249492)) ;
#48101=CARTESIAN_POINT('Origin',(27.1375,0.8,43.6)) ;
#48102=CARTESIAN_POINT('',(26.9882361227066,0.8,43.6148423359122)) ;
#48103=CARTESIAN_POINT('',(27.2867638772934,0.799999999999996,43.5851576640877)) ;
#48104=CARTESIAN_POINT('Origin',(27.1375,0.8,43.6)) ;
#48105=CARTESIAN_POINT('',(26.9881289970792,0.805251324321436,43.6126778183972)) ;
#48106=CARTESIAN_POINT('Origin',(27.1375,0.8,43.6)) ;
#48107=CARTESIAN_POINT('Origin',(27.1375,0.8,43.6)) ;
#48108=CARTESIAN_POINT('Origin',(27.08125,0.565685424949237,43.0343145750508)) ;
#48109=CARTESIAN_POINT('',(26.9319861227066,0.57618054132144,43.044809691423)) ;
#48110=CARTESIAN_POINT('',(27.2305138772934,0.555190308577053,43.0238194586786)) ;
#48111=CARTESIAN_POINT('Origin',(27.08125,0.565685424949237,43.0343145750508)) ;
#48112=CARTESIAN_POINT('',(26.9318789970792,0.578363243346467,43.0395658993722)) ;
#48113=CARTESIAN_POINT('Origin',(27.08125,0.565685424949237,43.0343145750508)) ;
#48114=CARTESIAN_POINT('Origin',(27.08125,0.565685424949237,43.0343145750508)) ;
#48115=CARTESIAN_POINT('Origin',(27.025,1.1766512962E-15,42.8)) ;
#48116=CARTESIAN_POINT('',(26.8757361227066,0.0148423359122424,42.8)) ;
#48117=CARTESIAN_POINT('',(27.1742638772934,-0.01484233591224,42.8)) ;
#48118=CARTESIAN_POINT('Origin',(27.025,1.16573417585641E-15,42.8)) ;
#48119=CARTESIAN_POINT('',(26.8791439534833,1.15878908214971E-15,42.7649855216442)) ;
#48120=CARTESIAN_POINT('Origin',(27.025,1.27675647831893E-15,42.8)) ;
#48121=CARTESIAN_POINT('',(27.025,1.1766512962E-15,42.65)) ;
#48122=CARTESIAN_POINT('Origin',(27.025,1.1766512962E-15,42.8)) ;
#48123=CARTESIAN_POINT('',(26.8756289970792,0.012677818397228,42.7947486756786)) ;
#48124=CARTESIAN_POINT('Origin',(27.025,1.27675647831893E-15,42.8)) ;
#48125=CARTESIAN_POINT('Origin',(27.025,1.27675647831893E-15,42.8)) ;
#48126=CARTESIAN_POINT('Origin',(26.96875,-0.56568542494924,43.0343145750508)) ;
#48127=CARTESIAN_POINT('',(26.8194861227066,-0.555190308577045,43.0238194586786)) ;
#48128=CARTESIAN_POINT('',(27.1180138772934,-0.576180541321435,43.044809691423)) ;
#48129=CARTESIAN_POINT('Origin',(26.96875,-0.56568542494924,43.0343145750508)) ;
#48130=CARTESIAN_POINT('',(26.8193789970792,-0.560434100627806,43.0216367566535)) ;
#48131=CARTESIAN_POINT('Origin',(26.96875,-0.56568542494924,43.0343145750508)) ;
#48132=CARTESIAN_POINT('Origin',(26.96875,-0.56568542494924,43.0343145750508)) ;
#48133=CARTESIAN_POINT('Origin',(26.9125,-0.8,43.6)) ;
#48134=CARTESIAN_POINT('',(26.7632361227066,-0.799999999999999,43.5851576640878)) ;
#48135=CARTESIAN_POINT('',(27.0617638772934,-0.799999999999999,43.6148423359123)) ;
#48136=CARTESIAN_POINT('Origin',(26.9125,-0.8,43.6)) ;
#48137=CARTESIAN_POINT('',(26.7631289970792,-0.805251324321435,43.5873221816028)) ;
#48138=CARTESIAN_POINT('Origin',(26.9125,-0.8,43.6)) ;
#48139=CARTESIAN_POINT('Origin',(26.9125,-0.8,43.6)) ;
#48140=CARTESIAN_POINT('Origin',(26.85625,-0.565685424949235,44.1656854249492)) ;
#48141=CARTESIAN_POINT('',(26.7069861227066,-0.57618054132143,44.1551903085771)) ;
#48142=CARTESIAN_POINT('',(27.0055138772934,-0.55519030857704,44.1761805413214)) ;
#48143=CARTESIAN_POINT('Origin',(26.85625,-0.565685424949235,44.1656854249492)) ;
#48144=CARTESIAN_POINT('',(26.7068789970792,-0.578363243346464,44.1604341006278)) ;
#48145=CARTESIAN_POINT('Origin',(26.85625,-0.565685424949235,44.1656854249492)) ;
#48146=CARTESIAN_POINT('Origin',(26.85625,-0.565685424949235,44.1656854249492)) ;
#48147=CARTESIAN_POINT('Origin',(26.8,1.56754790290861E-15,44.4)) ;
#48148=CARTESIAN_POINT('',(26.6507361227066,-0.0148423359122415,44.4)) ;
#48149=CARTESIAN_POINT('',(26.9492638772934,0.014842335912241,44.4)) ;
#48150=CARTESIAN_POINT('Origin',(26.8,1.55431223447522E-15,44.4)) ;
#48151=CARTESIAN_POINT('',(26.6541439534833,1.54968568885832E-15,44.4350144783558)) ;
#48152=CARTESIAN_POINT('Origin',(26.8,1.55431223447522E-15,44.4)) ;
#48153=CARTESIAN_POINT('',(26.8,1.56754790290861E-15,44.55)) ;
#48154=CARTESIAN_POINT('Origin',(26.8,1.56754790290861E-15,44.4)) ;
#48155=CARTESIAN_POINT('',(26.6506289970792,-0.0126778183972318,44.4052513243214)) ;
#48156=CARTESIAN_POINT('Origin',(26.8,1.55431223447522E-15,44.4)) ;
#48157=CARTESIAN_POINT('Origin',(26.8,1.55431223447522E-15,44.4)) ;
#48158=CARTESIAN_POINT('Origin',(26.74375,0.565685424949238,44.1656854249492)) ;
#48159=CARTESIAN_POINT('',(26.5944861227066,0.555190308577043,44.1761805413214)) ;
#48160=CARTESIAN_POINT('',(26.8930138772934,0.57618054132143,44.155190308577)) ;
#48161=CARTESIAN_POINT('Origin',(26.74375,0.565685424949238,44.1656854249492)) ;
#48162=CARTESIAN_POINT('',(26.5943789970792,0.560434100627802,44.1783632433465)) ;
#48163=CARTESIAN_POINT('Origin',(26.74375,0.565685424949238,44.1656854249492)) ;
#48164=CARTESIAN_POINT('Origin',(26.74375,0.565685424949238,44.1656854249492)) ;
#48165=CARTESIAN_POINT('Origin',(26.6875,0.8,43.6)) ;
#48166=CARTESIAN_POINT('',(26.5382361227066,0.800000000000001,43.6148423359122)) ;
#48167=CARTESIAN_POINT('',(26.8367638772934,0.800000000000002,43.5851576640877)) ;
#48168=CARTESIAN_POINT('Origin',(26.6875,0.8,43.6)) ;
#48169=CARTESIAN_POINT('',(26.5381289970792,0.805251324321436,43.6126778183972)) ;
#48170=CARTESIAN_POINT('Origin',(26.6875,0.8,43.6)) ;
#48171=CARTESIAN_POINT('Origin',(26.6875,0.8,43.6)) ;
#48172=CARTESIAN_POINT('Origin',(26.63125,0.565685424949237,43.0343145750508)) ;
#48173=CARTESIAN_POINT('',(26.4819861227066,0.57618054132144,43.0448096914229)) ;
#48174=CARTESIAN_POINT('',(26.7805138772934,0.555190308577052,43.0238194586786)) ;
#48175=CARTESIAN_POINT('Origin',(26.63125,0.565685424949237,43.0343145750508)) ;
#48176=CARTESIAN_POINT('',(26.4818789970792,0.578363243346473,43.0395658993722)) ;
#48177=CARTESIAN_POINT('Origin',(26.63125,0.565685424949238,43.0343145750508)) ;
#48178=CARTESIAN_POINT('Origin',(26.63125,0.565685424949238,43.0343145750508)) ;
#48179=CARTESIAN_POINT('Origin',(26.575,-4.31174710201723E-15,42.8)) ;
#48180=CARTESIAN_POINT('',(26.4257361227066,0.0148423359122368,42.8)) ;
#48181=CARTESIAN_POINT('',(26.7242638772934,-0.0148423359122456,42.8)) ;
#48182=CARTESIAN_POINT('Origin',(26.575,-4.38538094726937E-15,42.8)) ;
#48183=CARTESIAN_POINT('',(26.4291439534833,-4.32960931606752E-15,42.7649855216442)) ;
#48184=CARTESIAN_POINT('Origin',(26.575,-4.32986979603811E-15,42.8)) ;
#48185=CARTESIAN_POINT('',(26.575,-4.31174710201723E-15,42.65)) ;
#48186=CARTESIAN_POINT('Origin',(26.575,-4.31174710201723E-15,42.8)) ;
#48187=CARTESIAN_POINT('',(26.4256289970792,0.0126778183972232,42.7947486756786)) ;
#48188=CARTESIAN_POINT('Origin',(26.575,-4.32986979603811E-15,42.8)) ;
#48189=CARTESIAN_POINT('Origin',(26.575,-4.32986979603811E-15,42.8)) ;
#48190=CARTESIAN_POINT('Origin',(26.51875,-0.56568542494924,43.0343145750508)) ;
#48191=CARTESIAN_POINT('',(26.3694861227066,-0.555190308577044,43.0238194586786)) ;
#48192=CARTESIAN_POINT('',(26.6680138772934,-0.576180541321435,43.044809691423)) ;
#48193=CARTESIAN_POINT('Origin',(26.51875,-0.56568542494924,43.0343145750508)) ;
#48194=CARTESIAN_POINT('',(26.3693789970792,-0.560434100627805,43.0216367566535)) ;
#48195=CARTESIAN_POINT('Origin',(26.51875,-0.56568542494924,43.0343145750508)) ;
#48196=CARTESIAN_POINT('Origin',(26.51875,-0.56568542494924,43.0343145750508)) ;
#48197=CARTESIAN_POINT('Origin',(26.4625,-0.8,43.6)) ;
#48198=CARTESIAN_POINT('',(26.3132361227066,-0.8,43.5851576640878)) ;
#48199=CARTESIAN_POINT('',(26.6117638772934,-0.799999999999997,43.6148423359123)) ;
#48200=CARTESIAN_POINT('Origin',(26.4625,-0.8,43.6)) ;
#48201=CARTESIAN_POINT('',(26.3131289970792,-0.805251324321436,43.5873221816028)) ;
#48202=CARTESIAN_POINT('Origin',(26.4625,-0.8,43.6)) ;
#48203=CARTESIAN_POINT('Origin',(26.4625,-0.8,43.6)) ;
#48204=CARTESIAN_POINT('Origin',(26.40625,-0.565685424949235,44.1656854249492)) ;
#48205=CARTESIAN_POINT('',(26.2569861227066,-0.576180541321437,44.1551903085771)) ;
#48206=CARTESIAN_POINT('',(26.5555138772934,-0.55519030857705,44.1761805413215)) ;
#48207=CARTESIAN_POINT('Origin',(26.40625,-0.565685424949235,44.1656854249493)) ;
#48208=CARTESIAN_POINT('',(26.2568789970792,-0.578363243346465,44.1604341006278)) ;
#48209=CARTESIAN_POINT('Origin',(26.40625,-0.565685424949235,44.1656854249492)) ;
#48210=CARTESIAN_POINT('Origin',(26.40625,-0.565685424949235,44.1656854249492)) ;
#48211=CARTESIAN_POINT('Origin',(26.35,1.37160441504504E-15,44.4)) ;
#48212=CARTESIAN_POINT('',(26.2007361227066,-0.0148423359122412,44.4)) ;
#48213=CARTESIAN_POINT('',(26.4992638772934,0.0148423359122403,44.4)) ;
#48214=CARTESIAN_POINT('Origin',(26.35,1.33226762955019E-15,44.4)) ;
#48215=CARTESIAN_POINT('',(26.2041439534833,1.35374220099474E-15,44.4350144783558)) ;
#48216=CARTESIAN_POINT('Origin',(26.35,1.33226762955019E-15,44.4)) ;
#48217=CARTESIAN_POINT('',(26.35,1.37160441504504E-15,44.55)) ;
#48218=CARTESIAN_POINT('Origin',(26.35,1.37160441504504E-15,44.4)) ;
#48219=CARTESIAN_POINT('',(26.2006289970792,-0.012677818397228,44.4052513243214)) ;
#48220=CARTESIAN_POINT('Origin',(26.35,1.33226762955019E-15,44.4)) ;
#48221=CARTESIAN_POINT('Origin',(26.35,1.33226762955019E-15,44.4)) ;
#48222=CARTESIAN_POINT('Origin',(26.29375,0.565685424949237,44.1656854249492)) ;
#48223=CARTESIAN_POINT('',(26.1444861227066,0.555190308577042,44.1761805413214)) ;
#48224=CARTESIAN_POINT('',(26.4430138772934,0.576180541321429,44.155190308577)) ;
#48225=CARTESIAN_POINT('Origin',(26.29375,0.565685424949237,44.1656854249492)) ;
#48226=CARTESIAN_POINT('',(26.1443789970792,0.560434100627804,44.1783632433465)) ;
#48227=CARTESIAN_POINT('Origin',(26.29375,0.565685424949238,44.1656854249492)) ;
#48228=CARTESIAN_POINT('Origin',(26.29375,0.565685424949238,44.1656854249492)) ;
#48229=CARTESIAN_POINT('Origin',(26.2375,0.8,43.6)) ;
#48230=CARTESIAN_POINT('',(26.0882361227066,0.799999999999999,43.6148423359122)) ;
#48231=CARTESIAN_POINT('',(26.3867638772934,0.800000000000001,43.5851576640878)) ;
#48232=CARTESIAN_POINT('Origin',(26.2375,0.8,43.6)) ;
#48233=CARTESIAN_POINT('',(26.0881289970792,0.805251324321434,43.6126778183972)) ;
#48234=CARTESIAN_POINT('Origin',(26.2375,0.8,43.6)) ;
#48235=CARTESIAN_POINT('Origin',(26.2375,0.8,43.6)) ;
#48236=CARTESIAN_POINT('Origin',(26.18125,0.565685424949238,43.0343145750508)) ;
#48237=CARTESIAN_POINT('',(26.0319861227066,0.576180541321433,43.044809691423)) ;
#48238=CARTESIAN_POINT('',(26.3305138772934,0.555190308577043,43.0238194586786)) ;
#48239=CARTESIAN_POINT('Origin',(26.18125,0.565685424949238,43.0343145750508)) ;
#48240=CARTESIAN_POINT('',(26.0318789970792,0.578363243346464,43.0395658993722)) ;
#48241=CARTESIAN_POINT('Origin',(26.18125,0.565685424949238,43.0343145750508)) ;
#48242=CARTESIAN_POINT('Origin',(26.18125,0.565685424949238,43.0343145750508)) ;
#48243=CARTESIAN_POINT('Origin',(26.125,1.56853827192715E-15,42.8)) ;
#48244=CARTESIAN_POINT('',(25.9757361227066,0.0148423359122427,42.8)) ;
#48245=CARTESIAN_POINT('',(26.2742638772934,-0.0148423359122397,42.8)) ;
#48246=CARTESIAN_POINT('Origin',(26.125,1.55431223447522E-15,42.8)) ;
#48247=CARTESIAN_POINT('',(25.9791439534833,1.55067605787686E-15,42.7649855216442)) ;
#48248=CARTESIAN_POINT('Origin',(26.125,1.60982338570648E-15,42.8)) ;
#48249=CARTESIAN_POINT('',(26.125,1.56853827192715E-15,42.65)) ;
#48250=CARTESIAN_POINT('Origin',(26.125,1.56853827192715E-15,42.8)) ;
#48251=CARTESIAN_POINT('',(25.9756289970792,0.0126778183972272,42.7947486756786)) ;
#48252=CARTESIAN_POINT('Origin',(26.125,1.60982338570648E-15,42.8)) ;
#48253=CARTESIAN_POINT('Origin',(26.125,1.60982338570648E-15,42.8)) ;
#48254=CARTESIAN_POINT('Origin',(26.06875,-0.565685424949239,43.0343145750508)) ;
#48255=CARTESIAN_POINT('',(25.9194861227066,-0.555190308577046,43.0238194586786)) ;
#48256=CARTESIAN_POINT('',(26.2180138772934,-0.576180541321434,43.044809691423)) ;
#48257=CARTESIAN_POINT('Origin',(26.06875,-0.56568542494924,43.0343145750508)) ;
#48258=CARTESIAN_POINT('',(25.9193789970792,-0.560434100627805,43.0216367566535)) ;
#48259=CARTESIAN_POINT('Origin',(26.06875,-0.565685424949239,43.0343145750508)) ;
#48260=CARTESIAN_POINT('Origin',(26.06875,-0.565685424949239,43.0343145750508)) ;
#48261=CARTESIAN_POINT('Origin',(26.0125,-0.8,43.6)) ;
#48262=CARTESIAN_POINT('',(25.8632361227066,-0.799999999999999,43.5851576640878)) ;
#48263=CARTESIAN_POINT('',(26.1617638772934,-0.799999999999997,43.6148423359122)) ;
#48264=CARTESIAN_POINT('Origin',(26.0125,-0.8,43.6)) ;
#48265=CARTESIAN_POINT('',(25.8631289970792,-0.805251324321436,43.5873221816028)) ;
#48266=CARTESIAN_POINT('Origin',(26.0125,-0.8,43.6)) ;
#48267=CARTESIAN_POINT('Origin',(26.0125,-0.8,43.6)) ;
#48268=CARTESIAN_POINT('Origin',(25.95625,-0.565685424949236,44.1656854249492)) ;
#48269=CARTESIAN_POINT('',(25.8069861227066,-0.576180541321438,44.1551903085771)) ;
#48270=CARTESIAN_POINT('',(26.1055138772934,-0.555190308577051,44.1761805413215)) ;
#48271=CARTESIAN_POINT('Origin',(25.95625,-0.565685424949236,44.1656854249493)) ;
#48272=CARTESIAN_POINT('',(25.8068789970792,-0.578363243346467,44.1604341006278)) ;
#48273=CARTESIAN_POINT('Origin',(25.95625,-0.565685424949236,44.1656854249492)) ;
#48274=CARTESIAN_POINT('Origin',(25.95625,-0.565685424949236,44.1656854249492)) ;
#48275=CARTESIAN_POINT('Origin',(25.9,1.17566092718146E-15,44.4)) ;
#48276=CARTESIAN_POINT('',(25.7507361227066,-0.0148423359122419,44.4)) ;
#48277=CARTESIAN_POINT('',(26.0492638772934,0.0148423359122407,44.4)) ;
#48278=CARTESIAN_POINT('Origin',(25.9,1.22124532708767E-15,44.4)) ;
#48279=CARTESIAN_POINT('',(25.7541439534833,1.15779871313117E-15,44.4350144783558)) ;
#48280=CARTESIAN_POINT('Origin',(25.9,1.22124532708767E-15,44.4)) ;
#48281=CARTESIAN_POINT('',(25.9,1.17566092718146E-15,44.55)) ;
#48282=CARTESIAN_POINT('Origin',(25.9,1.17566092718146E-15,44.4)) ;
#48283=CARTESIAN_POINT('',(25.7506289970792,-0.0126778183972336,44.4052513243214)) ;
#48284=CARTESIAN_POINT('Origin',(25.9,1.22124532708767E-15,44.4)) ;
#48285=CARTESIAN_POINT('Origin',(25.9,1.22124532708767E-15,44.4)) ;
#48286=CARTESIAN_POINT('Origin',(25.84375,0.565685424949237,44.1656854249492)) ;
#48287=CARTESIAN_POINT('',(25.6944861227066,0.555190308577042,44.1761805413214)) ;
#48288=CARTESIAN_POINT('',(25.9930138772934,0.576180541321432,44.155190308577)) ;
#48289=CARTESIAN_POINT('Origin',(25.84375,0.565685424949237,44.1656854249492)) ;
#48290=CARTESIAN_POINT('',(25.6943789970792,0.560434100627803,44.1783632433465)) ;
#48291=CARTESIAN_POINT('Origin',(25.84375,0.565685424949237,44.1656854249492)) ;
#48292=CARTESIAN_POINT('Origin',(25.84375,0.565685424949237,44.1656854249492)) ;
#48293=CARTESIAN_POINT('Origin',(25.7875,0.8,43.6)) ;
#48294=CARTESIAN_POINT('',(25.6382361227066,0.8,43.6148423359122)) ;
#48295=CARTESIAN_POINT('',(25.9367638772934,0.8,43.5851576640878)) ;
#48296=CARTESIAN_POINT('Origin',(25.7875,0.8,43.6)) ;
#48297=CARTESIAN_POINT('',(25.6381289970792,0.805251324321434,43.6126778183972)) ;
#48298=CARTESIAN_POINT('Origin',(25.7875,0.8,43.6)) ;
#48299=CARTESIAN_POINT('Origin',(25.7875,0.8,43.6)) ;
#48300=CARTESIAN_POINT('Origin',(25.73125,0.565685424949238,43.0343145750508)) ;
#48301=CARTESIAN_POINT('',(25.5819861227066,0.576180541321433,43.044809691423)) ;
#48302=CARTESIAN_POINT('',(25.8805138772934,0.555190308577043,43.0238194586786)) ;
#48303=CARTESIAN_POINT('Origin',(25.73125,0.565685424949238,43.0343145750508)) ;
#48304=CARTESIAN_POINT('',(25.5818789970792,0.578363243346464,43.0395658993722)) ;
#48305=CARTESIAN_POINT('Origin',(25.73125,0.565685424949238,43.0343145750508)) ;
#48306=CARTESIAN_POINT('Origin',(25.73125,0.565685424949238,43.0343145750508)) ;
#48307=CARTESIAN_POINT('Origin',(25.675,-3.91986012629007E-15,42.8)) ;
#48308=CARTESIAN_POINT('',(25.5257361227066,0.0148423359122374,42.8)) ;
#48309=CARTESIAN_POINT('',(25.8242638772934,-0.014842335912245,42.8)) ;
#48310=CARTESIAN_POINT('Origin',(25.675,-3.88578058618805E-15,42.8)) ;
#48311=CARTESIAN_POINT('',(25.5291439534833,-3.93772234034036E-15,42.7649855216442)) ;
#48312=CARTESIAN_POINT('Origin',(25.675,-3.83026943495679E-15,42.8)) ;
#48313=CARTESIAN_POINT('',(25.675,-3.91986012629007E-15,42.65)) ;
#48314=CARTESIAN_POINT('Origin',(25.675,-3.91986012629007E-15,42.8)) ;
#48315=CARTESIAN_POINT('',(25.5256289970792,0.0126778183972214,42.7947486756786)) ;
#48316=CARTESIAN_POINT('Origin',(25.675,-3.83026943495679E-15,42.8)) ;
#48317=CARTESIAN_POINT('Origin',(25.675,-3.83026943495679E-15,42.8)) ;
#48318=CARTESIAN_POINT('Origin',(25.61875,-0.565685424949239,43.0343145750508)) ;
#48319=CARTESIAN_POINT('',(25.4694861227066,-0.555190308577046,43.0238194586786)) ;
#48320=CARTESIAN_POINT('',(25.7680138772934,-0.576180541321433,43.044809691423)) ;
#48321=CARTESIAN_POINT('Origin',(25.61875,-0.565685424949239,43.0343145750508)) ;
#48322=CARTESIAN_POINT('',(25.4693789970792,-0.560434100627804,43.0216367566535)) ;
#48323=CARTESIAN_POINT('Origin',(25.61875,-0.565685424949239,43.0343145750508)) ;
#48324=CARTESIAN_POINT('Origin',(25.61875,-0.565685424949239,43.0343145750508)) ;
#48325=CARTESIAN_POINT('Origin',(25.5625,-0.8,43.6)) ;
#48326=CARTESIAN_POINT('',(25.4132361227066,-0.799999999999997,43.5851576640878)) ;
#48327=CARTESIAN_POINT('',(25.7117638772934,-0.799999999999999,43.6148423359122)) ;
#48328=CARTESIAN_POINT('Origin',(25.5625,-0.8,43.6)) ;
#48329=CARTESIAN_POINT('',(25.4131289970792,-0.805251324321435,43.5873221816028)) ;
#48330=CARTESIAN_POINT('Origin',(25.5625,-0.8,43.6)) ;
#48331=CARTESIAN_POINT('Origin',(25.5625,-0.8,43.6)) ;
#48332=CARTESIAN_POINT('Origin',(25.50625,-0.565685424949236,44.1656854249492)) ;
#48333=CARTESIAN_POINT('',(25.3569861227066,-0.57618054132143,44.155190308577)) ;
#48334=CARTESIAN_POINT('',(25.6555138772934,-0.555190308577042,44.1761805413214)) ;
#48335=CARTESIAN_POINT('Origin',(25.50625,-0.565685424949236,44.1656854249492)) ;
#48336=CARTESIAN_POINT('',(25.3568789970792,-0.578363243346464,44.1604341006278)) ;
#48337=CARTESIAN_POINT('Origin',(25.50625,-0.565685424949236,44.1656854249492)) ;
#48338=CARTESIAN_POINT('Origin',(25.50625,-0.565685424949236,44.1656854249492)) ;
#48339=CARTESIAN_POINT('Origin',(25.45,9.79717439317883E-16,44.4)) ;
#48340=CARTESIAN_POINT('',(25.3007361227066,-0.014842335912242,44.4)) ;
#48341=CARTESIAN_POINT('',(25.5992638772934,0.0148423359122405,44.4)) ;
#48342=CARTESIAN_POINT('Origin',(25.45,9.99200722162641E-16,44.4)) ;
#48343=CARTESIAN_POINT('',(25.3041439534833,9.6185522526759E-16,44.4350144783558)) ;
#48344=CARTESIAN_POINT('Origin',(25.45,9.43689570931383E-16,44.4)) ;
#48345=CARTESIAN_POINT('',(25.45,9.79717439317883E-16,44.55)) ;
#48346=CARTESIAN_POINT('Origin',(25.45,9.79717439317883E-16,44.4)) ;
#48347=CARTESIAN_POINT('',(25.3006289970792,-0.0126778183972314,44.4052513243214)) ;
#48348=CARTESIAN_POINT('Origin',(25.45,9.43689570931383E-16,44.4)) ;
#48349=CARTESIAN_POINT('Origin',(25.45,9.43689570931383E-16,44.4)) ;
#48350=CARTESIAN_POINT('Origin',(25.39375,0.565685424949239,44.1656854249492)) ;
#48351=CARTESIAN_POINT('',(25.2444861227066,0.555190308577043,44.1761805413214)) ;
#48352=CARTESIAN_POINT('',(25.5430138772934,0.576180541321433,44.155190308577)) ;
#48353=CARTESIAN_POINT('Origin',(25.39375,0.565685424949239,44.1656854249492)) ;
#48354=CARTESIAN_POINT('',(25.2443789970792,0.560434100627806,44.1783632433465)) ;
#48355=CARTESIAN_POINT('Origin',(25.39375,0.565685424949239,44.1656854249492)) ;
#48356=CARTESIAN_POINT('Origin',(25.39375,0.565685424949239,44.1656854249492)) ;
#48357=CARTESIAN_POINT('Origin',(25.3375,0.8,43.6)) ;
#48358=CARTESIAN_POINT('',(25.1882361227066,0.800000000000002,43.6148423359122)) ;
#48359=CARTESIAN_POINT('',(25.4867638772934,0.799999999999999,43.5851576640878)) ;
#48360=CARTESIAN_POINT('Origin',(25.3375,0.8,43.6)) ;
#48361=CARTESIAN_POINT('',(25.1881289970792,0.805251324321435,43.6126778183972)) ;
#48362=CARTESIAN_POINT('Origin',(25.3375,0.8,43.6)) ;
#48363=CARTESIAN_POINT('Origin',(25.3375,0.8,43.6)) ;
#48364=CARTESIAN_POINT('Origin',(25.28125,0.565685424949238,43.0343145750508)) ;
#48365=CARTESIAN_POINT('',(25.1319861227066,0.576180541321432,43.044809691423)) ;
#48366=CARTESIAN_POINT('',(25.4305138772934,0.555190308577045,43.0238194586786)) ;
#48367=CARTESIAN_POINT('Origin',(25.28125,0.565685424949238,43.0343145750508)) ;
#48368=CARTESIAN_POINT('',(25.1318789970792,0.578363243346464,43.0395658993722)) ;
#48369=CARTESIAN_POINT('Origin',(25.28125,0.565685424949238,43.0343145750508)) ;
#48370=CARTESIAN_POINT('Origin',(25.28125,0.565685424949238,43.0343145750508)) ;
#48371=CARTESIAN_POINT('Origin',(25.225,-8.81745695386094E-16,42.8)) ;
#48372=CARTESIAN_POINT('',(25.0757361227066,0.0148423359122398,42.8)) ;
#48373=CARTESIAN_POINT('',(25.3742638772934,-0.0148423359122416,42.8)) ;
#48374=CARTESIAN_POINT('Origin',(25.225,-8.88178419700125E-16,42.8)) ;
#48375=CARTESIAN_POINT('',(25.0791439534833,-8.99607909436387E-16,42.7649855216442)) ;
#48376=CARTESIAN_POINT('Origin',(25.225,-8.88178419700125E-16,42.8)) ;
#48377=CARTESIAN_POINT('',(25.225,-8.81745695386094E-16,42.65)) ;
#48378=CARTESIAN_POINT('Origin',(25.225,-8.81745695386094E-16,42.8)) ;
#48379=CARTESIAN_POINT('',(25.0756289970792,0.012677818397226,42.7947486756786)) ;
#48380=CARTESIAN_POINT('Origin',(25.225,-8.88178419700125E-16,42.8)) ;
#48381=CARTESIAN_POINT('Origin',(25.225,-8.88178419700125E-16,42.8)) ;
#48382=CARTESIAN_POINT('Origin',(25.16875,-0.565685424949239,43.0343145750508)) ;
#48383=CARTESIAN_POINT('',(25.0194861227066,-0.555190308577046,43.0238194586786)) ;
#48384=CARTESIAN_POINT('',(25.3180138772934,-0.576180541321433,43.044809691423)) ;
#48385=CARTESIAN_POINT('Origin',(25.16875,-0.565685424949239,43.0343145750508)) ;
#48386=CARTESIAN_POINT('',(25.0193789970792,-0.560434100627804,43.0216367566535)) ;
#48387=CARTESIAN_POINT('Origin',(25.16875,-0.565685424949239,43.0343145750508)) ;
#48388=CARTESIAN_POINT('Origin',(25.16875,-0.565685424949239,43.0343145750508)) ;
#48389=CARTESIAN_POINT('Origin',(25.1125,-0.8,43.6)) ;
#48390=CARTESIAN_POINT('',(24.9632361227066,-0.799999999999999,43.5851576640878)) ;
#48391=CARTESIAN_POINT('',(25.2617638772934,-0.800000000000001,43.6148423359122)) ;
#48392=CARTESIAN_POINT('Origin',(25.1125,-0.8,43.6)) ;
#48393=CARTESIAN_POINT('',(24.9631289970792,-0.805251324321434,43.5873221816028)) ;
#48394=CARTESIAN_POINT('Origin',(25.1125,-0.8,43.6)) ;
#48395=CARTESIAN_POINT('Origin',(25.1125,-0.8,43.6)) ;
#48396=CARTESIAN_POINT('Origin',(25.05625,-0.565685424949238,44.1656854249492)) ;
#48397=CARTESIAN_POINT('',(24.9069861227066,-0.576180541321437,44.155190308577)) ;
#48398=CARTESIAN_POINT('',(25.2055138772934,-0.555190308577047,44.1761805413214)) ;
#48399=CARTESIAN_POINT('Origin',(25.05625,-0.565685424949238,44.1656854249492)) ;
#48400=CARTESIAN_POINT('',(24.9068789970792,-0.578363243346473,44.1604341006278)) ;
#48401=CARTESIAN_POINT('Origin',(25.05625,-0.565685424949238,44.1656854249492)) ;
#48402=CARTESIAN_POINT('Origin',(25.05625,-0.565685424949238,44.1656854249492)) ;
#48403=CARTESIAN_POINT('Origin',(25.,7.83773951454306E-16,44.4)) ;
#48404=CARTESIAN_POINT('',(24.8507361227066,-0.0148423359122422,44.4)) ;
#48405=CARTESIAN_POINT('',(25.1492638772934,0.0148423359122402,44.4)) ;
#48406=CARTESIAN_POINT('Origin',(25.,8.32667268468867E-16,44.4)) ;
#48407=CARTESIAN_POINT('',(24.8541439534833,7.65911737404014E-16,44.4350144783558)) ;
#48408=CARTESIAN_POINT('Origin',(25.,7.7715611723761E-16,44.4)) ;
#48409=CARTESIAN_POINT('',(25.,7.83773951454306E-16,44.55)) ;
#48410=CARTESIAN_POINT('Origin',(25.,7.83773951454306E-16,44.4)) ;
#48411=CARTESIAN_POINT('',(24.8506289970792,-0.0126778183972275,44.4052513243214)) ;
#48412=CARTESIAN_POINT('Origin',(25.,7.7715611723761E-16,44.4)) ;
#48413=CARTESIAN_POINT('Origin',(25.,7.7715611723761E-16,44.4)) ;
#48414=CARTESIAN_POINT('Origin',(24.94375,0.565685424949239,44.1656854249492)) ;
#48415=CARTESIAN_POINT('',(24.7944861227066,0.555190308577044,44.1761805413214)) ;
#48416=CARTESIAN_POINT('',(25.0930138772934,0.576180541321431,44.155190308577)) ;
#48417=CARTESIAN_POINT('Origin',(24.94375,0.565685424949239,44.1656854249492)) ;
#48418=CARTESIAN_POINT('',(24.7943789970792,0.560434100627806,44.1783632433465)) ;
#48419=CARTESIAN_POINT('Origin',(24.94375,0.565685424949239,44.1656854249492)) ;
#48420=CARTESIAN_POINT('Origin',(24.94375,0.565685424949239,44.1656854249492)) ;
#48421=CARTESIAN_POINT('Origin',(24.8875,0.8,43.6)) ;
#48422=CARTESIAN_POINT('',(24.7382361227066,0.800000000000001,43.6148423359122)) ;
#48423=CARTESIAN_POINT('',(25.0367638772934,0.799999999999999,43.5851576640878)) ;
#48424=CARTESIAN_POINT('Origin',(24.8875,0.8,43.6)) ;
#48425=CARTESIAN_POINT('',(24.7381289970792,0.805251324321435,43.6126778183972)) ;
#48426=CARTESIAN_POINT('Origin',(24.8875,0.8,43.6)) ;
#48427=CARTESIAN_POINT('Origin',(24.8875,0.8,43.6)) ;
#48428=CARTESIAN_POINT('Origin',(24.83125,0.565685424949238,43.0343145750508)) ;
#48429=CARTESIAN_POINT('',(24.6819861227066,0.576180541321432,43.044809691423)) ;
#48430=CARTESIAN_POINT('',(24.9805138772934,0.555190308577045,43.0238194586786)) ;
#48431=CARTESIAN_POINT('Origin',(24.83125,0.565685424949238,43.0343145750508)) ;
#48432=CARTESIAN_POINT('',(24.6818789970792,0.578363243346464,43.0395658993722)) ;
#48433=CARTESIAN_POINT('Origin',(24.83125,0.565685424949238,43.0343145750508)) ;
#48434=CARTESIAN_POINT('Origin',(24.83125,0.565685424949238,43.0343145750508)) ;
#48435=CARTESIAN_POINT('Origin',(24.775,-6.85802207522518E-16,42.8)) ;
#48436=CARTESIAN_POINT('',(24.6257361227066,0.0148423359122406,42.8)) ;
#48437=CARTESIAN_POINT('',(24.9242638772934,-0.0148423359122418,42.8)) ;
#48438=CARTESIAN_POINT('Origin',(24.775,-6.66133814775094E-16,42.8)) ;
#48439=CARTESIAN_POINT('',(24.6291439534833,-7.0366442157281E-16,42.7649855216442)) ;
#48440=CARTESIAN_POINT('Origin',(24.775,-6.10622663543836E-16,42.8)) ;
#48441=CARTESIAN_POINT('',(24.775,-6.85802207522518E-16,42.65)) ;
#48442=CARTESIAN_POINT('Origin',(24.775,-6.85802207522518E-16,42.8)) ;
#48443=CARTESIAN_POINT('',(24.6256289970792,0.0126778183972263,42.7947486756786)) ;
#48444=CARTESIAN_POINT('Origin',(24.775,-6.10622663543836E-16,42.8)) ;
#48445=CARTESIAN_POINT('Origin',(24.775,-6.10622663543836E-16,42.8)) ;
#48446=CARTESIAN_POINT('Origin',(24.71875,-0.565685424949239,43.0343145750508)) ;
#48447=CARTESIAN_POINT('',(24.5694861227066,-0.555190308577044,43.0238194586786)) ;
#48448=CARTESIAN_POINT('',(24.8680138772934,-0.576180541321434,43.044809691423)) ;
#48449=CARTESIAN_POINT('Origin',(24.71875,-0.565685424949239,43.0343145750508)) ;
#48450=CARTESIAN_POINT('',(24.5693789970792,-0.560434100627804,43.0216367566535)) ;
#48451=CARTESIAN_POINT('Origin',(24.71875,-0.565685424949239,43.0343145750508)) ;
#48452=CARTESIAN_POINT('Origin',(24.71875,-0.565685424949239,43.0343145750508)) ;
#48453=CARTESIAN_POINT('Origin',(24.6625,-0.8,43.6)) ;
#48454=CARTESIAN_POINT('',(24.5132361227066,-0.8,43.5851576640878)) ;
#48455=CARTESIAN_POINT('',(24.8117638772934,-0.8,43.6148423359122)) ;
#48456=CARTESIAN_POINT('Origin',(24.6625,-0.8,43.6)) ;
#48457=CARTESIAN_POINT('',(24.5131289970792,-0.805251324321434,43.5873221816028)) ;
#48458=CARTESIAN_POINT('Origin',(24.6625,-0.8,43.6)) ;
#48459=CARTESIAN_POINT('Origin',(24.6625,-0.8,43.6)) ;
#48460=CARTESIAN_POINT('Origin',(24.60625,-0.565685424949238,44.1656854249492)) ;
#48461=CARTESIAN_POINT('',(24.4569861227066,-0.576180541321437,44.155190308577)) ;
#48462=CARTESIAN_POINT('',(24.7555138772934,-0.555190308577047,44.1761805413214)) ;
#48463=CARTESIAN_POINT('Origin',(24.60625,-0.565685424949238,44.1656854249492)) ;
#48464=CARTESIAN_POINT('',(24.4568789970792,-0.578363243346473,44.1604341006278)) ;
#48465=CARTESIAN_POINT('Origin',(24.60625,-0.565685424949238,44.1656854249492)) ;
#48466=CARTESIAN_POINT('Origin',(24.60625,-0.565685424949238,44.1656854249492)) ;
#48467=CARTESIAN_POINT('Origin',(24.55,5.8783046359073E-16,44.4)) ;
#48468=CARTESIAN_POINT('',(24.4007361227066,-0.014842335912239,44.4)) ;
#48469=CARTESIAN_POINT('',(24.6992638772934,0.0148423359122435,44.4)) ;
#48470=CARTESIAN_POINT('Origin',(24.55,5.55111512312578E-16,44.4)) ;
#48471=CARTESIAN_POINT('',(24.4041439534833,5.69968249540437E-16,44.4350144783558)) ;
#48472=CARTESIAN_POINT('Origin',(24.55,4.9960036108132E-16,44.4)) ;
#48473=CARTESIAN_POINT('',(24.55,5.8783046359073E-16,44.55)) ;
#48474=CARTESIAN_POINT('Origin',(24.55,5.8783046359073E-16,44.4)) ;
#48475=CARTESIAN_POINT('',(24.4006289970792,-0.0126778183972271,44.4052513243214)) ;
#48476=CARTESIAN_POINT('Origin',(24.55,4.9960036108132E-16,44.4)) ;
#48477=CARTESIAN_POINT('Origin',(24.55,4.9960036108132E-16,44.4)) ;
#48478=CARTESIAN_POINT('Origin',(24.49375,0.565685424949239,44.1656854249492)) ;
#48479=CARTESIAN_POINT('',(24.3444861227066,0.555190308577044,44.1761805413214)) ;
#48480=CARTESIAN_POINT('',(24.6430138772934,0.576180541321431,44.155190308577)) ;
#48481=CARTESIAN_POINT('Origin',(24.49375,0.565685424949239,44.1656854249492)) ;
#48482=CARTESIAN_POINT('',(24.3443789970792,0.560434100627805,44.1783632433465)) ;
#48483=CARTESIAN_POINT('Origin',(24.49375,0.565685424949239,44.1656854249492)) ;
#48484=CARTESIAN_POINT('Origin',(24.49375,0.565685424949239,44.1656854249492)) ;
#48485=CARTESIAN_POINT('Origin',(24.4375,0.8,43.6)) ;
#48486=CARTESIAN_POINT('',(24.2882361227066,0.799999999999999,43.6148423359123)) ;
#48487=CARTESIAN_POINT('',(24.5867638772934,0.800000000000001,43.5851576640878)) ;
#48488=CARTESIAN_POINT('Origin',(24.4375,0.8,43.6)) ;
#48489=CARTESIAN_POINT('',(24.2881289970792,0.805251324321434,43.6126778183972)) ;
#48490=CARTESIAN_POINT('Origin',(24.4375,0.8,43.6)) ;
#48491=CARTESIAN_POINT('Origin',(24.4375,0.8,43.6)) ;
#48492=CARTESIAN_POINT('Origin',(24.38125,0.565685424949238,43.0343145750508)) ;
#48493=CARTESIAN_POINT('',(24.2319861227066,0.576180541321432,43.044809691423)) ;
#48494=CARTESIAN_POINT('',(24.5305138772934,0.555190308577044,43.0238194586786)) ;
#48495=CARTESIAN_POINT('Origin',(24.38125,0.565685424949238,43.0343145750508)) ;
#48496=CARTESIAN_POINT('',(24.2318789970792,0.578363243346464,43.0395658993722)) ;
#48497=CARTESIAN_POINT('Origin',(24.38125,0.565685424949238,43.0343145750508)) ;
#48498=CARTESIAN_POINT('Origin',(24.38125,0.565685424949238,43.0343145750508)) ;
#48499=CARTESIAN_POINT('Origin',(24.325,-4.89858719658941E-16,42.8)) ;
#48500=CARTESIAN_POINT('',(24.1757361227066,0.0148423359122407,42.8)) ;
#48501=CARTESIAN_POINT('',(24.4742638772934,-0.0148423359122417,42.8)) ;
#48502=CARTESIAN_POINT('Origin',(24.325,-4.44089209850063E-16,42.8)) ;
#48503=CARTESIAN_POINT('',(24.1791439534833,-5.07720933709234E-16,42.7649855216442)) ;
#48504=CARTESIAN_POINT('Origin',(24.325,-4.44089209850063E-16,42.8)) ;
#48505=CARTESIAN_POINT('',(24.325,-4.89858719658941E-16,42.65)) ;
#48506=CARTESIAN_POINT('Origin',(24.325,-4.89858719658941E-16,42.8)) ;
#48507=CARTESIAN_POINT('',(24.1756289970792,0.0126778183972273,42.7947486756786)) ;
#48508=CARTESIAN_POINT('Origin',(24.325,-4.44089209850063E-16,42.8)) ;
#48509=CARTESIAN_POINT('Origin',(24.325,-4.44089209850063E-16,42.8)) ;
#48510=CARTESIAN_POINT('Origin',(24.26875,-0.565685424949239,43.0343145750508)) ;
#48511=CARTESIAN_POINT('',(24.1194861227066,-0.555190308577044,43.0238194586786)) ;
#48512=CARTESIAN_POINT('',(24.4180138772934,-0.576180541321434,43.044809691423)) ;
#48513=CARTESIAN_POINT('Origin',(24.26875,-0.565685424949239,43.0343145750508)) ;
#48514=CARTESIAN_POINT('',(24.1193789970792,-0.560434100627804,43.0216367566535)) ;
#48515=CARTESIAN_POINT('Origin',(24.26875,-0.565685424949239,43.0343145750508)) ;
#48516=CARTESIAN_POINT('Origin',(24.26875,-0.565685424949239,43.0343145750508)) ;
#48517=CARTESIAN_POINT('Origin',(24.2125,-0.8,43.6)) ;
#48518=CARTESIAN_POINT('',(24.0632361227066,-0.800000000000001,43.5851576640878)) ;
#48519=CARTESIAN_POINT('',(24.3617638772934,-0.799999999999999,43.6148423359122)) ;
#48520=CARTESIAN_POINT('Origin',(24.2125,-0.8,43.6)) ;
#48521=CARTESIAN_POINT('',(24.0631289970792,-0.805251324321435,43.5873221816028)) ;
#48522=CARTESIAN_POINT('Origin',(24.2125,-0.8,43.6)) ;
#48523=CARTESIAN_POINT('Origin',(24.2125,-0.8,43.6)) ;
#48524=CARTESIAN_POINT('Origin',(24.15625,-0.565685424949238,44.1656854249492)) ;
#48525=CARTESIAN_POINT('',(24.0069861227066,-0.576180541321436,44.155190308577)) ;
#48526=CARTESIAN_POINT('',(24.3055138772934,-0.555190308577049,44.1761805413214)) ;
#48527=CARTESIAN_POINT('Origin',(24.15625,-0.565685424949238,44.1656854249492)) ;
#48528=CARTESIAN_POINT('',(24.0068789970792,-0.578363243346471,44.1604341006278)) ;
#48529=CARTESIAN_POINT('Origin',(24.15625,-0.565685424949238,44.1656854249492)) ;
#48530=CARTESIAN_POINT('Origin',(24.15625,-0.565685424949238,44.1656854249492)) ;
#48531=CARTESIAN_POINT('Origin',(24.1,3.91886975727153E-16,44.4)) ;
#48532=CARTESIAN_POINT('',(23.9507361227066,-0.014842335912242,44.4)) ;
#48533=CARTESIAN_POINT('',(24.2492638772934,0.0148423359122394,44.4)) ;
#48534=CARTESIAN_POINT('Origin',(24.1,4.9960036108132E-16,44.4)) ;
#48535=CARTESIAN_POINT('',(23.9541439534833,3.74024761676861E-16,44.4350144783558)) ;
#48536=CARTESIAN_POINT('Origin',(24.1,3.88578058618805E-16,44.4)) ;
#48537=CARTESIAN_POINT('',(24.1,3.91886975727153E-16,44.55)) ;
#48538=CARTESIAN_POINT('Origin',(24.1,3.91886975727153E-16,44.4)) ;
#48539=CARTESIAN_POINT('',(23.9506289970792,-0.0126778183972283,44.4052513243214)) ;
#48540=CARTESIAN_POINT('Origin',(24.1,3.88578058618805E-16,44.4)) ;
#48541=CARTESIAN_POINT('Origin',(24.1,3.88578058618805E-16,44.4)) ;
#48542=CARTESIAN_POINT('Origin',(24.04375,0.565685424949239,44.1656854249492)) ;
#48543=CARTESIAN_POINT('',(23.8944861227066,0.555190308577044,44.1761805413214)) ;
#48544=CARTESIAN_POINT('',(24.1930138772934,0.576180541321431,44.155190308577)) ;
#48545=CARTESIAN_POINT('Origin',(24.04375,0.565685424949239,44.1656854249492)) ;
#48546=CARTESIAN_POINT('',(23.8943789970792,0.560434100627805,44.1783632433465)) ;
#48547=CARTESIAN_POINT('Origin',(24.04375,0.565685424949239,44.1656854249492)) ;
#48548=CARTESIAN_POINT('Origin',(24.04375,0.565685424949239,44.1656854249492)) ;
#48549=CARTESIAN_POINT('Origin',(23.9875,0.8,43.6)) ;
#48550=CARTESIAN_POINT('',(23.8382361227066,0.8,43.6148423359122)) ;
#48551=CARTESIAN_POINT('',(24.1367638772934,0.800000000000001,43.5851576640878)) ;
#48552=CARTESIAN_POINT('Origin',(23.9875,0.8,43.6)) ;
#48553=CARTESIAN_POINT('',(23.8381289970792,0.805251324321434,43.6126778183972)) ;
#48554=CARTESIAN_POINT('Origin',(23.9875,0.8,43.6)) ;
#48555=CARTESIAN_POINT('Origin',(23.9875,0.8,43.6)) ;
#48556=CARTESIAN_POINT('Origin',(23.93125,0.565685424949238,43.0343145750508)) ;
#48557=CARTESIAN_POINT('',(23.7819861227066,0.576180541321434,43.044809691423)) ;
#48558=CARTESIAN_POINT('',(24.0805138772934,0.555190308577043,43.0238194586786)) ;
#48559=CARTESIAN_POINT('Origin',(23.93125,0.565685424949238,43.0343145750508)) ;
#48560=CARTESIAN_POINT('',(23.7818789970792,0.578363243346466,43.0395658993722)) ;
#48561=CARTESIAN_POINT('Origin',(23.93125,0.565685424949238,43.0343145750508)) ;
#48562=CARTESIAN_POINT('Origin',(23.93125,0.565685424949238,43.0343145750508)) ;
#48563=CARTESIAN_POINT('Origin',(23.875,-2.93915231795365E-16,42.8)) ;
#48564=CARTESIAN_POINT('',(23.7257361227066,0.0148423359122408,42.8)) ;
#48565=CARTESIAN_POINT('',(24.0242638772934,-0.0148423359122416,42.8)) ;
#48566=CARTESIAN_POINT('Origin',(23.875,-3.33066907387547E-16,42.8)) ;
#48567=CARTESIAN_POINT('',(23.7291439534833,-3.11777445845657E-16,42.7649855216442)) ;
#48568=CARTESIAN_POINT('Origin',(23.875,-2.77555756156289E-16,42.8)) ;
#48569=CARTESIAN_POINT('',(23.875,-2.93915231795365E-16,42.65)) ;
#48570=CARTESIAN_POINT('Origin',(23.875,-2.93915231795365E-16,42.8)) ;
#48571=CARTESIAN_POINT('',(23.7256289970792,0.0126778183972251,42.7947486756786)) ;
#48572=CARTESIAN_POINT('Origin',(23.875,-2.77555756156289E-16,42.8)) ;
#48573=CARTESIAN_POINT('Origin',(23.875,-2.77555756156289E-16,42.8)) ;
#48574=CARTESIAN_POINT('Origin',(23.81875,-0.565685424949239,43.0343145750508)) ;
#48575=CARTESIAN_POINT('',(23.6694861227066,-0.555190308577045,43.0238194586786)) ;
#48576=CARTESIAN_POINT('',(23.9680138772934,-0.576180541321433,43.044809691423)) ;
#48577=CARTESIAN_POINT('Origin',(23.81875,-0.565685424949239,43.0343145750508)) ;
#48578=CARTESIAN_POINT('',(23.6693789970792,-0.560434100627804,43.0216367566535)) ;
#48579=CARTESIAN_POINT('Origin',(23.81875,-0.565685424949239,43.0343145750508)) ;
#48580=CARTESIAN_POINT('Origin',(23.81875,-0.565685424949239,43.0343145750508)) ;
#48581=CARTESIAN_POINT('Origin',(23.7625,-0.8,43.6)) ;
#48582=CARTESIAN_POINT('',(23.6132361227066,-0.800000000000001,43.5851576640878)) ;
#48583=CARTESIAN_POINT('',(23.9117638772934,-0.799999999999999,43.6148423359122)) ;
#48584=CARTESIAN_POINT('Origin',(23.7625,-0.8,43.6)) ;
#48585=CARTESIAN_POINT('',(23.6131289970792,-0.805251324321435,43.5873221816028)) ;
#48586=CARTESIAN_POINT('Origin',(23.7625,-0.8,43.6)) ;
#48587=CARTESIAN_POINT('Origin',(23.7625,-0.8,43.6)) ;
#48588=CARTESIAN_POINT('Origin',(23.70625,-0.565685424949238,44.1656854249492)) ;
#48589=CARTESIAN_POINT('',(23.5569861227066,-0.576180541321436,44.155190308577)) ;
#48590=CARTESIAN_POINT('',(23.8555138772934,-0.555190308577049,44.1761805413214)) ;
#48591=CARTESIAN_POINT('Origin',(23.70625,-0.565685424949238,44.1656854249492)) ;
#48592=CARTESIAN_POINT('',(23.5568789970792,-0.57836324334647,44.1604341006278)) ;
#48593=CARTESIAN_POINT('Origin',(23.70625,-0.565685424949238,44.1656854249492)) ;
#48594=CARTESIAN_POINT('Origin',(23.70625,-0.565685424949238,44.1656854249492)) ;
#48595=CARTESIAN_POINT('Origin',(23.65,1.95943487863577E-16,44.4)) ;
#48596=CARTESIAN_POINT('',(23.5007361227066,-0.0148423359122428,44.4)) ;
#48597=CARTESIAN_POINT('',(23.7992638772934,0.0148423359122396,44.4)) ;
#48598=CARTESIAN_POINT('Origin',(23.65,2.22044604925031E-16,44.4)) ;
#48599=CARTESIAN_POINT('',(23.5041439534833,1.78081273813284E-16,44.4350144783558)) ;
#48600=CARTESIAN_POINT('Origin',(23.65,2.22044604925031E-16,44.4)) ;
#48601=CARTESIAN_POINT('',(23.65,1.95943487863577E-16,44.55)) ;
#48602=CARTESIAN_POINT('Origin',(23.65,1.95943487863577E-16,44.4)) ;
#48603=CARTESIAN_POINT('',(23.5006289970792,-0.012677818397231,44.4052513243214)) ;
#48604=CARTESIAN_POINT('Origin',(23.65,2.22044604925031E-16,44.4)) ;
#48605=CARTESIAN_POINT('Origin',(23.65,2.22044604925031E-16,44.4)) ;
#48606=CARTESIAN_POINT('Origin',(23.59375,0.565685424949238,44.1656854249492)) ;
#48607=CARTESIAN_POINT('',(23.4444861227066,0.555190308577043,44.1761805413214)) ;
#48608=CARTESIAN_POINT('',(23.7430138772934,0.576180541321433,44.155190308577)) ;
#48609=CARTESIAN_POINT('Origin',(23.59375,0.565685424949238,44.1656854249492)) ;
#48610=CARTESIAN_POINT('',(23.4443789970792,0.560434100627803,44.1783632433465)) ;
#48611=CARTESIAN_POINT('Origin',(23.59375,0.565685424949238,44.1656854249492)) ;
#48612=CARTESIAN_POINT('Origin',(23.59375,0.565685424949238,44.1656854249492)) ;
#48613=CARTESIAN_POINT('Origin',(23.5375,0.8,43.6)) ;
#48614=CARTESIAN_POINT('',(23.3882361227066,0.8,43.6148423359122)) ;
#48615=CARTESIAN_POINT('',(23.6867638772934,0.8,43.5851576640878)) ;
#48616=CARTESIAN_POINT('Origin',(23.5375,0.8,43.6)) ;
#48617=CARTESIAN_POINT('',(23.3881289970792,0.805251324321434,43.6126778183972)) ;
#48618=CARTESIAN_POINT('Origin',(23.5375,0.8,43.6)) ;
#48619=CARTESIAN_POINT('Origin',(23.5375,0.8,43.6)) ;
#48620=CARTESIAN_POINT('Origin',(23.48125,0.565685424949238,43.0343145750508)) ;
#48621=CARTESIAN_POINT('',(23.3319861227066,0.576180541321433,43.044809691423)) ;
#48622=CARTESIAN_POINT('',(23.6305138772934,0.555190308577043,43.0238194586786)) ;
#48623=CARTESIAN_POINT('Origin',(23.48125,0.565685424949238,43.0343145750508)) ;
#48624=CARTESIAN_POINT('',(23.3318789970792,0.578363243346464,43.0395658993722)) ;
#48625=CARTESIAN_POINT('Origin',(23.48125,0.565685424949238,43.0343145750508)) ;
#48626=CARTESIAN_POINT('Origin',(23.48125,0.565685424949238,43.0343145750508)) ;
#48627=CARTESIAN_POINT('Origin',(23.425,-9.79717439317883E-17,42.8)) ;
#48628=CARTESIAN_POINT('',(23.2757361227066,0.0148423359122411,42.8)) ;
#48629=CARTESIAN_POINT('',(23.5742638772934,-0.0148423359122413,42.8)) ;
#48630=CARTESIAN_POINT('Origin',(23.425,-1.11022302462516E-16,42.8)) ;
#48631=CARTESIAN_POINT('',(23.2791439534833,-1.15833957982081E-16,42.7649855216442)) ;
#48632=CARTESIAN_POINT('Origin',(23.425,-5.55111512312578E-17,42.8)) ;
#48633=CARTESIAN_POINT('',(23.425,-9.79717439317883E-17,42.65)) ;
#48634=CARTESIAN_POINT('Origin',(23.425,-9.79717439317883E-17,42.8)) ;
#48635=CARTESIAN_POINT('',(23.2756289970792,0.0126778183972252,42.7947486756786)) ;
#48636=CARTESIAN_POINT('Origin',(23.425,-5.55111512312578E-17,42.8)) ;
#48637=CARTESIAN_POINT('Origin',(23.425,-5.55111512312578E-17,42.8)) ;
#48638=CARTESIAN_POINT('Origin',(23.36875,-0.565685424949238,43.0343145750508)) ;
#48639=CARTESIAN_POINT('',(23.2194861227066,-0.555190308577045,43.0238194586786)) ;
#48640=CARTESIAN_POINT('',(23.5180138772934,-0.576180541321432,43.044809691423)) ;
#48641=CARTESIAN_POINT('Origin',(23.36875,-0.565685424949238,43.0343145750508)) ;
#48642=CARTESIAN_POINT('',(23.2193789970792,-0.560434100627803,43.0216367566535)) ;
#48643=CARTESIAN_POINT('Origin',(23.36875,-0.565685424949238,43.0343145750508)) ;
#48644=CARTESIAN_POINT('Origin',(23.36875,-0.565685424949238,43.0343145750508)) ;
#48645=CARTESIAN_POINT('Origin',(23.3125,-0.8,43.6)) ;
#48646=CARTESIAN_POINT('',(23.1632361227066,-0.799999999999999,43.5851576640878)) ;
#48647=CARTESIAN_POINT('',(23.4617638772934,-0.800000000000001,43.6148423359122)) ;
#48648=CARTESIAN_POINT('Origin',(23.3125,-0.8,43.6)) ;
#48649=CARTESIAN_POINT('',(23.1631289970792,-0.805251324321434,43.5873221816028)) ;
#48650=CARTESIAN_POINT('Origin',(23.3125,-0.8,43.6)) ;
#48651=CARTESIAN_POINT('Origin',(23.3125,-0.8,43.6)) ;
#48652=CARTESIAN_POINT('Origin',(23.25625,-0.565685424949238,44.1656854249492)) ;
#48653=CARTESIAN_POINT('',(23.1069861227066,-0.576180541321436,44.155190308577)) ;
#48654=CARTESIAN_POINT('',(23.4055138772934,-0.555190308577049,44.1761805413214)) ;
#48655=CARTESIAN_POINT('Origin',(23.25625,-0.565685424949238,44.1656854249492)) ;
#48656=CARTESIAN_POINT('',(23.1068789970792,-0.578363243346471,44.1604341006278)) ;
#48657=CARTESIAN_POINT('Origin',(23.25625,-0.565685424949238,44.1656854249492)) ;
#48658=CARTESIAN_POINT('Origin',(23.25625,-0.565685424949238,44.1656854249492)) ;
#48659=CARTESIAN_POINT('Origin',(30.371875,0.282842712474621,44.2828427124746)) ;
#48660=CARTESIAN_POINT('Origin',(30.34375,0.565685424949243,44.1656854249492)) ;
#48661=CARTESIAN_POINT('Origin',(30.315625,0.682842712474619,43.8828427124746)) ;
#48662=CARTESIAN_POINT('Origin',(30.2875,0.8,43.6)) ;
#48663=CARTESIAN_POINT('Origin',(30.259375,0.682842712474616,43.3171572875254)) ;
#48664=CARTESIAN_POINT('',(30.0820931715058,0.571828912643789,43.0491462663632)) ;
#48665=CARTESIAN_POINT('',(30.1100039970792,0.68809403679605,43.3298351059226)) ;
#48666=CARTESIAN_POINT('Origin',(30.23125,0.565685424949236,43.0343145750508)) ;
#48667=CARTESIAN_POINT('Origin',(30.23125,0.565685424949236,43.0343145750508)) ;
#48668=CARTESIAN_POINT('Origin',(30.203125,0.282842712474613,42.9171572875254)) ;
#48669=CARTESIAN_POINT('',(30.0258431715057,0.0148316913124444,42.8061434876946)) ;
#48670=CARTESIAN_POINT('',(30.0537539970792,0.295520530871838,42.9224086118468)) ;
#48671=CARTESIAN_POINT('Origin',(30.175,-1.0325074129014E-14,42.8)) ;
#48672=CARTESIAN_POINT('Origin',(30.175,-1.0325074129014E-14,42.8)) ;
#48673=CARTESIAN_POINT('Origin',(30.146875,-0.282842712474623,42.9171572875254)) ;
#48674=CARTESIAN_POINT('',(29.9695931715058,-0.550853733636784,43.0281710873562)) ;
#48675=CARTESIAN_POINT('',(29.9975039970792,-0.270164894077399,42.9119059632039)) ;
#48676=CARTESIAN_POINT('Origin',(30.11875,-0.56568542494924,43.0343145750508)) ;
#48677=CARTESIAN_POINT('Origin',(30.11875,-0.56568542494924,43.0343145750508)) ;
#48678=CARTESIAN_POINT('Origin',(30.090625,-0.68284271247462,43.3171572875254)) ;
#48679=CARTESIAN_POINT('',(29.9133431715058,-0.793856512305449,43.5851683086875)) ;
#48680=CARTESIAN_POINT('',(29.9412539970792,-0.677591388153187,43.3044794691282)) ;
#48681=CARTESIAN_POINT('Origin',(30.0625,-0.8,43.6)) ;
#48682=CARTESIAN_POINT('Origin',(30.0625,-0.8,43.6)) ;
#48683=CARTESIAN_POINT('Origin',(30.034375,-0.682842712474619,43.8828427124746)) ;
#48684=CARTESIAN_POINT('',(29.8570931715057,-0.57182891264379,44.1508537336368)) ;
#48685=CARTESIAN_POINT('',(29.8850039970792,-0.688094036796053,43.8701648940774)) ;
#48686=CARTESIAN_POINT('Origin',(30.00625,-0.565685424949241,44.1656854249492)) ;
#48687=CARTESIAN_POINT('Origin',(30.00625,-0.565685424949241,44.1656854249492)) ;
#48688=CARTESIAN_POINT('Origin',(29.978125,-0.282842712474615,44.2828427124746)) ;
#48689=CARTESIAN_POINT('',(29.8008431715058,-0.0148316913124417,44.3938565123055)) ;
#48690=CARTESIAN_POINT('',(29.8287539970792,-0.295520530871839,44.2775913881532)) ;
#48691=CARTESIAN_POINT('Origin',(29.95,1.26565424807268E-14,44.4)) ;
#48692=CARTESIAN_POINT('Origin',(29.95,1.26565424807268E-14,44.4)) ;
#48693=CARTESIAN_POINT('Origin',(29.921875,0.282842712474626,44.2828427124746)) ;
#48694=CARTESIAN_POINT('',(29.7445931715057,0.55085373363679,44.1718289126438)) ;
#48695=CARTESIAN_POINT('',(29.7725039970792,0.270164894077401,44.2880940367961)) ;
#48696=CARTESIAN_POINT('Origin',(29.89375,0.565685424949242,44.1656854249492)) ;
#48697=CARTESIAN_POINT('Origin',(29.89375,0.565685424949242,44.1656854249492)) ;
#48698=CARTESIAN_POINT('Origin',(29.865625,0.682842712474621,43.8828427124746)) ;
#48699=CARTESIAN_POINT('',(29.6883431715058,0.793856512305448,43.6148316913125)) ;
#48700=CARTESIAN_POINT('',(29.7162539970792,0.677591388153188,43.8955205308718)) ;
#48701=CARTESIAN_POINT('Origin',(29.8375,0.8,43.6)) ;
#48702=CARTESIAN_POINT('Origin',(29.8375,0.8,43.6)) ;
#48703=CARTESIAN_POINT('Origin',(29.809375,0.682842712474618,43.3171572875254)) ;
#48704=CARTESIAN_POINT('',(29.6320931715058,0.57182891264379,43.0491462663632)) ;
#48705=CARTESIAN_POINT('',(29.6600039970792,0.688094036796052,43.3298351059226)) ;
#48706=CARTESIAN_POINT('Origin',(29.78125,0.565685424949238,43.0343145750508)) ;
#48707=CARTESIAN_POINT('Origin',(29.78125,0.565685424949238,43.0343145750508)) ;
#48708=CARTESIAN_POINT('Origin',(29.753125,0.282842712474618,42.9171572875254)) ;
#48709=CARTESIAN_POINT('',(29.5758431715058,0.0148316913124541,42.8061434876946)) ;
#48710=CARTESIAN_POINT('',(29.6037539970792,0.295520530871842,42.9224086118468)) ;
#48711=CARTESIAN_POINT('Origin',(29.725,5.55111512312578E-17,42.8)) ;
#48712=CARTESIAN_POINT('Origin',(29.725,5.55111512312578E-17,42.8)) ;
#48713=CARTESIAN_POINT('Origin',(29.696875,-0.282842712474618,42.9171572875254)) ;
#48714=CARTESIAN_POINT('',(29.5195931715058,-0.55085373363678,43.0281710873562)) ;
#48715=CARTESIAN_POINT('',(29.5475039970792,-0.270164894077394,42.9119059632039)) ;
#48716=CARTESIAN_POINT('Origin',(29.66875,-0.565685424949235,43.0343145750508)) ;
#48717=CARTESIAN_POINT('Origin',(29.66875,-0.565685424949235,43.0343145750508)) ;
#48718=CARTESIAN_POINT('Origin',(29.640625,-0.682842712474618,43.3171572875254)) ;
#48719=CARTESIAN_POINT('',(29.4633431715058,-0.793856512305448,43.5851683086876)) ;
#48720=CARTESIAN_POINT('',(29.4912539970792,-0.677591388153185,43.3044794691282)) ;
#48721=CARTESIAN_POINT('Origin',(29.6125,-0.799999999999998,43.6)) ;
#48722=CARTESIAN_POINT('Origin',(29.6125,-0.799999999999998,43.6)) ;
#48723=CARTESIAN_POINT('Origin',(29.584375,-0.682842712474617,43.8828427124746)) ;
#48724=CARTESIAN_POINT('',(29.4070931715057,-0.571828912643784,44.1508537336368)) ;
#48725=CARTESIAN_POINT('',(29.4350039970792,-0.688094036796051,43.8701648940774)) ;
#48726=CARTESIAN_POINT('Origin',(29.55625,-0.565685424949235,44.1656854249492)) ;
#48727=CARTESIAN_POINT('Origin',(29.55625,-0.565685424949235,44.1656854249492)) ;
#48728=CARTESIAN_POINT('Origin',(29.528125,-0.282842712474616,44.2828427124746)) ;
#48729=CARTESIAN_POINT('',(29.3508431715058,-0.0148316913124563,44.3938565123055)) ;
#48730=CARTESIAN_POINT('',(29.3787539970792,-0.295520530871841,44.2775913881532)) ;
#48731=CARTESIAN_POINT('Origin',(29.5,-1.49880108324396E-15,44.4)) ;
#48732=CARTESIAN_POINT('Origin',(29.5,-1.49880108324396E-15,44.4)) ;
#48733=CARTESIAN_POINT('Origin',(29.471875,0.282842712474621,44.2828427124746)) ;
#48734=CARTESIAN_POINT('',(29.2945931715057,0.550853733636796,44.1718289126438)) ;
#48735=CARTESIAN_POINT('',(29.3225039970792,0.270164894077397,44.2880940367961)) ;
#48736=CARTESIAN_POINT('Origin',(29.44375,0.565685424949242,44.1656854249492)) ;
#48737=CARTESIAN_POINT('Origin',(29.44375,0.565685424949242,44.1656854249492)) ;
#48738=CARTESIAN_POINT('Origin',(29.415625,0.682842712474619,43.8828427124746)) ;
#48739=CARTESIAN_POINT('',(29.2383431715058,0.79385651230545,43.6148316913125)) ;
#48740=CARTESIAN_POINT('',(29.2662539970792,0.677591388153186,43.8955205308718)) ;
#48741=CARTESIAN_POINT('Origin',(29.3875,0.8,43.6)) ;
#48742=CARTESIAN_POINT('Origin',(29.3875,0.8,43.6)) ;
#48743=CARTESIAN_POINT('Origin',(29.359375,0.682842712474616,43.3171572875254)) ;
#48744=CARTESIAN_POINT('',(29.1820931715058,0.571828912643789,43.0491462663632)) ;
#48745=CARTESIAN_POINT('',(29.2100039970792,0.68809403679605,43.3298351059226)) ;
#48746=CARTESIAN_POINT('Origin',(29.33125,0.565685424949237,43.0343145750508)) ;
#48747=CARTESIAN_POINT('Origin',(29.33125,0.565685424949237,43.0343145750508)) ;
#48748=CARTESIAN_POINT('Origin',(29.303125,0.282842712474614,42.9171572875254)) ;
#48749=CARTESIAN_POINT('',(29.1258431715058,0.0148316913124456,42.8061434876946)) ;
#48750=CARTESIAN_POINT('',(29.1537539970792,0.295520530871838,42.9224086118468)) ;
#48751=CARTESIAN_POINT('Origin',(29.275,-9.38138455808257E-15,42.8)) ;
#48752=CARTESIAN_POINT('Origin',(29.275,-9.38138455808257E-15,42.8)) ;
#48753=CARTESIAN_POINT('Origin',(29.246875,-0.282842712474623,42.9171572875254)) ;
#48754=CARTESIAN_POINT('',(29.0695931715058,-0.550853733636788,43.0281710873562)) ;
#48755=CARTESIAN_POINT('',(29.0975039970792,-0.270164894077398,42.9119059632039)) ;
#48756=CARTESIAN_POINT('Origin',(29.21875,-0.56568542494924,43.0343145750508)) ;
#48757=CARTESIAN_POINT('Origin',(29.21875,-0.56568542494924,43.0343145750508)) ;
#48758=CARTESIAN_POINT('Origin',(29.190625,-0.68284271247462,43.3171572875254)) ;
#48759=CARTESIAN_POINT('',(29.0133431715058,-0.79385651230545,43.5851683086875)) ;
#48760=CARTESIAN_POINT('',(29.0412539970792,-0.677591388153187,43.3044794691282)) ;
#48761=CARTESIAN_POINT('Origin',(29.1625,-0.8,43.6)) ;
#48762=CARTESIAN_POINT('Origin',(29.1625,-0.8,43.6)) ;
#48763=CARTESIAN_POINT('Origin',(29.134375,-0.682842712474619,43.8828427124746)) ;
#48764=CARTESIAN_POINT('',(28.9570931715058,-0.571828912643791,44.1508537336368)) ;
#48765=CARTESIAN_POINT('',(28.9850039970792,-0.688094036796053,43.8701648940774)) ;
#48766=CARTESIAN_POINT('Origin',(29.10625,-0.565685424949241,44.1656854249492)) ;
#48767=CARTESIAN_POINT('Origin',(29.10625,-0.565685424949241,44.1656854249492)) ;
#48768=CARTESIAN_POINT('Origin',(29.078125,-0.282842712474621,44.2828427124746)) ;
#48769=CARTESIAN_POINT('',(28.9008431715057,-0.014831691312453,44.3938565123055)) ;
#48770=CARTESIAN_POINT('',(28.9287539970792,-0.295520530871846,44.2775913881532)) ;
#48771=CARTESIAN_POINT('Origin',(29.05,1.11022302462516E-15,44.4)) ;
#48772=CARTESIAN_POINT('Origin',(29.05,1.11022302462516E-15,44.4)) ;
#48773=CARTESIAN_POINT('Origin',(29.021875,0.28284271247462,44.2828427124746)) ;
#48774=CARTESIAN_POINT('',(28.8445931715058,0.55085373363679,44.1718289126438)) ;
#48775=CARTESIAN_POINT('',(28.8725039970792,0.270164894077396,44.2880940367961)) ;
#48776=CARTESIAN_POINT('Origin',(28.99375,0.565685424949242,44.1656854249492)) ;
#48777=CARTESIAN_POINT('Origin',(28.99375,0.565685424949242,44.1656854249492)) ;
#48778=CARTESIAN_POINT('Origin',(28.965625,0.682842712474621,43.8828427124746)) ;
#48779=CARTESIAN_POINT('',(28.7883431715058,0.793856512305448,43.6148316913125)) ;
#48780=CARTESIAN_POINT('',(28.8162539970792,0.677591388153188,43.8955205308718)) ;
#48781=CARTESIAN_POINT('Origin',(28.9375,0.8,43.6)) ;
#48782=CARTESIAN_POINT('Origin',(28.9375,0.8,43.6)) ;
#48783=CARTESIAN_POINT('Origin',(28.909375,0.682842712474618,43.3171572875254)) ;
#48784=CARTESIAN_POINT('',(28.7320931715057,0.571828912643787,43.0491462663632)) ;
#48785=CARTESIAN_POINT('',(28.7600039970792,0.688094036796052,43.3298351059226)) ;
#48786=CARTESIAN_POINT('Origin',(28.88125,0.565685424949238,43.0343145750508)) ;
#48787=CARTESIAN_POINT('Origin',(28.88125,0.565685424949238,43.0343145750508)) ;
#48788=CARTESIAN_POINT('Origin',(28.853125,0.282842712474619,42.9171572875254)) ;
#48789=CARTESIAN_POINT('',(28.6758431715058,0.0148316913124594,42.8061434876946)) ;
#48790=CARTESIAN_POINT('',(28.7037539970792,0.295520530871843,42.9224086118468)) ;
#48791=CARTESIAN_POINT('Origin',(28.825,4.77395900588817E-15,42.8)) ;
#48792=CARTESIAN_POINT('Origin',(28.825,4.77395900588817E-15,42.8)) ;
#48793=CARTESIAN_POINT('Origin',(28.796875,-0.282842712474618,42.9171572875254)) ;
#48794=CARTESIAN_POINT('',(28.6195931715057,-0.55085373363679,43.0281710873562)) ;
#48795=CARTESIAN_POINT('',(28.6475039970792,-0.270164894077393,42.9119059632039)) ;
#48796=CARTESIAN_POINT('Origin',(28.76875,-0.56568542494924,43.0343145750508)) ;
#48797=CARTESIAN_POINT('Origin',(28.76875,-0.56568542494924,43.0343145750508)) ;
#48798=CARTESIAN_POINT('Origin',(28.740625,-0.682842712474618,43.3171572875254)) ;
#48799=CARTESIAN_POINT('',(28.5633431715058,-0.793856512305451,43.5851683086876)) ;
#48800=CARTESIAN_POINT('',(28.5912539970792,-0.677591388153185,43.3044794691282)) ;
#48801=CARTESIAN_POINT('Origin',(28.7125,-0.8,43.6)) ;
#48802=CARTESIAN_POINT('Origin',(28.7125,-0.8,43.6)) ;
#48803=CARTESIAN_POINT('Origin',(28.684375,-0.682842712474617,43.8828427124746)) ;
#48804=CARTESIAN_POINT('',(28.5070931715058,-0.571828912643787,44.1508537336368)) ;
#48805=CARTESIAN_POINT('',(28.5350039970792,-0.688094036796051,43.8701648940774)) ;
#48806=CARTESIAN_POINT('Origin',(28.65625,-0.565685424949235,44.1656854249492)) ;
#48807=CARTESIAN_POINT('Origin',(28.65625,-0.565685424949235,44.1656854249492)) ;
#48808=CARTESIAN_POINT('Origin',(28.628125,-0.282842712474616,44.2828427124746)) ;
#48809=CARTESIAN_POINT('',(28.4508431715058,-0.0148316913124563,44.3938565123055)) ;
#48810=CARTESIAN_POINT('',(28.4787539970792,-0.29552053087184,44.2775913881532)) ;
#48811=CARTESIAN_POINT('Origin',(28.6,-2.22044604925031E-15,44.4)) ;
#48812=CARTESIAN_POINT('Origin',(28.6,-2.22044604925031E-15,44.4)) ;
#48813=CARTESIAN_POINT('Origin',(28.571875,0.28284271247462,44.2828427124746)) ;
#48814=CARTESIAN_POINT('',(28.3945931715058,0.550853733636788,44.1718289126438)) ;
#48815=CARTESIAN_POINT('',(28.4225039970792,0.270164894077396,44.2880940367961)) ;
#48816=CARTESIAN_POINT('Origin',(28.54375,0.565685424949242,44.1656854249492)) ;
#48817=CARTESIAN_POINT('Origin',(28.54375,0.565685424949242,44.1656854249492)) ;
#48818=CARTESIAN_POINT('Origin',(28.515625,0.682842712474619,43.8828427124746)) ;
#48819=CARTESIAN_POINT('',(28.3383431715057,0.793856512305449,43.6148316913125)) ;
#48820=CARTESIAN_POINT('',(28.3662539970792,0.677591388153185,43.8955205308718)) ;
#48821=CARTESIAN_POINT('Origin',(28.4875,0.8,43.6)) ;
#48822=CARTESIAN_POINT('Origin',(28.4875,0.8,43.6)) ;
#48823=CARTESIAN_POINT('Origin',(28.459375,0.682842712474616,43.3171572875254)) ;
#48824=CARTESIAN_POINT('',(28.2820931715057,0.571828912643789,43.0491462663632)) ;
#48825=CARTESIAN_POINT('',(28.3100039970792,0.68809403679605,43.3298351059226)) ;
#48826=CARTESIAN_POINT('Origin',(28.43125,0.565685424949237,43.0343145750508)) ;
#48827=CARTESIAN_POINT('Origin',(28.43125,0.565685424949237,43.0343145750508)) ;
#48828=CARTESIAN_POINT('Origin',(28.403125,0.282842712474614,42.9171572875254)) ;
#48829=CARTESIAN_POINT('',(28.2258431715058,0.0148316913124452,42.8061434876946)) ;
#48830=CARTESIAN_POINT('',(28.2537539970792,0.295520530871839,42.9224086118468)) ;
#48831=CARTESIAN_POINT('Origin',(28.375,-9.54791801177635E-15,42.8)) ;
#48832=CARTESIAN_POINT('Origin',(28.375,-9.54791801177635E-15,42.8)) ;
#48833=CARTESIAN_POINT('Origin',(28.346875,-0.282842712474623,42.9171572875254)) ;
#48834=CARTESIAN_POINT('',(28.1695931715057,-0.550853733636789,43.0281710873562)) ;
#48835=CARTESIAN_POINT('',(28.1975039970792,-0.270164894077398,42.9119059632039)) ;
#48836=CARTESIAN_POINT('Origin',(28.31875,-0.56568542494924,43.0343145750508)) ;
#48837=CARTESIAN_POINT('Origin',(28.31875,-0.56568542494924,43.0343145750508)) ;
#48838=CARTESIAN_POINT('Origin',(28.290625,-0.68284271247462,43.3171572875254)) ;
#48839=CARTESIAN_POINT('',(28.1133431715058,-0.79385651230545,43.5851683086875)) ;
#48840=CARTESIAN_POINT('',(28.1412539970792,-0.677591388153187,43.3044794691282)) ;
#48841=CARTESIAN_POINT('Origin',(28.2625,-0.8,43.6)) ;
#48842=CARTESIAN_POINT('Origin',(28.2625,-0.8,43.6)) ;
#48843=CARTESIAN_POINT('Origin',(28.234375,-0.682842712474619,43.8828427124746)) ;
#48844=CARTESIAN_POINT('',(28.0570931715058,-0.571828912643794,44.1508537336368)) ;
#48845=CARTESIAN_POINT('',(28.0850039970792,-0.688094036796053,43.8701648940774)) ;
#48846=CARTESIAN_POINT('Origin',(28.20625,-0.565685424949242,44.1656854249492)) ;
#48847=CARTESIAN_POINT('Origin',(28.20625,-0.565685424949242,44.1656854249492)) ;
#48848=CARTESIAN_POINT('Origin',(28.178125,-0.282842712474616,44.2828427124746)) ;
#48849=CARTESIAN_POINT('',(28.0008431715058,-0.0148316913124424,44.3938565123055)) ;
#48850=CARTESIAN_POINT('',(28.0287539970792,-0.295520530871839,44.2775913881532)) ;
#48851=CARTESIAN_POINT('Origin',(28.15,1.19904086659517E-14,44.4)) ;
#48852=CARTESIAN_POINT('Origin',(28.15,1.19904086659517E-14,44.4)) ;
#48853=CARTESIAN_POINT('Origin',(28.121875,0.282842712474625,44.2828427124746)) ;
#48854=CARTESIAN_POINT('',(27.9445931715057,0.55085373363679,44.1718289126438)) ;
#48855=CARTESIAN_POINT('',(27.9725039970792,0.2701648940774,44.2880940367961)) ;
#48856=CARTESIAN_POINT('Origin',(28.09375,0.565685424949242,44.1656854249492)) ;
#48857=CARTESIAN_POINT('Origin',(28.09375,0.565685424949242,44.1656854249492)) ;
#48858=CARTESIAN_POINT('Origin',(28.065625,0.682842712474621,43.8828427124746)) ;
#48859=CARTESIAN_POINT('',(27.8883431715058,0.793856512305448,43.6148316913124)) ;
#48860=CARTESIAN_POINT('',(27.9162539970792,0.677591388153188,43.8955205308718)) ;
#48861=CARTESIAN_POINT('Origin',(28.0375,0.8,43.6)) ;
#48862=CARTESIAN_POINT('Origin',(28.0375,0.8,43.6)) ;
#48863=CARTESIAN_POINT('Origin',(28.009375,0.682842712474619,43.3171572875254)) ;
#48864=CARTESIAN_POINT('',(27.8320931715058,0.571828912643788,43.0491462663632)) ;
#48865=CARTESIAN_POINT('',(27.8600039970792,0.688094036796052,43.3298351059226)) ;
#48866=CARTESIAN_POINT('Origin',(27.98125,0.565685424949239,43.0343145750508)) ;
#48867=CARTESIAN_POINT('Origin',(27.98125,0.565685424949239,43.0343145750508)) ;
#48868=CARTESIAN_POINT('Origin',(27.953125,0.282842712474619,42.9171572875254)) ;
#48869=CARTESIAN_POINT('',(27.7758431715058,0.01483169131246,42.8061434876946)) ;
#48870=CARTESIAN_POINT('',(27.8037539970792,0.295520530871844,42.9224086118468)) ;
#48871=CARTESIAN_POINT('Origin',(27.925,5.21804821573824E-15,42.8)) ;
#48872=CARTESIAN_POINT('Origin',(27.925,5.21804821573824E-15,42.8)) ;
#48873=CARTESIAN_POINT('Origin',(27.896875,-0.282842712474618,42.9171572875254)) ;
#48874=CARTESIAN_POINT('',(27.7195931715058,-0.550853733636787,43.0281710873562)) ;
#48875=CARTESIAN_POINT('',(27.7475039970792,-0.270164894077393,42.9119059632039)) ;
#48876=CARTESIAN_POINT('Origin',(27.86875,-0.565685424949239,43.0343145750508)) ;
#48877=CARTESIAN_POINT('Origin',(27.86875,-0.565685424949239,43.0343145750508)) ;
#48878=CARTESIAN_POINT('Origin',(27.840625,-0.682842712474618,43.3171572875254)) ;
#48879=CARTESIAN_POINT('',(27.6633431715058,-0.793856512305451,43.5851683086875)) ;
#48880=CARTESIAN_POINT('',(27.6912539970792,-0.677591388153184,43.3044794691282)) ;
#48881=CARTESIAN_POINT('Origin',(27.8125,-0.8,43.6)) ;
#48882=CARTESIAN_POINT('Origin',(27.8125,-0.8,43.6)) ;
#48883=CARTESIAN_POINT('Origin',(27.784375,-0.682842712474618,43.8828427124746)) ;
#48884=CARTESIAN_POINT('',(27.6070931715057,-0.571828912643784,44.1508537336368)) ;
#48885=CARTESIAN_POINT('',(27.6350039970792,-0.688094036796051,43.8701648940774)) ;
#48886=CARTESIAN_POINT('Origin',(27.75625,-0.565685424949235,44.1656854249492)) ;
#48887=CARTESIAN_POINT('Origin',(27.75625,-0.565685424949235,44.1656854249492)) ;
#48888=CARTESIAN_POINT('Origin',(27.728125,-0.282842712474617,44.2828427124746)) ;
#48889=CARTESIAN_POINT('',(27.5508431715058,-0.0148316913124567,44.3938565123055)) ;
#48890=CARTESIAN_POINT('',(27.5787539970792,-0.295520530871841,44.2775913881532)) ;
#48891=CARTESIAN_POINT('Origin',(27.7,-1.94289029309402E-15,44.4)) ;
#48892=CARTESIAN_POINT('Origin',(27.7,-1.94289029309402E-15,44.4)) ;
#48893=CARTESIAN_POINT('Origin',(27.671875,0.28284271247462,44.2828427124746)) ;
#48894=CARTESIAN_POINT('',(27.4945931715057,0.550853733636784,44.1718289126438)) ;
#48895=CARTESIAN_POINT('',(27.5225039970792,0.270164894077395,44.2880940367961)) ;
#48896=CARTESIAN_POINT('Origin',(27.64375,0.565685424949235,44.1656854249492)) ;
#48897=CARTESIAN_POINT('Origin',(27.64375,0.565685424949235,44.1656854249492)) ;
#48898=CARTESIAN_POINT('Origin',(27.615625,0.682842712474619,43.8828427124746)) ;
#48899=CARTESIAN_POINT('',(27.4383431715057,0.79385651230545,43.6148316913124)) ;
#48900=CARTESIAN_POINT('',(27.4662539970792,0.677591388153186,43.8955205308718)) ;
#48901=CARTESIAN_POINT('Origin',(27.5875,0.799999999999999,43.6)) ;
#48902=CARTESIAN_POINT('Origin',(27.5875,0.799999999999999,43.6)) ;
#48903=CARTESIAN_POINT('Origin',(27.559375,0.682842712474619,43.3171572875254)) ;
#48904=CARTESIAN_POINT('',(27.3820931715058,0.571828912643791,43.0491462663632)) ;
#48905=CARTESIAN_POINT('',(27.4100039970792,0.688094036796052,43.3298351059226)) ;
#48906=CARTESIAN_POINT('Origin',(27.53125,0.565685424949239,43.0343145750508)) ;
#48907=CARTESIAN_POINT('Origin',(27.53125,0.565685424949239,43.0343145750508)) ;
#48908=CARTESIAN_POINT('Origin',(27.503125,0.282842712474616,42.9171572875254)) ;
#48909=CARTESIAN_POINT('',(27.3258431715058,0.0148316913124495,42.8061434876946)) ;
#48910=CARTESIAN_POINT('',(27.3537539970792,0.29552053087184,42.9224086118468)) ;
#48911=CARTESIAN_POINT('Origin',(27.475,-4.49640324973188E-15,42.8)) ;
#48912=CARTESIAN_POINT('Origin',(27.475,-4.49640324973188E-15,42.8)) ;
#48913=CARTESIAN_POINT('Origin',(27.446875,-0.282842712474622,42.9171572875254)) ;
#48914=CARTESIAN_POINT('',(27.2695931715058,-0.550853733636784,43.0281710873562)) ;
#48915=CARTESIAN_POINT('',(27.2975039970792,-0.270164894077398,42.9119059632039)) ;
#48916=CARTESIAN_POINT('Origin',(27.41875,-0.56568542494924,43.0343145750508)) ;
#48917=CARTESIAN_POINT('Origin',(27.41875,-0.56568542494924,43.0343145750508)) ;
#48918=CARTESIAN_POINT('Origin',(27.390625,-0.68284271247462,43.3171572875254)) ;
#48919=CARTESIAN_POINT('',(27.2133431715057,-0.793856512305449,43.5851683086875)) ;
#48920=CARTESIAN_POINT('',(27.2412539970792,-0.677591388153186,43.3044794691282)) ;
#48921=CARTESIAN_POINT('Origin',(27.3625,-0.8,43.6)) ;
#48922=CARTESIAN_POINT('Origin',(27.3625,-0.8,43.6)) ;
#48923=CARTESIAN_POINT('Origin',(27.334375,-0.682842712474618,43.8828427124746)) ;
#48924=CARTESIAN_POINT('',(27.1570931715057,-0.571828912643786,44.1508537336368)) ;
#48925=CARTESIAN_POINT('',(27.1850039970792,-0.688094036796051,43.8701648940774)) ;
#48926=CARTESIAN_POINT('Origin',(27.30625,-0.565685424949237,44.1656854249492)) ;
#48927=CARTESIAN_POINT('Origin',(27.30625,-0.565685424949237,44.1656854249492)) ;
#48928=CARTESIAN_POINT('Origin',(27.278125,-0.282842712474617,44.2828427124746)) ;
#48929=CARTESIAN_POINT('',(27.1008431715058,-0.0148316913124573,44.3938565123055)) ;
#48930=CARTESIAN_POINT('',(27.1287539970792,-0.295520530871842,44.2775913881532)) ;
#48931=CARTESIAN_POINT('Origin',(27.25,-2.55351295663786E-15,44.4)) ;
#48932=CARTESIAN_POINT('Origin',(27.25,-2.55351295663786E-15,44.4)) ;
#48933=CARTESIAN_POINT('Origin',(27.221875,0.28284271247462,44.2828427124746)) ;
#48934=CARTESIAN_POINT('',(27.0445931715057,0.550853733636785,44.1718289126438)) ;
#48935=CARTESIAN_POINT('',(27.0725039970792,0.270164894077396,44.2880940367961)) ;
#48936=CARTESIAN_POINT('Origin',(27.19375,0.565685424949235,44.1656854249492)) ;
#48937=CARTESIAN_POINT('Origin',(27.19375,0.565685424949235,44.1656854249492)) ;
#48938=CARTESIAN_POINT('Origin',(27.165625,0.682842712474619,43.8828427124746)) ;
#48939=CARTESIAN_POINT('',(26.9883431715058,0.793856512305447,43.6148316913124)) ;
#48940=CARTESIAN_POINT('',(27.0162539970792,0.677591388153186,43.8955205308718)) ;
#48941=CARTESIAN_POINT('Origin',(27.1375,0.799999999999999,43.6)) ;
#48942=CARTESIAN_POINT('Origin',(27.1375,0.799999999999999,43.6)) ;
#48943=CARTESIAN_POINT('Origin',(27.109375,0.682842712474619,43.3171572875254)) ;
#48944=CARTESIAN_POINT('',(26.9320931715058,0.571828912643791,43.0491462663632)) ;
#48945=CARTESIAN_POINT('',(26.9600039970792,0.688094036796053,43.3298351059226)) ;
#48946=CARTESIAN_POINT('Origin',(27.08125,0.565685424949239,43.0343145750508)) ;
#48947=CARTESIAN_POINT('Origin',(27.08125,0.565685424949239,43.0343145750508)) ;
#48948=CARTESIAN_POINT('Origin',(27.053125,0.282842712474619,42.9171572875254)) ;
#48949=CARTESIAN_POINT('',(26.8758431715058,0.0148316913124561,42.8061434876946)) ;
#48950=CARTESIAN_POINT('',(26.9037539970792,0.295520530871843,42.9224086118468)) ;
#48951=CARTESIAN_POINT('Origin',(27.025,1.49880108324396E-15,42.8)) ;
#48952=CARTESIAN_POINT('Origin',(27.025,1.49880108324396E-15,42.8)) ;
#48953=CARTESIAN_POINT('Origin',(26.996875,-0.282842712474619,42.9171572875254)) ;
#48954=CARTESIAN_POINT('',(26.8195931715057,-0.550853733636788,43.0281710873562)) ;
#48955=CARTESIAN_POINT('',(26.8475039970792,-0.270164894077394,42.9119059632039)) ;
#48956=CARTESIAN_POINT('Origin',(26.96875,-0.56568542494924,43.0343145750508)) ;
#48957=CARTESIAN_POINT('Origin',(26.96875,-0.56568542494924,43.0343145750508)) ;
#48958=CARTESIAN_POINT('Origin',(26.940625,-0.68284271247462,43.3171572875254)) ;
#48959=CARTESIAN_POINT('',(26.7633431715058,-0.79385651230545,43.5851683086875)) ;
#48960=CARTESIAN_POINT('',(26.7912539970792,-0.677591388153187,43.3044794691282)) ;
#48961=CARTESIAN_POINT('Origin',(26.9125,-0.8,43.6)) ;
#48962=CARTESIAN_POINT('Origin',(26.9125,-0.8,43.6)) ;
#48963=CARTESIAN_POINT('Origin',(26.884375,-0.682842712474618,43.8828427124746)) ;
#48964=CARTESIAN_POINT('',(26.7070931715058,-0.571828912643786,44.1508537336368)) ;
#48965=CARTESIAN_POINT('',(26.7350039970792,-0.688094036796051,43.8701648940774)) ;
#48966=CARTESIAN_POINT('Origin',(26.85625,-0.565685424949237,44.1656854249492)) ;
#48967=CARTESIAN_POINT('Origin',(26.85625,-0.565685424949237,44.1656854249492)) ;
#48968=CARTESIAN_POINT('Origin',(26.828125,-0.282842712474617,44.2828427124746)) ;
#48969=CARTESIAN_POINT('',(26.6508431715058,-0.0148316913124579,44.3938565123055)) ;
#48970=CARTESIAN_POINT('',(26.6787539970792,-0.295520530871842,44.2775913881532)) ;
#48971=CARTESIAN_POINT('Origin',(26.8,-2.99760216648792E-15,44.4)) ;
#48972=CARTESIAN_POINT('Origin',(26.8,-2.99760216648792E-15,44.4)) ;
#48973=CARTESIAN_POINT('Origin',(26.771875,0.28284271247462,44.2828427124746)) ;
#48974=CARTESIAN_POINT('',(26.5945931715058,0.550853733636778,44.1718289126438)) ;
#48975=CARTESIAN_POINT('',(26.6225039970792,0.270164894077396,44.2880940367961)) ;
#48976=CARTESIAN_POINT('Origin',(26.74375,0.565685424949235,44.1656854249492)) ;
#48977=CARTESIAN_POINT('Origin',(26.74375,0.565685424949235,44.1656854249492)) ;
#48978=CARTESIAN_POINT('Origin',(26.715625,0.682842712474619,43.8828427124746)) ;
#48979=CARTESIAN_POINT('',(26.5383431715058,0.79385651230545,43.6148316913124)) ;
#48980=CARTESIAN_POINT('',(26.5662539970792,0.677591388153185,43.8955205308718)) ;
#48981=CARTESIAN_POINT('Origin',(26.6875,0.799999999999999,43.6)) ;
#48982=CARTESIAN_POINT('Origin',(26.6875,0.799999999999999,43.6)) ;
#48983=CARTESIAN_POINT('Origin',(26.659375,0.682842712474619,43.3171572875254)) ;
#48984=CARTESIAN_POINT('',(26.4820931715057,0.571828912643788,43.0491462663632)) ;
#48985=CARTESIAN_POINT('',(26.5100039970792,0.688094036796052,43.3298351059226)) ;
#48986=CARTESIAN_POINT('Origin',(26.63125,0.565685424949239,43.0343145750508)) ;
#48987=CARTESIAN_POINT('Origin',(26.63125,0.565685424949239,43.0343145750508)) ;
#48988=CARTESIAN_POINT('Origin',(26.603125,0.282842712474617,42.9171572875254)) ;
#48989=CARTESIAN_POINT('',(26.4258431715058,0.0148316913124502,42.8061434876946)) ;
#48990=CARTESIAN_POINT('',(26.4537539970792,0.295520530871841,42.9224086118468)) ;
#48991=CARTESIAN_POINT('Origin',(26.575,-4.44089209850063E-15,42.8)) ;
#48992=CARTESIAN_POINT('Origin',(26.575,-4.44089209850063E-15,42.8)) ;
#48993=CARTESIAN_POINT('Origin',(26.546875,-0.282842712474622,42.9171572875254)) ;
#48994=CARTESIAN_POINT('',(26.3695931715057,-0.550853733636787,43.0281710873562)) ;
#48995=CARTESIAN_POINT('',(26.3975039970792,-0.270164894077397,42.9119059632039)) ;
#48996=CARTESIAN_POINT('Origin',(26.51875,-0.565685424949239,43.0343145750508)) ;
#48997=CARTESIAN_POINT('Origin',(26.51875,-0.565685424949239,43.0343145750508)) ;
#48998=CARTESIAN_POINT('Origin',(26.490625,-0.68284271247462,43.3171572875254)) ;
#48999=CARTESIAN_POINT('',(26.3133431715058,-0.79385651230545,43.5851683086875)) ;
#49000=CARTESIAN_POINT('',(26.3412539970792,-0.677591388153186,43.3044794691282)) ;
#49001=CARTESIAN_POINT('Origin',(26.4625,-0.8,43.6)) ;
#49002=CARTESIAN_POINT('Origin',(26.4625,-0.8,43.6)) ;
#49003=CARTESIAN_POINT('Origin',(26.434375,-0.682842712474618,43.8828427124746)) ;
#49004=CARTESIAN_POINT('',(26.2570931715058,-0.571828912643789,44.1508537336368)) ;
#49005=CARTESIAN_POINT('',(26.2850039970792,-0.688094036796051,43.8701648940774)) ;
#49006=CARTESIAN_POINT('Origin',(26.40625,-0.565685424949237,44.1656854249492)) ;
#49007=CARTESIAN_POINT('Origin',(26.40625,-0.565685424949237,44.1656854249492)) ;
#49008=CARTESIAN_POINT('Origin',(26.378125,-0.282842712474617,44.2828427124746)) ;
#49009=CARTESIAN_POINT('',(26.2008431715058,-0.0148316913124567,44.3938565123055)) ;
#49010=CARTESIAN_POINT('',(26.2287539970792,-0.295520530871841,44.2775913881532)) ;
#49011=CARTESIAN_POINT('Origin',(26.35,-2.66453525910038E-15,44.4)) ;
#49012=CARTESIAN_POINT('Origin',(26.35,-2.66453525910038E-15,44.4)) ;
#49013=CARTESIAN_POINT('Origin',(26.321875,0.282842712474619,44.2828427124746)) ;
#49014=CARTESIAN_POINT('',(26.1445931715058,0.550853733636787,44.1718289126438)) ;
#49015=CARTESIAN_POINT('',(26.1725039970792,0.270164894077395,44.2880940367961)) ;
#49016=CARTESIAN_POINT('Origin',(26.29375,0.565685424949241,44.1656854249492)) ;
#49017=CARTESIAN_POINT('Origin',(26.29375,0.565685424949241,44.1656854249492)) ;
#49018=CARTESIAN_POINT('Origin',(26.265625,0.682842712474619,43.8828427124746)) ;
#49019=CARTESIAN_POINT('',(26.0883431715058,0.79385651230545,43.6148316913125)) ;
#49020=CARTESIAN_POINT('',(26.1162539970792,0.677591388153185,43.8955205308718)) ;
#49021=CARTESIAN_POINT('Origin',(26.2375,0.8,43.6)) ;
#49022=CARTESIAN_POINT('Origin',(26.2375,0.8,43.6)) ;
#49023=CARTESIAN_POINT('Origin',(26.209375,0.682842712474619,43.3171572875254)) ;
#49024=CARTESIAN_POINT('',(26.0320931715057,0.571828912643787,43.0491462663632)) ;
#49025=CARTESIAN_POINT('',(26.0600039970792,0.688094036796052,43.3298351059226)) ;
#49026=CARTESIAN_POINT('Origin',(26.18125,0.565685424949238,43.0343145750508)) ;
#49027=CARTESIAN_POINT('Origin',(26.18125,0.565685424949238,43.0343145750508)) ;
#49028=CARTESIAN_POINT('Origin',(26.153125,0.28284271247462,42.9171572875254)) ;
#49029=CARTESIAN_POINT('',(25.9758431715058,0.0148316913124558,42.8061434876946)) ;
#49030=CARTESIAN_POINT('',(26.0037539970792,0.295520530871845,42.9224086118468)) ;
#49031=CARTESIAN_POINT('Origin',(26.125,1.33226762955019E-15,42.8)) ;
#49032=CARTESIAN_POINT('Origin',(26.125,1.33226762955019E-15,42.8)) ;
#49033=CARTESIAN_POINT('Origin',(26.096875,-0.282842712474619,42.9171572875254)) ;
#49034=CARTESIAN_POINT('',(25.9195931715057,-0.550853733636788,43.0281710873562)) ;
#49035=CARTESIAN_POINT('',(25.9475039970792,-0.270164894077395,42.9119059632039)) ;
#49036=CARTESIAN_POINT('Origin',(26.06875,-0.565685424949239,43.0343145750508)) ;
#49037=CARTESIAN_POINT('Origin',(26.06875,-0.565685424949239,43.0343145750508)) ;
#49038=CARTESIAN_POINT('Origin',(26.040625,-0.68284271247462,43.3171572875254)) ;
#49039=CARTESIAN_POINT('',(25.8633431715058,-0.79385651230545,43.5851683086875)) ;
#49040=CARTESIAN_POINT('',(25.8912539970792,-0.677591388153186,43.3044794691282)) ;
#49041=CARTESIAN_POINT('Origin',(26.0125,-0.8,43.6)) ;
#49042=CARTESIAN_POINT('Origin',(26.0125,-0.8,43.6)) ;
#49043=CARTESIAN_POINT('Origin',(25.984375,-0.682842712474618,43.8828427124746)) ;
#49044=CARTESIAN_POINT('',(25.8070931715058,-0.571828912643789,44.1508537336368)) ;
#49045=CARTESIAN_POINT('',(25.8350039970792,-0.688094036796052,43.8701648940774)) ;
#49046=CARTESIAN_POINT('Origin',(25.95625,-0.565685424949237,44.1656854249492)) ;
#49047=CARTESIAN_POINT('Origin',(25.95625,-0.565685424949237,44.1656854249492)) ;
#49048=CARTESIAN_POINT('Origin',(25.928125,-0.282842712474617,44.2828427124746)) ;
#49049=CARTESIAN_POINT('',(25.7508431715058,-0.0148316913124584,44.3938565123055)) ;
#49050=CARTESIAN_POINT('',(25.7787539970792,-0.295520530871841,44.2775913881532)) ;
#49051=CARTESIAN_POINT('Origin',(25.9,-3.44169137633799E-15,44.4)) ;
#49052=CARTESIAN_POINT('Origin',(25.9,-3.44169137633799E-15,44.4)) ;
#49053=CARTESIAN_POINT('Origin',(25.871875,0.282842712474619,44.2828427124746)) ;
#49054=CARTESIAN_POINT('',(25.6945931715057,0.550853733636793,44.1718289126438)) ;
#49055=CARTESIAN_POINT('',(25.7225039970792,0.270164894077394,44.2880940367961)) ;
#49056=CARTESIAN_POINT('Origin',(25.84375,0.565685424949241,44.1656854249492)) ;
#49057=CARTESIAN_POINT('Origin',(25.84375,0.565685424949241,44.1656854249492)) ;
#49058=CARTESIAN_POINT('Origin',(25.815625,0.682842712474619,43.8828427124746)) ;
#49059=CARTESIAN_POINT('',(25.6383431715058,0.79385651230545,43.6148316913125)) ;
#49060=CARTESIAN_POINT('',(25.6662539970792,0.677591388153185,43.8955205308718)) ;
#49061=CARTESIAN_POINT('Origin',(25.7875,0.8,43.6)) ;
#49062=CARTESIAN_POINT('Origin',(25.7875,0.8,43.6)) ;
#49063=CARTESIAN_POINT('Origin',(25.759375,0.682842712474619,43.3171572875254)) ;
#49064=CARTESIAN_POINT('',(25.5820931715058,0.571828912643787,43.0491462663632)) ;
#49065=CARTESIAN_POINT('',(25.6100039970792,0.688094036796052,43.3298351059226)) ;
#49066=CARTESIAN_POINT('Origin',(25.73125,0.565685424949238,43.0343145750508)) ;
#49067=CARTESIAN_POINT('Origin',(25.73125,0.565685424949238,43.0343145750508)) ;
#49068=CARTESIAN_POINT('Origin',(25.703125,0.282842712474617,42.9171572875254)) ;
#49069=CARTESIAN_POINT('',(25.5258431715058,0.0148316913124512,42.8061434876946)) ;
#49070=CARTESIAN_POINT('',(25.5537539970792,0.295520530871842,42.9224086118468)) ;
#49071=CARTESIAN_POINT('Origin',(25.675,-3.60822483003176E-15,42.8)) ;
#49072=CARTESIAN_POINT('Origin',(25.675,-3.60822483003176E-15,42.8)) ;
#49073=CARTESIAN_POINT('Origin',(25.646875,-0.282842712474622,42.9171572875254)) ;
#49074=CARTESIAN_POINT('',(25.4695931715058,-0.550853733636783,43.0281710873562)) ;
#49075=CARTESIAN_POINT('',(25.4975039970792,-0.270164894077397,42.9119059632039)) ;
#49076=CARTESIAN_POINT('Origin',(25.61875,-0.565685424949239,43.0343145750508)) ;
#49077=CARTESIAN_POINT('Origin',(25.61875,-0.565685424949239,43.0343145750508)) ;
#49078=CARTESIAN_POINT('Origin',(25.590625,-0.68284271247462,43.3171572875254)) ;
#49079=CARTESIAN_POINT('',(25.4133431715058,-0.793856512305449,43.5851683086875)) ;
#49080=CARTESIAN_POINT('',(25.4412539970792,-0.677591388153186,43.3044794691282)) ;
#49081=CARTESIAN_POINT('Origin',(25.5625,-0.8,43.6)) ;
#49082=CARTESIAN_POINT('Origin',(25.5625,-0.8,43.6)) ;
#49083=CARTESIAN_POINT('Origin',(25.534375,-0.682842712474618,43.8828427124746)) ;
#49084=CARTESIAN_POINT('',(25.3570931715057,-0.571828912643786,44.1508537336368)) ;
#49085=CARTESIAN_POINT('',(25.3850039970792,-0.688094036796051,43.8701648940774)) ;
#49086=CARTESIAN_POINT('Origin',(25.50625,-0.565685424949237,44.1656854249492)) ;
#49087=CARTESIAN_POINT('Origin',(25.50625,-0.565685424949237,44.1656854249492)) ;
#49088=CARTESIAN_POINT('Origin',(25.478125,-0.282842712474617,44.2828427124746)) ;
#49089=CARTESIAN_POINT('',(25.3008431715058,-0.0148316913124581,44.3938565123055)) ;
#49090=CARTESIAN_POINT('',(25.3287539970792,-0.295520530871842,44.2775913881532)) ;
#49091=CARTESIAN_POINT('Origin',(25.45,-3.38618022510673E-15,44.4)) ;
#49092=CARTESIAN_POINT('Origin',(25.45,-3.38618022510673E-15,44.4)) ;
#49093=CARTESIAN_POINT('Origin',(25.421875,0.28284271247462,44.2828427124746)) ;
#49094=CARTESIAN_POINT('',(25.2445931715057,0.550853733636795,44.1718289126438)) ;
#49095=CARTESIAN_POINT('',(25.2725039970792,0.270164894077395,44.2880940367961)) ;
#49096=CARTESIAN_POINT('Origin',(25.39375,0.565685424949243,44.1656854249492)) ;
#49097=CARTESIAN_POINT('Origin',(25.39375,0.565685424949243,44.1656854249492)) ;
#49098=CARTESIAN_POINT('Origin',(25.365625,0.68284271247462,43.8828427124746)) ;
#49099=CARTESIAN_POINT('',(25.1883431715058,0.79385651230545,43.6148316913125)) ;
#49100=CARTESIAN_POINT('',(25.2162539970792,0.677591388153186,43.8955205308718)) ;
#49101=CARTESIAN_POINT('Origin',(25.3375,0.8,43.6)) ;
#49102=CARTESIAN_POINT('Origin',(25.3375,0.8,43.6)) ;
#49103=CARTESIAN_POINT('Origin',(25.309375,0.682842712474619,43.3171572875254)) ;
#49104=CARTESIAN_POINT('',(25.1320931715058,0.57182891264379,43.0491462663632)) ;
#49105=CARTESIAN_POINT('',(25.1600039970792,0.688094036796053,43.3298351059226)) ;
#49106=CARTESIAN_POINT('Origin',(25.28125,0.565685424949238,43.0343145750508)) ;
#49107=CARTESIAN_POINT('Origin',(25.28125,0.565685424949238,43.0343145750508)) ;
#49108=CARTESIAN_POINT('Origin',(25.253125,0.282842712474619,42.9171572875254)) ;
#49109=CARTESIAN_POINT('',(25.0758431715058,0.0148316913124534,42.8061434876946)) ;
#49110=CARTESIAN_POINT('',(25.1037539970792,0.295520530871843,42.9224086118468)) ;
#49111=CARTESIAN_POINT('Origin',(25.225,-5.55111512312578E-16,42.8)) ;
#49112=CARTESIAN_POINT('Origin',(25.225,-5.55111512312578E-16,42.8)) ;
#49113=CARTESIAN_POINT('Origin',(25.196875,-0.28284271247462,42.9171572875254)) ;
#49114=CARTESIAN_POINT('',(25.0195931715058,-0.550853733636783,43.0281710873562)) ;
#49115=CARTESIAN_POINT('',(25.0475039970792,-0.270164894077396,42.9119059632039)) ;
#49116=CARTESIAN_POINT('Origin',(25.16875,-0.565685424949239,43.0343145750508)) ;
#49117=CARTESIAN_POINT('Origin',(25.16875,-0.565685424949239,43.0343145750508)) ;
#49118=CARTESIAN_POINT('Origin',(25.140625,-0.68284271247462,43.3171572875254)) ;
#49119=CARTESIAN_POINT('',(24.9633431715058,-0.79385651230545,43.5851683086875)) ;
#49120=CARTESIAN_POINT('',(24.9912539970792,-0.677591388153186,43.3044794691282)) ;
#49121=CARTESIAN_POINT('Origin',(25.1125,-0.8,43.6)) ;
#49122=CARTESIAN_POINT('Origin',(25.1125,-0.8,43.6)) ;
#49123=CARTESIAN_POINT('Origin',(25.084375,-0.682842712474619,43.8828427124746)) ;
#49124=CARTESIAN_POINT('',(24.9070931715057,-0.571828912643791,44.1508537336368)) ;
#49125=CARTESIAN_POINT('',(24.9350039970792,-0.688094036796052,43.8701648940774)) ;
#49126=CARTESIAN_POINT('Origin',(25.05625,-0.565685424949241,44.1656854249492)) ;
#49127=CARTESIAN_POINT('Origin',(25.05625,-0.565685424949241,44.1656854249492)) ;
#49128=CARTESIAN_POINT('Origin',(25.028125,-0.282842712474619,44.2828427124746)) ;
#49129=CARTESIAN_POINT('',(24.8508431715058,-0.0148316913124536,44.3938565123055)) ;
#49130=CARTESIAN_POINT('',(24.8787539970792,-0.295520530871843,44.2775913881532)) ;
#49131=CARTESIAN_POINT('Origin',(25.,8.88178419700125E-16,44.4)) ;
#49132=CARTESIAN_POINT('Origin',(25.,8.88178419700125E-16,44.4)) ;
#49133=CARTESIAN_POINT('Origin',(24.971875,0.28284271247462,44.2828427124746)) ;
#49134=CARTESIAN_POINT('',(24.7945931715057,0.550853733636796,44.1718289126438)) ;
#49135=CARTESIAN_POINT('',(24.8225039970792,0.270164894077396,44.2880940367961)) ;
#49136=CARTESIAN_POINT('Origin',(24.94375,0.565685424949243,44.1656854249492)) ;
#49137=CARTESIAN_POINT('Origin',(24.94375,0.565685424949243,44.1656854249492)) ;
#49138=CARTESIAN_POINT('Origin',(24.915625,0.682842712474619,43.8828427124746)) ;
#49139=CARTESIAN_POINT('',(24.7383431715058,0.79385651230545,43.6148316913125)) ;
#49140=CARTESIAN_POINT('',(24.7662539970792,0.677591388153186,43.8955205308718)) ;
#49141=CARTESIAN_POINT('Origin',(24.8875,0.8,43.6)) ;
#49142=CARTESIAN_POINT('Origin',(24.8875,0.8,43.6)) ;
#49143=CARTESIAN_POINT('Origin',(24.859375,0.682842712474619,43.3171572875254)) ;
#49144=CARTESIAN_POINT('',(24.6820931715058,0.57182891264379,43.0491462663632)) ;
#49145=CARTESIAN_POINT('',(24.7100039970792,0.688094036796053,43.3298351059226)) ;
#49146=CARTESIAN_POINT('Origin',(24.83125,0.565685424949238,43.0343145750508)) ;
#49147=CARTESIAN_POINT('Origin',(24.83125,0.565685424949238,43.0343145750508)) ;
#49148=CARTESIAN_POINT('Origin',(24.803125,0.282842712474619,42.9171572875254)) ;
#49149=CARTESIAN_POINT('',(24.6258431715058,0.0148316913124541,42.8061434876946)) ;
#49150=CARTESIAN_POINT('',(24.6537539970792,0.295520530871843,42.9224086118468)) ;
#49151=CARTESIAN_POINT('Origin',(24.775,-7.21644966006352E-16,42.8)) ;
#49152=CARTESIAN_POINT('Origin',(24.775,-7.21644966006352E-16,42.8)) ;
#49153=CARTESIAN_POINT('Origin',(24.746875,-0.28284271247462,42.9171572875254)) ;
#49154=CARTESIAN_POINT('',(24.5695931715057,-0.550853733636787,43.0281710873562)) ;
#49155=CARTESIAN_POINT('',(24.5975039970792,-0.270164894077395,42.9119059632039)) ;
#49156=CARTESIAN_POINT('Origin',(24.71875,-0.565685424949239,43.0343145750508)) ;
#49157=CARTESIAN_POINT('Origin',(24.71875,-0.565685424949239,43.0343145750508)) ;
#49158=CARTESIAN_POINT('Origin',(24.690625,-0.682842712474619,43.3171572875254)) ;
#49159=CARTESIAN_POINT('',(24.5133431715058,-0.79385651230545,43.5851683086875)) ;
#49160=CARTESIAN_POINT('',(24.5412539970792,-0.677591388153186,43.3044794691282)) ;
#49161=CARTESIAN_POINT('Origin',(24.6625,-0.8,43.6)) ;
#49162=CARTESIAN_POINT('Origin',(24.6625,-0.8,43.6)) ;
#49163=CARTESIAN_POINT('Origin',(24.634375,-0.682842712474619,43.8828427124746)) ;
#49164=CARTESIAN_POINT('',(24.4570931715058,-0.57182891264379,44.1508537336368)) ;
#49165=CARTESIAN_POINT('',(24.4850039970792,-0.688094036796052,43.8701648940774)) ;
#49166=CARTESIAN_POINT('Origin',(24.60625,-0.565685424949241,44.1656854249492)) ;
#49167=CARTESIAN_POINT('Origin',(24.60625,-0.565685424949241,44.1656854249492)) ;
#49168=CARTESIAN_POINT('Origin',(24.578125,-0.282842712474619,44.2828427124746)) ;
#49169=CARTESIAN_POINT('',(24.4008431715058,-0.0148316913124548,44.3938565123055)) ;
#49170=CARTESIAN_POINT('',(24.4287539970792,-0.295520530871844,44.2775913881532)) ;
#49171=CARTESIAN_POINT('Origin',(24.55,5.55111512312578E-17,44.4)) ;
#49172=CARTESIAN_POINT('Origin',(24.55,5.55111512312578E-17,44.4)) ;
#49173=CARTESIAN_POINT('Origin',(24.521875,0.28284271247462,44.2828427124746)) ;
#49174=CARTESIAN_POINT('',(24.3445931715058,0.550853733636791,44.1718289126438)) ;
#49175=CARTESIAN_POINT('',(24.3725039970792,0.270164894077396,44.2880940367961)) ;
#49176=CARTESIAN_POINT('Origin',(24.49375,0.565685424949243,44.1656854249492)) ;
#49177=CARTESIAN_POINT('Origin',(24.49375,0.565685424949243,44.1656854249492)) ;
#49178=CARTESIAN_POINT('Origin',(24.465625,0.682842712474619,43.8828427124746)) ;
#49179=CARTESIAN_POINT('',(24.2883431715058,0.793856512305449,43.6148316913125)) ;
#49180=CARTESIAN_POINT('',(24.3162539970792,0.677591388153186,43.8955205308718)) ;
#49181=CARTESIAN_POINT('Origin',(24.4375,0.8,43.6)) ;
#49182=CARTESIAN_POINT('Origin',(24.4375,0.8,43.6)) ;
#49183=CARTESIAN_POINT('Origin',(24.409375,0.682842712474619,43.3171572875254)) ;
#49184=CARTESIAN_POINT('',(24.2320931715057,0.571828912643786,43.0491462663632)) ;
#49185=CARTESIAN_POINT('',(24.2600039970792,0.688094036796052,43.3298351059226)) ;
#49186=CARTESIAN_POINT('Origin',(24.38125,0.565685424949238,43.0343145750508)) ;
#49187=CARTESIAN_POINT('Origin',(24.38125,0.565685424949238,43.0343145750508)) ;
#49188=CARTESIAN_POINT('Origin',(24.353125,0.282842712474619,42.9171572875254)) ;
#49189=CARTESIAN_POINT('',(24.1758431715058,0.0148316913124543,42.8061434876946)) ;
#49190=CARTESIAN_POINT('',(24.2037539970792,0.295520530871843,42.9224086118468)) ;
#49191=CARTESIAN_POINT('Origin',(24.325,-2.77555756156289E-16,42.8)) ;
#49192=CARTESIAN_POINT('Origin',(24.325,-2.77555756156289E-16,42.8)) ;
#49193=CARTESIAN_POINT('Origin',(24.296875,-0.28284271247462,42.9171572875254)) ;
#49194=CARTESIAN_POINT('',(24.1195931715057,-0.550853733636786,43.0281710873562)) ;
#49195=CARTESIAN_POINT('',(24.1475039970792,-0.270164894077395,42.9119059632039)) ;
#49196=CARTESIAN_POINT('Origin',(24.26875,-0.565685424949238,43.0343145750508)) ;
#49197=CARTESIAN_POINT('Origin',(24.26875,-0.565685424949238,43.0343145750508)) ;
#49198=CARTESIAN_POINT('Origin',(24.240625,-0.682842712474619,43.3171572875254)) ;
#49199=CARTESIAN_POINT('',(24.0633431715058,-0.79385651230545,43.5851683086875)) ;
#49200=CARTESIAN_POINT('',(24.0912539970792,-0.677591388153186,43.3044794691282)) ;
#49201=CARTESIAN_POINT('Origin',(24.2125,-0.8,43.6)) ;
#49202=CARTESIAN_POINT('Origin',(24.2125,-0.8,43.6)) ;
#49203=CARTESIAN_POINT('Origin',(24.184375,-0.682842712474619,43.8828427124746)) ;
#49204=CARTESIAN_POINT('',(24.0070931715058,-0.571828912643794,44.1508537336368)) ;
#49205=CARTESIAN_POINT('',(24.0350039970792,-0.688094036796053,43.8701648940774)) ;
#49206=CARTESIAN_POINT('Origin',(24.15625,-0.565685424949241,44.1656854249492)) ;
#49207=CARTESIAN_POINT('Origin',(24.15625,-0.565685424949241,44.1656854249492)) ;
#49208=CARTESIAN_POINT('Origin',(24.128125,-0.282842712474619,44.2828427124746)) ;
#49209=CARTESIAN_POINT('',(23.9508431715058,-0.0148316913124537,44.3938565123055)) ;
#49210=CARTESIAN_POINT('',(23.9787539970792,-0.295520530871843,44.2775913881532)) ;
#49211=CARTESIAN_POINT('Origin',(24.1,3.33066907387547E-16,44.4)) ;
#49212=CARTESIAN_POINT('Origin',(24.1,3.33066907387547E-16,44.4)) ;
#49213=CARTESIAN_POINT('Origin',(24.071875,0.28284271247462,44.2828427124746)) ;
#49214=CARTESIAN_POINT('',(23.8945931715058,0.550853733636791,44.1718289126438)) ;
#49215=CARTESIAN_POINT('',(23.9225039970792,0.270164894077396,44.2880940367961)) ;
#49216=CARTESIAN_POINT('Origin',(24.04375,0.565685424949242,44.1656854249492)) ;
#49217=CARTESIAN_POINT('Origin',(24.04375,0.565685424949242,44.1656854249492)) ;
#49218=CARTESIAN_POINT('Origin',(24.015625,0.682842712474619,43.8828427124746)) ;
#49219=CARTESIAN_POINT('',(23.8383431715058,0.79385651230545,43.6148316913125)) ;
#49220=CARTESIAN_POINT('',(23.8662539970792,0.677591388153186,43.8955205308718)) ;
#49221=CARTESIAN_POINT('Origin',(23.9875,0.8,43.6)) ;
#49222=CARTESIAN_POINT('Origin',(23.9875,0.8,43.6)) ;
#49223=CARTESIAN_POINT('Origin',(23.959375,0.682842712474619,43.3171572875254)) ;
#49224=CARTESIAN_POINT('',(23.7820931715057,0.571828912643788,43.0491462663632)) ;
#49225=CARTESIAN_POINT('',(23.8100039970792,0.688094036796053,43.3298351059226)) ;
#49226=CARTESIAN_POINT('Origin',(23.93125,0.565685424949238,43.0343145750508)) ;
#49227=CARTESIAN_POINT('Origin',(23.93125,0.565685424949238,43.0343145750508)) ;
#49228=CARTESIAN_POINT('Origin',(23.903125,0.282842712474619,42.9171572875254)) ;
#49229=CARTESIAN_POINT('',(23.7258431715058,0.0148316913124538,42.8061434876946)) ;
#49230=CARTESIAN_POINT('',(23.7537539970792,0.295520530871844,42.9224086118468)) ;
#49231=CARTESIAN_POINT('Origin',(23.875,-6.66133814775094E-16,42.8)) ;
#49232=CARTESIAN_POINT('Origin',(23.875,-6.66133814775094E-16,42.8)) ;
#49233=CARTESIAN_POINT('Origin',(23.846875,-0.28284271247462,42.9171572875254)) ;
#49234=CARTESIAN_POINT('',(23.6695931715057,-0.550853733636787,43.0281710873562)) ;
#49235=CARTESIAN_POINT('',(23.6975039970792,-0.270164894077395,42.9119059632039)) ;
#49236=CARTESIAN_POINT('Origin',(23.81875,-0.565685424949239,43.0343145750508)) ;
#49237=CARTESIAN_POINT('Origin',(23.81875,-0.565685424949239,43.0343145750508)) ;
#49238=CARTESIAN_POINT('Origin',(23.790625,-0.682842712474619,43.3171572875254)) ;
#49239=CARTESIAN_POINT('',(23.6133431715058,-0.79385651230545,43.5851683086875)) ;
#49240=CARTESIAN_POINT('',(23.6412539970792,-0.677591388153186,43.3044794691282)) ;
#49241=CARTESIAN_POINT('Origin',(23.7625,-0.8,43.6)) ;
#49242=CARTESIAN_POINT('Origin',(23.7625,-0.8,43.6)) ;
#49243=CARTESIAN_POINT('Origin',(23.734375,-0.682842712474619,43.8828427124746)) ;
#49244=CARTESIAN_POINT('',(23.5570931715058,-0.571828912643793,44.1508537336368)) ;
#49245=CARTESIAN_POINT('',(23.5850039970792,-0.688094036796053,43.8701648940774)) ;
#49246=CARTESIAN_POINT('Origin',(23.70625,-0.565685424949241,44.1656854249492)) ;
#49247=CARTESIAN_POINT('Origin',(23.70625,-0.565685424949241,44.1656854249492)) ;
#49248=CARTESIAN_POINT('Origin',(23.678125,-0.282842712474619,44.2828427124746)) ;
#49249=CARTESIAN_POINT('',(23.5008431715058,-0.0148316913124547,44.3938565123055)) ;
#49250=CARTESIAN_POINT('',(23.5287539970792,-0.295520530871843,44.2775913881532)) ;
#49251=CARTESIAN_POINT('Origin',(23.65,1.66533453693773E-16,44.4)) ;
#49252=CARTESIAN_POINT('Origin',(23.65,1.66533453693773E-16,44.4)) ;
#49253=CARTESIAN_POINT('Origin',(23.621875,0.282842712474619,44.2828427124746)) ;
#49254=CARTESIAN_POINT('',(23.4445931715057,0.550853733636794,44.1718289126438)) ;
#49255=CARTESIAN_POINT('',(23.4725039970792,0.270164894077394,44.2880940367961)) ;
#49256=CARTESIAN_POINT('Origin',(23.59375,0.565685424949242,44.1656854249492)) ;
#49257=CARTESIAN_POINT('Origin',(23.59375,0.565685424949242,44.1656854249492)) ;
#49258=CARTESIAN_POINT('Origin',(23.565625,0.682842712474619,43.8828427124746)) ;
#49259=CARTESIAN_POINT('',(23.3883431715058,0.79385651230545,43.6148316913125)) ;
#49260=CARTESIAN_POINT('',(23.4162539970792,0.677591388153186,43.8955205308718)) ;
#49261=CARTESIAN_POINT('Origin',(23.5375,0.8,43.6)) ;
#49262=CARTESIAN_POINT('Origin',(23.5375,0.8,43.6)) ;
#49263=CARTESIAN_POINT('Origin',(23.509375,0.682842712474619,43.3171572875254)) ;
#49264=CARTESIAN_POINT('',(23.3320931715058,0.571828912643787,43.0491462663632)) ;
#49265=CARTESIAN_POINT('',(23.3600039970792,0.688094036796052,43.3298351059226)) ;
#49266=CARTESIAN_POINT('Origin',(23.48125,0.565685424949238,43.0343145750508)) ;
#49267=CARTESIAN_POINT('Origin',(23.48125,0.565685424949238,43.0343145750508)) ;
#49268=CARTESIAN_POINT('Origin',(23.453125,0.282842712474619,42.9171572875254)) ;
#49269=CARTESIAN_POINT('',(23.2758431715058,0.0148316913124553,42.8061434876946)) ;
#49270=CARTESIAN_POINT('',(23.3037539970792,0.295520530871844,42.9224086118468)) ;
#49271=CARTESIAN_POINT('Origin',(23.425,4.9960036108132E-16,42.8)) ;
#49272=CARTESIAN_POINT('Origin',(23.425,4.9960036108132E-16,42.8)) ;
#49273=CARTESIAN_POINT('Origin',(23.396875,-0.282842712474619,42.9171572875254)) ;
#49274=CARTESIAN_POINT('',(23.2195931715058,-0.550853733636782,43.0281710873562)) ;
#49275=CARTESIAN_POINT('',(23.2475039970792,-0.270164894077395,42.9119059632039)) ;
#49276=CARTESIAN_POINT('Origin',(23.36875,-0.565685424949238,43.0343145750508)) ;
#49277=CARTESIAN_POINT('Origin',(23.36875,-0.565685424949238,43.0343145750508)) ;
#49278=CARTESIAN_POINT('Origin',(23.340625,-0.682842712474619,43.3171572875254)) ;
#49279=CARTESIAN_POINT('',(23.1633431715058,-0.793856512305449,43.5851683086875)) ;
#49280=CARTESIAN_POINT('',(23.1912539970792,-0.677591388153185,43.3044794691282)) ;
#49281=CARTESIAN_POINT('Origin',(23.3125,-0.8,43.6)) ;
#49282=CARTESIAN_POINT('Origin',(23.3125,-0.8,43.6)) ;
#49283=CARTESIAN_POINT('Origin',(23.284375,-0.682842712474619,43.8828427124746)) ;
#49284=CARTESIAN_POINT('',(23.1070931715057,-0.57182891264379,44.1508537336368)) ;
#49285=CARTESIAN_POINT('',(23.1350039970792,-0.688094036796052,43.8701648940774)) ;
#49286=CARTESIAN_POINT('Origin',(23.25625,-0.565685424949241,44.1656854249492)) ;
#49287=CARTESIAN_POINT('Origin',(23.25625,-0.565685424949241,44.1656854249492)) ;
#49288=CARTESIAN_POINT('Origin',(23.228125,-0.282842712474619,44.2828427124746)) ;
#49289=CARTESIAN_POINT('',(23.0506289970792,-0.0126778183972212,44.3947486756786)) ;
#49290=CARTESIAN_POINT('',(23.0787539970792,-0.295520530871843,44.2775913881532)) ;
#49291=CARTESIAN_POINT('Origin',(23.2,0.,44.4)) ;
#49292=CARTESIAN_POINT('Origin',(23.2,0.,44.4)) ;
#49293=CARTESIAN_POINT('Origin',(31.9,0.,43.2)) ;
#49294=CARTESIAN_POINT('',(31.35,-6.73555739531044E-17,43.6)) ;
#49295=CARTESIAN_POINT('Origin',(31.9,0.,43.6)) ;
#49296=CARTESIAN_POINT('',(31.35,-5.36271069502855E-17,43.4747805496751)) ;
#49297=CARTESIAN_POINT('',(31.35,-6.73555739531044E-17,43.2)) ;
#49298=CARTESIAN_POINT('',(31.35,-1.6551677115079E-16,43.1585527836583)) ;
#49299=CARTESIAN_POINT('Ctrl Pts',(31.35,-2.63677968348475E-16,43.1585527836583)) ;
#49300=CARTESIAN_POINT('Ctrl Pts',(31.35,-0.0188191332662162,43.1585527836583)) ;
#49301=CARTESIAN_POINT('Ctrl Pts',(31.3510631096512,-0.0388916191458831,
43.1621613787556)) ;
#49302=CARTESIAN_POINT('Ctrl Pts',(31.3549322157784,-0.0757982758665373,
43.1769669116142)) ;
#49303=CARTESIAN_POINT('Ctrl Pts',(31.3576877759068,-0.0926307743041964,
43.1881811506715)) ;
#49304=CARTESIAN_POINT('Ctrl Pts',(31.3629682744752,-0.119540791091898,
43.2147010690475)) ;
#49305=CARTESIAN_POINT('Ctrl Pts',(31.3658184898934,-0.131194409953506,
43.2318737514959)) ;
#49306=CARTESIAN_POINT('Ctrl Pts',(31.3697883951301,-0.146415562473201,
43.2697170608075)) ;
#49307=CARTESIAN_POINT('Ctrl Pts',(31.3708497377871,-0.15,43.2903869851339)) ;
#49308=CARTESIAN_POINT('Ctrl Pts',(31.3708497377871,-0.15,43.3299223679419)) ;
#49309=CARTESIAN_POINT('Ctrl Pts',(31.3697109017808,-0.146136718812717,
43.3514677287737)) ;
#49310=CARTESIAN_POINT('Ctrl Pts',(31.3657306796926,-0.130838683604474,
43.3915453490939)) ;
#49311=CARTESIAN_POINT('Ctrl Pts',(31.3629471493545,-0.1194120242323,43.4100864224367)) ;
#49312=CARTESIAN_POINT('Ctrl Pts',(31.3577971876893,-0.093208439870651,
43.4394240794729)) ;
#49313=CARTESIAN_POINT('Ctrl Pts',(31.3550634167387,-0.0767307277487665,
43.4524660649886)) ;
#49314=CARTESIAN_POINT('Ctrl Pts',(31.3511342241156,-0.0398728705117728,
43.47016523252)) ;
#49315=CARTESIAN_POINT('Ctrl Pts',(31.35,-0.0194661400469685,43.4747805496751)) ;
#49316=CARTESIAN_POINT('Ctrl Pts',(31.35,-6.27969898303604E-16,43.4747805496751)) ;
#49317=CARTESIAN_POINT('',(31.35,-6.73555739531044E-17,42.8)) ;
#49318=CARTESIAN_POINT('',(31.35,-6.73555739531044E-17,43.2)) ;
#49319=CARTESIAN_POINT('Origin',(31.9,0.,42.8)) ;
#49320=CARTESIAN_POINT('',(31.3708497377871,0.15,43.309716754071)) ;
#49321=CARTESIAN_POINT('Ctrl Pts',(31.3708497377871,0.15,43.309716754071)) ;
#49322=CARTESIAN_POINT('Ctrl Pts',(31.3708497377871,0.15,43.2903869851339)) ;
#49323=CARTESIAN_POINT('Ctrl Pts',(31.3697883951301,0.146415562473201,43.2697170608075)) ;
#49324=CARTESIAN_POINT('Ctrl Pts',(31.3658184898934,0.131194409953506,43.2318737514959)) ;
#49325=CARTESIAN_POINT('Ctrl Pts',(31.3629682744752,0.119540791091898,43.2147010690475)) ;
#49326=CARTESIAN_POINT('Ctrl Pts',(31.3576877759068,0.0926307743041964,
43.1881811506715)) ;
#49327=CARTESIAN_POINT('Ctrl Pts',(31.3549322157784,0.0757982758665373,
43.1769669116142)) ;
#49328=CARTESIAN_POINT('Ctrl Pts',(31.3510631096512,0.0388916191458832,
43.1621613787556)) ;
#49329=CARTESIAN_POINT('Ctrl Pts',(31.35,0.0188191332662163,43.1585527836583)) ;
#49330=CARTESIAN_POINT('Ctrl Pts',(31.35,3.88578058618805E-16,43.1585527836583)) ;
#49331=CARTESIAN_POINT('Ctrl Pts',(31.35,-3.98986399474666E-17,43.4747805496751)) ;
#49332=CARTESIAN_POINT('Ctrl Pts',(31.35,0.0194661400469678,43.4747805496751)) ;
#49333=CARTESIAN_POINT('Ctrl Pts',(31.3511342241156,0.0398728705117756,
43.47016523252)) ;
#49334=CARTESIAN_POINT('Ctrl Pts',(31.3550634167387,0.0767307277487687,
43.4524660649886)) ;
#49335=CARTESIAN_POINT('Ctrl Pts',(31.3577971876893,0.0932084398706509,
43.4394240794729)) ;
#49336=CARTESIAN_POINT('Ctrl Pts',(31.3629471493545,0.1194120242323,43.4100864224367)) ;
#49337=CARTESIAN_POINT('Ctrl Pts',(31.3657306796926,0.130838683604474,43.3915453490939)) ;
#49338=CARTESIAN_POINT('Ctrl Pts',(31.3697109017808,0.146136718812717,43.3514677287737)) ;
#49339=CARTESIAN_POINT('Ctrl Pts',(31.3708497377871,0.15,43.3299223679419)) ;
#49340=CARTESIAN_POINT('Ctrl Pts',(31.3708497377871,0.15,43.309716754071)) ;
#49341=CARTESIAN_POINT('Origin',(31.9,0.,43.2)) ;
#49342=CARTESIAN_POINT('',(31.65,-3.06161699786838E-17,42.8)) ;
#49343=CARTESIAN_POINT('Origin',(31.9,0.,42.8)) ;
#49344=CARTESIAN_POINT('',(31.65,3.06161699786838E-17,43.6)) ;
#49345=CARTESIAN_POINT('',(31.65,-3.06161699786838E-17,43.2)) ;
#49346=CARTESIAN_POINT('Origin',(31.9,0.,43.6)) ;
#49347=CARTESIAN_POINT('Origin',(31.9,0.,42.8)) ;
#49348=CARTESIAN_POINT('Origin',(31.9,0.,43.6)) ;
#49349=CARTESIAN_POINT('Origin',(30.95,0.,43.45)) ;
#49350=CARTESIAN_POINT('',(30.4525658350975,1.83697019872103E-17,43.4576975052924)) ;
#49351=CARTESIAN_POINT('',(30.9025658350975,1.83697019872103E-17,43.3076975052924)) ;
#49352=CARTESIAN_POINT('Origin',(30.5,0.,43.6)) ;
#49353=CARTESIAN_POINT('Origin',(30.5,0.,43.6)) ;
#50372=UNCERTAINTY_MEASURE_WITH_UNIT(LENGTH_MEASURE(0.001),#50441,
'DISTANCE_ACCURACY_VALUE',
'Maximum model space distance between geometric entities at asserted c
onnectivities') ;
#50387=UNCERTAINTY_MEASURE_WITH_UNIT(LENGTH_MEASURE(0.001),#50441,
'DISTANCE_ACCURACY_VALUE',
'Maximum model space distance between geometric entities at asserted c
onnectivities') ;
#50425=(
GEOMETRIC_REPRESENTATION_CONTEXT(3)
GLOBAL_UNCERTAINTY_ASSIGNED_CONTEXT((#50372))
GLOBAL_UNIT_ASSIGNED_CONTEXT((#50441,#50443,#50444))
REPRESENTATION_CONTEXT('','3D')
) ;
#50440=(
GEOMETRIC_REPRESENTATION_CONTEXT(3)
GLOBAL_UNCERTAINTY_ASSIGNED_CONTEXT((#50387))
GLOBAL_UNIT_ASSIGNED_CONTEXT((#50441,#50443,#50444))
REPRESENTATION_CONTEXT('','3D')
) ;
#50441=(
LENGTH_UNIT()
NAMED_UNIT(*)
SI_UNIT(.CENTI.,.METRE.)
) ;
#50443=(
NAMED_UNIT(*)
PLANE_ANGLE_UNIT()
SI_UNIT($,.RADIAN.)
) ;
#50444=(
NAMED_UNIT(*)
SI_UNIT($,.STERADIAN.)
SOLID_ANGLE_UNIT()
) ;
#50482=SHAPE_DEFINITION_REPRESENTATION(#50558,#50656) ;
#50558=PRODUCT_DEFINITION_SHAPE('',$,#50709) ;
#50656=SHAPE_REPRESENTATION('',(#31069),#50425) ;
#50671=PRODUCT_DEFINITION_CONTEXT('part definition',#50829,'design') ;
#50709=PRODUCT_DEFINITION('RETURN_TENSION_SPRING_ASSEMBLY',
'RETURN_TENSION_SPRING_ASSEMBLY',#50761,#50671) ;
#50761=PRODUCT_DEFINITION_FORMATION('',$,#50868) ;
#50829=APPLICATION_CONTEXT(
'Core Data for Automotive Mechanical Design Process') ;
#50830=PRODUCT_CONTEXT('part definition',#50829,'mechanical') ;
#50868=PRODUCT('RETURN_TENSION_SPRING_ASSEMBLY',
'RETURN_TENSION_SPRING_ASSEMBLY',$,(#50830)) ;
#50883=PRESENTATION_STYLE_ASSIGNMENT((#50890)) ;
#50890=SURFACE_STYLE_USAGE(.BOTH.,#50897) ;
#50897=SURFACE_SIDE_STYLE('',(#50904)) ;
#50904=SURFACE_STYLE_FILL_AREA(#50911) ;
#50911=FILL_AREA_STYLE('Steel - Satin',(#50918)) ;
#50918=FILL_AREA_STYLE_COLOUR('Steel - Satin',#50925) ;
#50925=COLOUR_RGB('Steel - Satin', 0.31764706, 0.68627451, 0.89019608) ;
ENDSEC;
END-ISO-10303-21;
